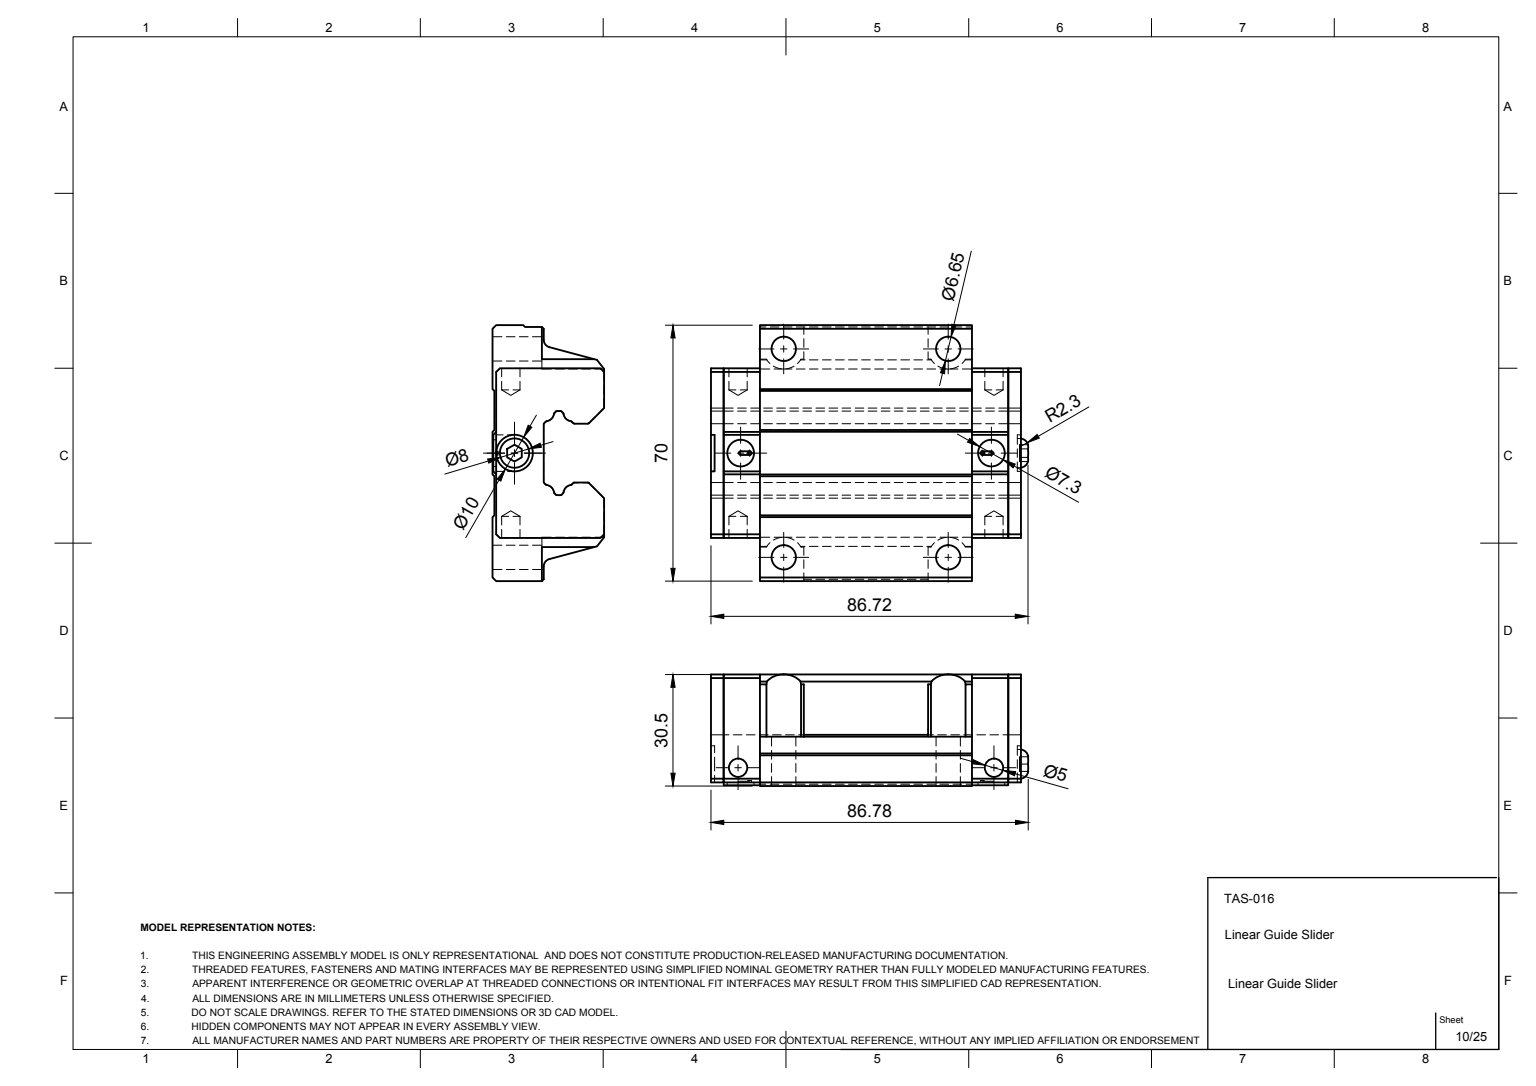
ISO-10303-21;
HEADER;
/* Generated by software containing ST-Developer
 * from STEP Tools, Inc. (www.steptools.com) 
 */

FILE_DESCRIPTION(
/* description */ ('STEP AP214'),
/* implementation_level */ '2;1');

FILE_NAME(
/* name */ 'Linear Guide Slider.step',
/* time_stamp */ '2026-11-15T14:55:55-08:00',
/* author */ (''),
/* organization */ (''),
/* preprocessor_version */ 'ST-DEVELOPER v20.2',
/* originating_system */ 'Autodesk Translation Framework v15.17.0.0',
/* authorisation */ '');

FILE_SCHEMA (('AUTOMOTIVE_DESIGN { 1 0 10303 214 3 1 1 }'));
ENDSEC;

DATA;
#10=MECHANICAL_DESIGN_GEOMETRIC_PRESENTATION_REPRESENTATION('',(#951),#57079);
#11=(
BOUNDED_CURVE()
B_SPLINE_CURVE(2,(#54195,#54196,#54197),.UNSPECIFIED.,.F.,.F.)
B_SPLINE_CURVE_WITH_KNOTS((3,3),(-1.29356557390797,0.),.UNSPECIFIED.)
CURVE()
GEOMETRIC_REPRESENTATION_ITEM()
RATIONAL_B_SPLINE_CURVE((0.954658532851732,0.77704632554749,1.))
REPRESENTATION_ITEM('')
);
#146=ELLIPSE('',#26558,6.97960018289555,5.49999999999817);
#147=ELLIPSE('',#26560,6.97960018289945,5.50000000000025);
#148=ELLIPSE('',#26561,6.97960018289465,5.49999999999756);
#149=ELLIPSE('',#26563,6.97960018289959,5.50000000000032);
#150=ELLIPSE('',#26564,6.97960018289765,5.49999999999922);
#151=ELLIPSE('',#26566,6.9796001828989,5.49999999999987);
#152=ELLIPSE('',#26887,21.2503681783598,5.50000000000001);
#153=ELLIPSE('',#26888,21.2503681783597,5.5);
#154=ELLIPSE('',#26893,21.2503681783597,5.5);
#155=ELLIPSE('',#26898,21.2503681783597,5.5);
#156=ELLIPSE('',#26900,21.2503681783597,5.49999999999999);
#157=ELLIPSE('',#26901,21.2503681783597,5.5);
#158=ELLIPSE('',#26994,21.2503681783598,5.50000000000001);
#159=ELLIPSE('',#26996,21.2503681783597,5.49999999999999);
#160=ELLIPSE('',#27001,6.97960018290351,5.50000000000224);
#161=ELLIPSE('',#27006,6.97960018290198,5.50000000000146);
#252=(
BOUNDED_SURFACE()
B_SPLINE_SURFACE(2,2,((#54133,#54134,#54135,#54136,#54137,#54138,#54139,
#54140,#54141),(#54142,#54143,#54144,#54145,#54146,#54147,#54148,#54149,
#54150),(#54151,#54152,#54153,#54154,#54155,#54156,#54157,#54158,#54159)),
 .UNSPECIFIED.,.F.,.T.,.F.)
B_SPLINE_SURFACE_WITH_KNOTS((3,3),(3,2,2,2,3),(0.,1.43998883071719),(-3.14159265358979,
-1.5707963267949,0.,1.5707963267949,3.14159265358979),.UNSPECIFIED.)
GEOMETRIC_REPRESENTATION_ITEM()
RATIONAL_B_SPLINE_SURFACE(((1.,0.707106781186548,1.,0.707106781186548,1.,
0.707106781186548,1.,0.707106781186548,1.),(0.751809411556116,0.531609533071198,
0.751809411556116,0.531609533071198,0.751809411556116,0.531609533071198,
0.751809411556116,0.531609533071198,0.751809411556116),(1.,0.707106781186548,
1.,0.707106781186548,1.,0.707106781186548,1.,0.707106781186548,1.)))
REPRESENTATION_ITEM('')
SURFACE()
);
#860=B_SPLINE_CURVE_WITH_KNOTS('',3,(#54162,#54163,#54164,#54165,#54166,
#54167,#54168,#54169,#54170,#54171),.UNSPECIFIED.,.F.,.F.,(4,2,2,2,4),(-0.991617660219933,
-0.988360888345703,-0.882558915285875,-0.776756942226048,-0.773500170351817),
 .UNSPECIFIED.);
#861=B_SPLINE_CURVE_WITH_KNOTS('',3,(#54173,#54174,#54175,#54176,#54177,
#54178,#54179,#54180,#54181,#54182),.UNSPECIFIED.,.F.,.F.,(4,2,2,2,4),(-0.991617660219933,
-0.988360888345703,-0.882558915285875,-0.776756942226048,-0.773500170351817),
 .UNSPECIFIED.);
#862=B_SPLINE_CURVE_WITH_KNOTS('',3,(#54184,#54185,#54186,#54187,#54188,
#54189,#54190,#54191,#54192,#54193),.UNSPECIFIED.,.F.,.F.,(4,2,2,2,4),(-0.991617660219934,
-0.988360888345704,-0.882558915285876,-0.776756942226048,-0.773500170351818),
 .UNSPECIFIED.);
#863=B_SPLINE_CURVE_WITH_KNOTS('',3,(#54202,#54203,#54204,#54205,#54206,
#54207,#54208,#54209,#54210,#54211),.UNSPECIFIED.,.F.,.F.,(4,2,2,2,4),(0.773500170351818,
0.776756942226048,0.882558915285876,0.988360888345703,0.991617660219934),
 .UNSPECIFIED.);
#864=B_SPLINE_CURVE_WITH_KNOTS('',3,(#54213,#54214,#54215,#54216,#54217,
#54218,#54219,#54220,#54221,#54222),.UNSPECIFIED.,.F.,.F.,(4,2,2,2,4),(0.773500170351817,
0.776756942226048,0.882558915285875,0.988360888345703,0.991617660219933),
 .UNSPECIFIED.);
#865=B_SPLINE_CURVE_WITH_KNOTS('',3,(#54223,#54224,#54225,#54226,#54227,
#54228,#54229,#54230,#54231,#54232),.UNSPECIFIED.,.F.,.F.,(4,2,2,2,4),(0.773500170351818,
0.776756942226048,0.882558915285876,0.988360888345704,0.991617660219934),
 .UNSPECIFIED.);
#889=SHAPE_REPRESENTATION_RELATIONSHIP('SRR','None',#57279,#918);
#918=ADVANCED_BREP_SHAPE_REPRESENTATION('',(#988),#57071);
#951=STYLED_ITEM('',(#57444),#988);
#988=MANIFOLD_SOLID_BREP('Body1',#24551);
#1293=FACE_BOUND('',#4751,.T.);
#1294=FACE_BOUND('',#4754,.T.);
#1295=FACE_BOUND('',#4769,.T.);
#1296=FACE_BOUND('',#4867,.T.);
#1297=FACE_BOUND('',#4880,.T.);
#1298=FACE_BOUND('',#4888,.T.);
#1299=FACE_BOUND('',#4891,.T.);
#1300=FACE_BOUND('',#4896,.T.);
#1301=FACE_BOUND('',#4944,.T.);
#1302=FACE_BOUND('',#4949,.T.);
#1303=FACE_BOUND('',#4951,.T.);
#1304=FACE_BOUND('',#4958,.T.);
#1305=FACE_BOUND('',#4959,.T.);
#1306=FACE_BOUND('',#4968,.T.);
#1307=FACE_BOUND('',#4969,.T.);
#1308=FACE_BOUND('',#4975,.T.);
#1309=FACE_BOUND('',#4981,.T.);
#1310=FACE_BOUND('',#4988,.T.);
#1311=FACE_BOUND('',#4993,.T.);
#1312=FACE_BOUND('',#5028,.T.);
#1313=FACE_BOUND('',#5040,.T.);
#1314=FACE_BOUND('',#5042,.T.);
#1788=PLANE('',#26557);
#1789=PLANE('',#26559);
#1790=PLANE('',#26562);
#1791=PLANE('',#26565);
#1792=PLANE('',#26567);
#1793=PLANE('',#26568);
#1794=PLANE('',#26569);
#1795=PLANE('',#26570);
#1796=PLANE('',#26571);
#1797=PLANE('',#26572);
#1798=PLANE('',#26573);
#1799=PLANE('',#26574);
#1800=PLANE('',#26575);
#1801=PLANE('',#26576);
#1802=PLANE('',#26577);
#1803=PLANE('',#26578);
#1804=PLANE('',#26579);
#1805=PLANE('',#26580);
#1806=PLANE('',#26581);
#1807=PLANE('',#26582);
#1808=PLANE('',#26583);
#1809=PLANE('',#26644);
#1810=PLANE('',#26645);
#1811=PLANE('',#26646);
#1812=PLANE('',#26647);
#1813=PLANE('',#26648);
#1814=PLANE('',#26649);
#1815=PLANE('',#26650);
#1816=PLANE('',#26651);
#1817=PLANE('',#26652);
#1818=PLANE('',#26653);
#1819=PLANE('',#26654);
#1820=PLANE('',#26655);
#1821=PLANE('',#26656);
#1822=PLANE('',#26657);
#1823=PLANE('',#26658);
#1824=PLANE('',#26659);
#1825=PLANE('',#26660);
#1826=PLANE('',#26681);
#1827=PLANE('',#26684);
#1828=PLANE('',#26687);
#1829=PLANE('',#26694);
#1830=PLANE('',#26697);
#1831=PLANE('',#26700);
#1832=PLANE('',#26707);
#1833=PLANE('',#26708);
#1834=PLANE('',#26709);
#1835=PLANE('',#26716);
#1836=PLANE('',#26719);
#1837=PLANE('',#26722);
#1838=PLANE('',#26729);
#1839=PLANE('',#26732);
#1840=PLANE('',#26735);
#1841=PLANE('',#26736);
#1842=PLANE('',#26737);
#1843=PLANE('',#26738);
#1844=PLANE('',#26739);
#1845=PLANE('',#26740);
#1846=PLANE('',#26741);
#1847=PLANE('',#26742);
#1848=PLANE('',#26743);
#1849=PLANE('',#26744);
#1850=PLANE('',#26745);
#1851=PLANE('',#26746);
#1852=PLANE('',#26748);
#1853=PLANE('',#26770);
#1854=PLANE('',#26771);
#1855=PLANE('',#26774);
#1856=PLANE('',#26775);
#1857=PLANE('',#26777);
#1858=PLANE('',#26778);
#1859=PLANE('',#26779);
#1860=PLANE('',#26780);
#1861=PLANE('',#26781);
#1862=PLANE('',#26782);
#1863=PLANE('',#26783);
#1864=PLANE('',#26784);
#1865=PLANE('',#26785);
#1866=PLANE('',#26786);
#1867=PLANE('',#26789);
#1868=PLANE('',#26792);
#1869=PLANE('',#26799);
#1870=PLANE('',#26802);
#1871=PLANE('',#26805);
#1872=PLANE('',#26812);
#1873=PLANE('',#26813);
#1874=PLANE('',#26814);
#1875=PLANE('',#26821);
#1876=PLANE('',#26824);
#1877=PLANE('',#26827);
#1878=PLANE('',#26834);
#1879=PLANE('',#26837);
#1880=PLANE('',#26840);
#1881=PLANE('',#26841);
#1882=PLANE('',#26842);
#1883=PLANE('',#26843);
#1884=PLANE('',#26844);
#1885=PLANE('',#26845);
#1886=PLANE('',#26851);
#1887=PLANE('',#26852);
#1888=PLANE('',#26853);
#1889=PLANE('',#26854);
#1890=PLANE('',#26858);
#1891=PLANE('',#26879);
#1892=PLANE('',#26880);
#1893=PLANE('',#26881);
#1894=PLANE('',#26882);
#1895=PLANE('',#26883);
#1896=PLANE('',#26884);
#1897=PLANE('',#26885);
#1898=PLANE('',#26886);
#1899=PLANE('',#26889);
#1900=PLANE('',#26891);
#1901=PLANE('',#26892);
#1902=PLANE('',#26894);
#1903=PLANE('',#26895);
#1904=PLANE('',#26897);
#1905=PLANE('',#26899);
#1906=PLANE('',#26902);
#1907=PLANE('',#26903);
#1908=PLANE('',#26904);
#1909=PLANE('',#26905);
#1910=PLANE('',#26906);
#1911=PLANE('',#26907);
#1912=PLANE('',#26908);
#1913=PLANE('',#26909);
#1914=PLANE('',#26910);
#1915=PLANE('',#26911);
#1916=PLANE('',#26914);
#1917=PLANE('',#26917);
#1918=PLANE('',#26924);
#1919=PLANE('',#26927);
#1920=PLANE('',#26930);
#1921=PLANE('',#26937);
#1922=PLANE('',#26938);
#1923=PLANE('',#26939);
#1924=PLANE('',#26946);
#1925=PLANE('',#26949);
#1926=PLANE('',#26952);
#1927=PLANE('',#26959);
#1928=PLANE('',#26962);
#1929=PLANE('',#26965);
#1930=PLANE('',#26966);
#1931=PLANE('',#26967);
#1932=PLANE('',#26968);
#1933=PLANE('',#26969);
#1934=PLANE('',#26970);
#1935=PLANE('',#26971);
#1936=PLANE('',#26972);
#1937=PLANE('',#26973);
#1938=PLANE('',#26974);
#1939=PLANE('',#26975);
#1940=PLANE('',#26976);
#1941=PLANE('',#26977);
#1942=PLANE('',#26978);
#1943=PLANE('',#26979);
#1944=PLANE('',#26980);
#1945=PLANE('',#26981);
#1946=PLANE('',#26982);
#1947=PLANE('',#26983);
#1948=PLANE('',#26984);
#1949=PLANE('',#26985);
#1950=PLANE('',#26986);
#1951=PLANE('',#26987);
#1952=PLANE('',#26988);
#1953=PLANE('',#26989);
#1954=PLANE('',#26990);
#1955=PLANE('',#26992);
#1956=PLANE('',#26993);
#1957=PLANE('',#26995);
#1958=PLANE('',#26997);
#1959=PLANE('',#26998);
#1960=PLANE('',#27000);
#1961=PLANE('',#27002);
#1962=PLANE('',#27003);
#1963=PLANE('',#27004);
#1964=PLANE('',#27005);
#1965=PLANE('',#27007);
#1966=PLANE('',#27028);
#1967=PLANE('',#27029);
#1968=PLANE('',#27030);
#1969=PLANE('',#27031);
#1970=PLANE('',#27032);
#1971=PLANE('',#27033);
#1972=PLANE('',#27038);
#1973=PLANE('',#27039);
#1974=PLANE('',#27040);
#1975=PLANE('',#27051);
#1976=PLANE('',#27052);
#1977=PLANE('',#27059);
#1978=PLANE('',#27060);
#1979=PLANE('',#27071);
#1980=PLANE('',#27072);
#1981=PLANE('',#27073);
#1982=PLANE('',#27084);
#1983=PLANE('',#27085);
#1984=PLANE('',#27086);
#1985=PLANE('',#27087);
#1986=PLANE('',#27088);
#1987=PLANE('',#27089);
#1988=PLANE('',#27090);
#1989=PLANE('',#27091);
#1990=PLANE('',#27092);
#1991=PLANE('',#27093);
#1992=PLANE('',#27094);
#1993=PLANE('',#27095);
#1994=PLANE('',#27096);
#1995=PLANE('',#27097);
#1996=PLANE('',#27098);
#1997=PLANE('',#27101);
#1998=PLANE('',#27102);
#2124=CONICAL_SURFACE('',#26517,2.5,1.02974425867665);
#2125=CONICAL_SURFACE('',#26518,2.5,1.02974425867665);
#2126=CONICAL_SURFACE('',#26544,2.5,1.02974425867665);
#2127=CONICAL_SURFACE('',#26545,2.5,1.02974425867665);
#3022=FACE_OUTER_BOUND('',#4690,.T.);
#3023=FACE_OUTER_BOUND('',#4691,.T.);
#3024=FACE_OUTER_BOUND('',#4692,.T.);
#3025=FACE_OUTER_BOUND('',#4693,.T.);
#3026=FACE_OUTER_BOUND('',#4694,.T.);
#3027=FACE_OUTER_BOUND('',#4695,.T.);
#3028=FACE_OUTER_BOUND('',#4696,.T.);
#3029=FACE_OUTER_BOUND('',#4697,.T.);
#3030=FACE_OUTER_BOUND('',#4698,.T.);
#3031=FACE_OUTER_BOUND('',#4699,.T.);
#3032=FACE_OUTER_BOUND('',#4700,.T.);
#3033=FACE_OUTER_BOUND('',#4701,.T.);
#3034=FACE_OUTER_BOUND('',#4702,.T.);
#3035=FACE_OUTER_BOUND('',#4703,.T.);
#3036=FACE_OUTER_BOUND('',#4704,.T.);
#3037=FACE_OUTER_BOUND('',#4705,.T.);
#3038=FACE_OUTER_BOUND('',#4706,.T.);
#3039=FACE_OUTER_BOUND('',#4707,.T.);
#3040=FACE_OUTER_BOUND('',#4708,.T.);
#3041=FACE_OUTER_BOUND('',#4709,.T.);
#3042=FACE_OUTER_BOUND('',#4710,.T.);
#3043=FACE_OUTER_BOUND('',#4711,.T.);
#3044=FACE_OUTER_BOUND('',#4712,.T.);
#3045=FACE_OUTER_BOUND('',#4713,.T.);
#3046=FACE_OUTER_BOUND('',#4714,.T.);
#3047=FACE_OUTER_BOUND('',#4715,.T.);
#3048=FACE_OUTER_BOUND('',#4716,.T.);
#3049=FACE_OUTER_BOUND('',#4717,.T.);
#3050=FACE_OUTER_BOUND('',#4718,.T.);
#3051=FACE_OUTER_BOUND('',#4719,.T.);
#3052=FACE_OUTER_BOUND('',#4720,.T.);
#3053=FACE_OUTER_BOUND('',#4721,.T.);
#3054=FACE_OUTER_BOUND('',#4722,.T.);
#3055=FACE_OUTER_BOUND('',#4723,.T.);
#3056=FACE_OUTER_BOUND('',#4724,.T.);
#3057=FACE_OUTER_BOUND('',#4725,.T.);
#3058=FACE_OUTER_BOUND('',#4726,.T.);
#3059=FACE_OUTER_BOUND('',#4727,.T.);
#3060=FACE_OUTER_BOUND('',#4728,.T.);
#3061=FACE_OUTER_BOUND('',#4729,.T.);
#3062=FACE_OUTER_BOUND('',#4730,.T.);
#3063=FACE_OUTER_BOUND('',#4731,.T.);
#3064=FACE_OUTER_BOUND('',#4732,.T.);
#3065=FACE_OUTER_BOUND('',#4733,.T.);
#3066=FACE_OUTER_BOUND('',#4734,.T.);
#3067=FACE_OUTER_BOUND('',#4735,.T.);
#3068=FACE_OUTER_BOUND('',#4736,.T.);
#3069=FACE_OUTER_BOUND('',#4737,.T.);
#3070=FACE_OUTER_BOUND('',#4738,.T.);
#3071=FACE_OUTER_BOUND('',#4739,.T.);
#3072=FACE_OUTER_BOUND('',#4740,.T.);
#3073=FACE_OUTER_BOUND('',#4741,.T.);
#3074=FACE_OUTER_BOUND('',#4742,.T.);
#3075=FACE_OUTER_BOUND('',#4743,.T.);
#3076=FACE_OUTER_BOUND('',#4744,.T.);
#3077=FACE_OUTER_BOUND('',#4745,.T.);
#3078=FACE_OUTER_BOUND('',#4746,.T.);
#3079=FACE_OUTER_BOUND('',#4747,.T.);
#3080=FACE_OUTER_BOUND('',#4748,.T.);
#3081=FACE_OUTER_BOUND('',#4749,.T.);
#3082=FACE_OUTER_BOUND('',#4750,.T.);
#3083=FACE_OUTER_BOUND('',#4752,.T.);
#3084=FACE_OUTER_BOUND('',#4753,.T.);
#3085=FACE_OUTER_BOUND('',#4755,.T.);
#3086=FACE_OUTER_BOUND('',#4756,.T.);
#3087=FACE_OUTER_BOUND('',#4757,.T.);
#3088=FACE_OUTER_BOUND('',#4758,.T.);
#3089=FACE_OUTER_BOUND('',#4759,.T.);
#3090=FACE_OUTER_BOUND('',#4760,.T.);
#3091=FACE_OUTER_BOUND('',#4761,.T.);
#3092=FACE_OUTER_BOUND('',#4762,.T.);
#3093=FACE_OUTER_BOUND('',#4763,.T.);
#3094=FACE_OUTER_BOUND('',#4764,.T.);
#3095=FACE_OUTER_BOUND('',#4765,.T.);
#3096=FACE_OUTER_BOUND('',#4766,.T.);
#3097=FACE_OUTER_BOUND('',#4767,.T.);
#3098=FACE_OUTER_BOUND('',#4768,.T.);
#3099=FACE_OUTER_BOUND('',#4770,.T.);
#3100=FACE_OUTER_BOUND('',#4771,.T.);
#3101=FACE_OUTER_BOUND('',#4772,.T.);
#3102=FACE_OUTER_BOUND('',#4773,.T.);
#3103=FACE_OUTER_BOUND('',#4774,.T.);
#3104=FACE_OUTER_BOUND('',#4775,.T.);
#3105=FACE_OUTER_BOUND('',#4776,.T.);
#3106=FACE_OUTER_BOUND('',#4777,.T.);
#3107=FACE_OUTER_BOUND('',#4778,.T.);
#3108=FACE_OUTER_BOUND('',#4779,.T.);
#3109=FACE_OUTER_BOUND('',#4780,.T.);
#3110=FACE_OUTER_BOUND('',#4781,.T.);
#3111=FACE_OUTER_BOUND('',#4782,.T.);
#3112=FACE_OUTER_BOUND('',#4783,.T.);
#3113=FACE_OUTER_BOUND('',#4784,.T.);
#3114=FACE_OUTER_BOUND('',#4785,.T.);
#3115=FACE_OUTER_BOUND('',#4786,.T.);
#3116=FACE_OUTER_BOUND('',#4787,.T.);
#3117=FACE_OUTER_BOUND('',#4788,.T.);
#3118=FACE_OUTER_BOUND('',#4789,.T.);
#3119=FACE_OUTER_BOUND('',#4790,.T.);
#3120=FACE_OUTER_BOUND('',#4791,.T.);
#3121=FACE_OUTER_BOUND('',#4792,.T.);
#3122=FACE_OUTER_BOUND('',#4793,.T.);
#3123=FACE_OUTER_BOUND('',#4794,.T.);
#3124=FACE_OUTER_BOUND('',#4795,.T.);
#3125=FACE_OUTER_BOUND('',#4796,.T.);
#3126=FACE_OUTER_BOUND('',#4797,.T.);
#3127=FACE_OUTER_BOUND('',#4798,.T.);
#3128=FACE_OUTER_BOUND('',#4799,.T.);
#3129=FACE_OUTER_BOUND('',#4800,.T.);
#3130=FACE_OUTER_BOUND('',#4801,.T.);
#3131=FACE_OUTER_BOUND('',#4802,.T.);
#3132=FACE_OUTER_BOUND('',#4803,.T.);
#3133=FACE_OUTER_BOUND('',#4804,.T.);
#3134=FACE_OUTER_BOUND('',#4805,.T.);
#3135=FACE_OUTER_BOUND('',#4806,.T.);
#3136=FACE_OUTER_BOUND('',#4807,.T.);
#3137=FACE_OUTER_BOUND('',#4808,.T.);
#3138=FACE_OUTER_BOUND('',#4809,.T.);
#3139=FACE_OUTER_BOUND('',#4810,.T.);
#3140=FACE_OUTER_BOUND('',#4811,.T.);
#3141=FACE_OUTER_BOUND('',#4812,.T.);
#3142=FACE_OUTER_BOUND('',#4813,.T.);
#3143=FACE_OUTER_BOUND('',#4814,.T.);
#3144=FACE_OUTER_BOUND('',#4815,.T.);
#3145=FACE_OUTER_BOUND('',#4816,.T.);
#3146=FACE_OUTER_BOUND('',#4817,.T.);
#3147=FACE_OUTER_BOUND('',#4818,.T.);
#3148=FACE_OUTER_BOUND('',#4819,.T.);
#3149=FACE_OUTER_BOUND('',#4820,.T.);
#3150=FACE_OUTER_BOUND('',#4821,.T.);
#3151=FACE_OUTER_BOUND('',#4822,.T.);
#3152=FACE_OUTER_BOUND('',#4823,.T.);
#3153=FACE_OUTER_BOUND('',#4824,.T.);
#3154=FACE_OUTER_BOUND('',#4825,.T.);
#3155=FACE_OUTER_BOUND('',#4826,.T.);
#3156=FACE_OUTER_BOUND('',#4827,.T.);
#3157=FACE_OUTER_BOUND('',#4828,.T.);
#3158=FACE_OUTER_BOUND('',#4829,.T.);
#3159=FACE_OUTER_BOUND('',#4830,.T.);
#3160=FACE_OUTER_BOUND('',#4831,.T.);
#3161=FACE_OUTER_BOUND('',#4832,.T.);
#3162=FACE_OUTER_BOUND('',#4833,.T.);
#3163=FACE_OUTER_BOUND('',#4834,.T.);
#3164=FACE_OUTER_BOUND('',#4835,.T.);
#3165=FACE_OUTER_BOUND('',#4836,.T.);
#3166=FACE_OUTER_BOUND('',#4837,.T.);
#3167=FACE_OUTER_BOUND('',#4838,.T.);
#3168=FACE_OUTER_BOUND('',#4839,.T.);
#3169=FACE_OUTER_BOUND('',#4840,.T.);
#3170=FACE_OUTER_BOUND('',#4841,.T.);
#3171=FACE_OUTER_BOUND('',#4842,.T.);
#3172=FACE_OUTER_BOUND('',#4843,.T.);
#3173=FACE_OUTER_BOUND('',#4844,.T.);
#3174=FACE_OUTER_BOUND('',#4845,.T.);
#3175=FACE_OUTER_BOUND('',#4846,.T.);
#3176=FACE_OUTER_BOUND('',#4847,.T.);
#3177=FACE_OUTER_BOUND('',#4848,.T.);
#3178=FACE_OUTER_BOUND('',#4849,.T.);
#3179=FACE_OUTER_BOUND('',#4850,.T.);
#3180=FACE_OUTER_BOUND('',#4851,.T.);
#3181=FACE_OUTER_BOUND('',#4852,.T.);
#3182=FACE_OUTER_BOUND('',#4853,.T.);
#3183=FACE_OUTER_BOUND('',#4854,.T.);
#3184=FACE_OUTER_BOUND('',#4855,.T.);
#3185=FACE_OUTER_BOUND('',#4856,.T.);
#3186=FACE_OUTER_BOUND('',#4857,.T.);
#3187=FACE_OUTER_BOUND('',#4858,.T.);
#3188=FACE_OUTER_BOUND('',#4859,.T.);
#3189=FACE_OUTER_BOUND('',#4860,.T.);
#3190=FACE_OUTER_BOUND('',#4861,.T.);
#3191=FACE_OUTER_BOUND('',#4862,.T.);
#3192=FACE_OUTER_BOUND('',#4863,.T.);
#3193=FACE_OUTER_BOUND('',#4864,.T.);
#3194=FACE_OUTER_BOUND('',#4865,.T.);
#3195=FACE_OUTER_BOUND('',#4866,.T.);
#3196=FACE_OUTER_BOUND('',#4868,.T.);
#3197=FACE_OUTER_BOUND('',#4869,.T.);
#3198=FACE_OUTER_BOUND('',#4870,.T.);
#3199=FACE_OUTER_BOUND('',#4871,.T.);
#3200=FACE_OUTER_BOUND('',#4872,.T.);
#3201=FACE_OUTER_BOUND('',#4873,.T.);
#3202=FACE_OUTER_BOUND('',#4874,.T.);
#3203=FACE_OUTER_BOUND('',#4875,.T.);
#3204=FACE_OUTER_BOUND('',#4876,.T.);
#3205=FACE_OUTER_BOUND('',#4877,.T.);
#3206=FACE_OUTER_BOUND('',#4878,.T.);
#3207=FACE_OUTER_BOUND('',#4879,.T.);
#3208=FACE_OUTER_BOUND('',#4881,.T.);
#3209=FACE_OUTER_BOUND('',#4882,.T.);
#3210=FACE_OUTER_BOUND('',#4883,.T.);
#3211=FACE_OUTER_BOUND('',#4884,.T.);
#3212=FACE_OUTER_BOUND('',#4885,.T.);
#3213=FACE_OUTER_BOUND('',#4886,.T.);
#3214=FACE_OUTER_BOUND('',#4887,.T.);
#3215=FACE_OUTER_BOUND('',#4889,.T.);
#3216=FACE_OUTER_BOUND('',#4890,.T.);
#3217=FACE_OUTER_BOUND('',#4892,.T.);
#3218=FACE_OUTER_BOUND('',#4893,.T.);
#3219=FACE_OUTER_BOUND('',#4894,.T.);
#3220=FACE_OUTER_BOUND('',#4895,.T.);
#3221=FACE_OUTER_BOUND('',#4897,.T.);
#3222=FACE_OUTER_BOUND('',#4898,.T.);
#3223=FACE_OUTER_BOUND('',#4899,.T.);
#3224=FACE_OUTER_BOUND('',#4900,.T.);
#3225=FACE_OUTER_BOUND('',#4901,.T.);
#3226=FACE_OUTER_BOUND('',#4902,.T.);
#3227=FACE_OUTER_BOUND('',#4903,.T.);
#3228=FACE_OUTER_BOUND('',#4904,.T.);
#3229=FACE_OUTER_BOUND('',#4905,.T.);
#3230=FACE_OUTER_BOUND('',#4906,.T.);
#3231=FACE_OUTER_BOUND('',#4907,.T.);
#3232=FACE_OUTER_BOUND('',#4908,.T.);
#3233=FACE_OUTER_BOUND('',#4909,.T.);
#3234=FACE_OUTER_BOUND('',#4910,.T.);
#3235=FACE_OUTER_BOUND('',#4911,.T.);
#3236=FACE_OUTER_BOUND('',#4912,.T.);
#3237=FACE_OUTER_BOUND('',#4913,.T.);
#3238=FACE_OUTER_BOUND('',#4914,.T.);
#3239=FACE_OUTER_BOUND('',#4915,.T.);
#3240=FACE_OUTER_BOUND('',#4916,.T.);
#3241=FACE_OUTER_BOUND('',#4917,.T.);
#3242=FACE_OUTER_BOUND('',#4918,.T.);
#3243=FACE_OUTER_BOUND('',#4919,.T.);
#3244=FACE_OUTER_BOUND('',#4920,.T.);
#3245=FACE_OUTER_BOUND('',#4921,.T.);
#3246=FACE_OUTER_BOUND('',#4922,.T.);
#3247=FACE_OUTER_BOUND('',#4923,.T.);
#3248=FACE_OUTER_BOUND('',#4924,.T.);
#3249=FACE_OUTER_BOUND('',#4925,.T.);
#3250=FACE_OUTER_BOUND('',#4926,.T.);
#3251=FACE_OUTER_BOUND('',#4927,.T.);
#3252=FACE_OUTER_BOUND('',#4928,.T.);
#3253=FACE_OUTER_BOUND('',#4929,.T.);
#3254=FACE_OUTER_BOUND('',#4930,.T.);
#3255=FACE_OUTER_BOUND('',#4931,.T.);
#3256=FACE_OUTER_BOUND('',#4932,.T.);
#3257=FACE_OUTER_BOUND('',#4933,.T.);
#3258=FACE_OUTER_BOUND('',#4934,.T.);
#3259=FACE_OUTER_BOUND('',#4935,.T.);
#3260=FACE_OUTER_BOUND('',#4936,.T.);
#3261=FACE_OUTER_BOUND('',#4937,.T.);
#3262=FACE_OUTER_BOUND('',#4938,.T.);
#3263=FACE_OUTER_BOUND('',#4939,.T.);
#3264=FACE_OUTER_BOUND('',#4940,.T.);
#3265=FACE_OUTER_BOUND('',#4941,.T.);
#3266=FACE_OUTER_BOUND('',#4942,.T.);
#3267=FACE_OUTER_BOUND('',#4943,.T.);
#3268=FACE_OUTER_BOUND('',#4945,.T.);
#3269=FACE_OUTER_BOUND('',#4946,.T.);
#3270=FACE_OUTER_BOUND('',#4947,.T.);
#3271=FACE_OUTER_BOUND('',#4948,.T.);
#3272=FACE_OUTER_BOUND('',#4950,.T.);
#3273=FACE_OUTER_BOUND('',#4952,.T.);
#3274=FACE_OUTER_BOUND('',#4953,.T.);
#3275=FACE_OUTER_BOUND('',#4954,.T.);
#3276=FACE_OUTER_BOUND('',#4955,.T.);
#3277=FACE_OUTER_BOUND('',#4956,.T.);
#3278=FACE_OUTER_BOUND('',#4957,.T.);
#3279=FACE_OUTER_BOUND('',#4960,.T.);
#3280=FACE_OUTER_BOUND('',#4961,.T.);
#3281=FACE_OUTER_BOUND('',#4962,.T.);
#3282=FACE_OUTER_BOUND('',#4963,.T.);
#3283=FACE_OUTER_BOUND('',#4964,.T.);
#3284=FACE_OUTER_BOUND('',#4965,.T.);
#3285=FACE_OUTER_BOUND('',#4966,.T.);
#3286=FACE_OUTER_BOUND('',#4967,.T.);
#3287=FACE_OUTER_BOUND('',#4970,.T.);
#3288=FACE_OUTER_BOUND('',#4971,.T.);
#3289=FACE_OUTER_BOUND('',#4972,.T.);
#3290=FACE_OUTER_BOUND('',#4973,.T.);
#3291=FACE_OUTER_BOUND('',#4974,.T.);
#3292=FACE_OUTER_BOUND('',#4976,.T.);
#3293=FACE_OUTER_BOUND('',#4977,.T.);
#3294=FACE_OUTER_BOUND('',#4978,.T.);
#3295=FACE_OUTER_BOUND('',#4979,.T.);
#3296=FACE_OUTER_BOUND('',#4980,.T.);
#3297=FACE_OUTER_BOUND('',#4982,.T.);
#3298=FACE_OUTER_BOUND('',#4983,.T.);
#3299=FACE_OUTER_BOUND('',#4984,.T.);
#3300=FACE_OUTER_BOUND('',#4985,.T.);
#3301=FACE_OUTER_BOUND('',#4986,.T.);
#3302=FACE_OUTER_BOUND('',#4987,.T.);
#3303=FACE_OUTER_BOUND('',#4989,.T.);
#3304=FACE_OUTER_BOUND('',#4990,.T.);
#3305=FACE_OUTER_BOUND('',#4991,.T.);
#3306=FACE_OUTER_BOUND('',#4992,.T.);
#3307=FACE_OUTER_BOUND('',#4994,.T.);
#3308=FACE_OUTER_BOUND('',#4995,.T.);
#3309=FACE_OUTER_BOUND('',#4996,.T.);
#3310=FACE_OUTER_BOUND('',#4997,.T.);
#3311=FACE_OUTER_BOUND('',#4998,.T.);
#3312=FACE_OUTER_BOUND('',#4999,.T.);
#3313=FACE_OUTER_BOUND('',#5000,.T.);
#3314=FACE_OUTER_BOUND('',#5001,.T.);
#3315=FACE_OUTER_BOUND('',#5002,.T.);
#3316=FACE_OUTER_BOUND('',#5003,.T.);
#3317=FACE_OUTER_BOUND('',#5004,.T.);
#3318=FACE_OUTER_BOUND('',#5005,.T.);
#3319=FACE_OUTER_BOUND('',#5006,.T.);
#3320=FACE_OUTER_BOUND('',#5007,.T.);
#3321=FACE_OUTER_BOUND('',#5008,.T.);
#3322=FACE_OUTER_BOUND('',#5009,.T.);
#3323=FACE_OUTER_BOUND('',#5010,.T.);
#3324=FACE_OUTER_BOUND('',#5011,.T.);
#3325=FACE_OUTER_BOUND('',#5012,.T.);
#3326=FACE_OUTER_BOUND('',#5013,.T.);
#3327=FACE_OUTER_BOUND('',#5014,.T.);
#3328=FACE_OUTER_BOUND('',#5015,.T.);
#3329=FACE_OUTER_BOUND('',#5016,.T.);
#3330=FACE_OUTER_BOUND('',#5017,.T.);
#3331=FACE_OUTER_BOUND('',#5018,.T.);
#3332=FACE_OUTER_BOUND('',#5019,.T.);
#3333=FACE_OUTER_BOUND('',#5020,.T.);
#3334=FACE_OUTER_BOUND('',#5021,.T.);
#3335=FACE_OUTER_BOUND('',#5022,.T.);
#3336=FACE_OUTER_BOUND('',#5023,.T.);
#3337=FACE_OUTER_BOUND('',#5024,.T.);
#3338=FACE_OUTER_BOUND('',#5025,.T.);
#3339=FACE_OUTER_BOUND('',#5026,.T.);
#3340=FACE_OUTER_BOUND('',#5027,.T.);
#3341=FACE_OUTER_BOUND('',#5029,.T.);
#3342=FACE_OUTER_BOUND('',#5030,.T.);
#3343=FACE_OUTER_BOUND('',#5031,.T.);
#3344=FACE_OUTER_BOUND('',#5032,.T.);
#3345=FACE_OUTER_BOUND('',#5033,.T.);
#3346=FACE_OUTER_BOUND('',#5034,.T.);
#3347=FACE_OUTER_BOUND('',#5035,.T.);
#3348=FACE_OUTER_BOUND('',#5036,.T.);
#3349=FACE_OUTER_BOUND('',#5037,.T.);
#3350=FACE_OUTER_BOUND('',#5038,.T.);
#3351=FACE_OUTER_BOUND('',#5039,.T.);
#3352=FACE_OUTER_BOUND('',#5041,.T.);
#3353=FACE_OUTER_BOUND('',#5043,.T.);
#3354=FACE_OUTER_BOUND('',#5044,.T.);
#3355=FACE_OUTER_BOUND('',#5045,.T.);
#3356=FACE_OUTER_BOUND('',#5046,.T.);
#3357=FACE_OUTER_BOUND('',#5047,.T.);
#3358=FACE_OUTER_BOUND('',#5048,.T.);
#3359=FACE_OUTER_BOUND('',#5049,.T.);
#3360=FACE_OUTER_BOUND('',#5050,.T.);
#4690=EDGE_LOOP('',(#20092,#20093,#20094,#20095));
#4691=EDGE_LOOP('',(#20096,#20097,#20098,#20099));
#4692=EDGE_LOOP('',(#20100,#20101,#20102,#20103));
#4693=EDGE_LOOP('',(#20104,#20105,#20106));
#4694=EDGE_LOOP('',(#20107,#20108,#20109));
#4695=EDGE_LOOP('',(#20110,#20111,#20112,#20113));
#4696=EDGE_LOOP('',(#20114,#20115,#20116,#20117));
#4697=EDGE_LOOP('',(#20118,#20119,#20120,#20121));
#4698=EDGE_LOOP('',(#20122,#20123,#20124,#20125));
#4699=EDGE_LOOP('',(#20126,#20127,#20128,#20129));
#4700=EDGE_LOOP('',(#20130,#20131,#20132,#20133));
#4701=EDGE_LOOP('',(#20134,#20135,#20136,#20137));
#4702=EDGE_LOOP('',(#20138,#20139,#20140,#20141,#20142,#20143,#20144));
#4703=EDGE_LOOP('',(#20145,#20146,#20147));
#4704=EDGE_LOOP('',(#20148,#20149,#20150));
#4705=EDGE_LOOP('',(#20151,#20152,#20153,#20154,#20155,#20156,#20157));
#4706=EDGE_LOOP('',(#20158,#20159,#20160,#20161,#20162,#20163,#20164,#20165,
#20166,#20167));
#4707=EDGE_LOOP('',(#20168,#20169,#20170,#20171,#20172));
#4708=EDGE_LOOP('',(#20173,#20174,#20175,#20176));
#4709=EDGE_LOOP('',(#20177,#20178,#20179,#20180));
#4710=EDGE_LOOP('',(#20181,#20182,#20183,#20184));
#4711=EDGE_LOOP('',(#20185,#20186,#20187,#20188));
#4712=EDGE_LOOP('',(#20189,#20190,#20191,#20192));
#4713=EDGE_LOOP('',(#20193,#20194,#20195,#20196));
#4714=EDGE_LOOP('',(#20197,#20198,#20199,#20200));
#4715=EDGE_LOOP('',(#20201,#20202,#20203,#20204));
#4716=EDGE_LOOP('',(#20205,#20206,#20207,#20208));
#4717=EDGE_LOOP('',(#20209,#20210,#20211,#20212));
#4718=EDGE_LOOP('',(#20213,#20214,#20215,#20216));
#4719=EDGE_LOOP('',(#20217,#20218,#20219,#20220));
#4720=EDGE_LOOP('',(#20221,#20222,#20223,#20224));
#4721=EDGE_LOOP('',(#20225,#20226,#20227,#20228));
#4722=EDGE_LOOP('',(#20229,#20230,#20231,#20232));
#4723=EDGE_LOOP('',(#20233,#20234,#20235,#20236));
#4724=EDGE_LOOP('',(#20237,#20238,#20239,#20240));
#4725=EDGE_LOOP('',(#20241,#20242,#20243,#20244));
#4726=EDGE_LOOP('',(#20245,#20246,#20247,#20248));
#4727=EDGE_LOOP('',(#20249,#20250,#20251,#20252));
#4728=EDGE_LOOP('',(#20253,#20254,#20255,#20256));
#4729=EDGE_LOOP('',(#20257,#20258,#20259,#20260));
#4730=EDGE_LOOP('',(#20261,#20262,#20263,#20264));
#4731=EDGE_LOOP('',(#20265,#20266,#20267,#20268));
#4732=EDGE_LOOP('',(#20269,#20270,#20271,#20272));
#4733=EDGE_LOOP('',(#20273,#20274,#20275,#20276));
#4734=EDGE_LOOP('',(#20277,#20278,#20279,#20280));
#4735=EDGE_LOOP('',(#20281,#20282,#20283,#20284));
#4736=EDGE_LOOP('',(#20285,#20286,#20287,#20288));
#4737=EDGE_LOOP('',(#20289,#20290,#20291,#20292));
#4738=EDGE_LOOP('',(#20293,#20294,#20295,#20296));
#4739=EDGE_LOOP('',(#20297,#20298,#20299,#20300));
#4740=EDGE_LOOP('',(#20301,#20302,#20303,#20304));
#4741=EDGE_LOOP('',(#20305,#20306,#20307,#20308));
#4742=EDGE_LOOP('',(#20309,#20310,#20311,#20312));
#4743=EDGE_LOOP('',(#20313,#20314,#20315,#20316));
#4744=EDGE_LOOP('',(#20317,#20318,#20319,#20320));
#4745=EDGE_LOOP('',(#20321,#20322,#20323,#20324));
#4746=EDGE_LOOP('',(#20325,#20326,#20327,#20328));
#4747=EDGE_LOOP('',(#20329,#20330,#20331,#20332));
#4748=EDGE_LOOP('',(#20333,#20334,#20335,#20336));
#4749=EDGE_LOOP('',(#20337,#20338,#20339,#20340));
#4750=EDGE_LOOP('',(#20341));
#4751=EDGE_LOOP('',(#20342));
#4752=EDGE_LOOP('',(#20343,#20344,#20345,#20346));
#4753=EDGE_LOOP('',(#20347,#20348,#20349,#20350,#20351,#20352,#20353,#20354,
#20355,#20356,#20357,#20358,#20359,#20360,#20361,#20362,#20363,#20364,#20365,
#20366,#20367,#20368,#20369,#20370,#20371,#20372,#20373,#20374,#20375,#20376,
#20377,#20378,#20379,#20380,#20381,#20382,#20383,#20384,#20385,#20386,#20387,
#20388,#20389,#20390));
#4754=EDGE_LOOP('',(#20391));
#4755=EDGE_LOOP('',(#20392,#20393,#20394,#20395));
#4756=EDGE_LOOP('',(#20396,#20397,#20398,#20399));
#4757=EDGE_LOOP('',(#20400,#20401,#20402,#20403));
#4758=EDGE_LOOP('',(#20404,#20405,#20406,#20407));
#4759=EDGE_LOOP('',(#20408,#20409,#20410,#20411));
#4760=EDGE_LOOP('',(#20412,#20413,#20414,#20415));
#4761=EDGE_LOOP('',(#20416,#20417,#20418,#20419));
#4762=EDGE_LOOP('',(#20420,#20421,#20422,#20423));
#4763=EDGE_LOOP('',(#20424,#20425,#20426,#20427));
#4764=EDGE_LOOP('',(#20428,#20429,#20430,#20431));
#4765=EDGE_LOOP('',(#20432,#20433,#20434,#20435));
#4766=EDGE_LOOP('',(#20436,#20437,#20438,#20439));
#4767=EDGE_LOOP('',(#20440,#20441,#20442,#20443,#20444,#20445));
#4768=EDGE_LOOP('',(#20446,#20447,#20448,#20449,#20450,#20451,#20452,#20453,
#20454,#20455,#20456,#20457,#20458,#20459,#20460,#20461,#20462,#20463,#20464,
#20465,#20466,#20467,#20468,#20469,#20470,#20471,#20472,#20473,#20474,#20475,
#20476,#20477,#20478,#20479,#20480,#20481,#20482,#20483,#20484,#20485,#20486,
#20487,#20488,#20489));
#4769=EDGE_LOOP('',(#20490,#20491,#20492,#20493,#20494,#20495,#20496,#20497,
#20498,#20499,#20500,#20501,#20502,#20503,#20504,#20505,#20506,#20507,#20508,
#20509,#20510,#20511,#20512,#20513,#20514,#20515,#20516,#20517,#20518,#20519,
#20520,#20521,#20522,#20523,#20524,#20525,#20526,#20527,#20528,#20529,#20530,
#20531,#20532,#20533));
#4770=EDGE_LOOP('',(#20534,#20535,#20536,#20537));
#4771=EDGE_LOOP('',(#20538,#20539,#20540,#20541));
#4772=EDGE_LOOP('',(#20542,#20543,#20544,#20545));
#4773=EDGE_LOOP('',(#20546,#20547,#20548,#20549));
#4774=EDGE_LOOP('',(#20550,#20551,#20552,#20553));
#4775=EDGE_LOOP('',(#20554,#20555,#20556,#20557));
#4776=EDGE_LOOP('',(#20558,#20559,#20560,#20561));
#4777=EDGE_LOOP('',(#20562,#20563,#20564,#20565));
#4778=EDGE_LOOP('',(#20566,#20567,#20568,#20569));
#4779=EDGE_LOOP('',(#20570,#20571,#20572,#20573));
#4780=EDGE_LOOP('',(#20574,#20575,#20576,#20577));
#4781=EDGE_LOOP('',(#20578,#20579,#20580,#20581));
#4782=EDGE_LOOP('',(#20582,#20583,#20584,#20585));
#4783=EDGE_LOOP('',(#20586,#20587,#20588,#20589));
#4784=EDGE_LOOP('',(#20590,#20591,#20592,#20593));
#4785=EDGE_LOOP('',(#20594,#20595,#20596,#20597));
#4786=EDGE_LOOP('',(#20598,#20599,#20600,#20601));
#4787=EDGE_LOOP('',(#20602,#20603,#20604,#20605));
#4788=EDGE_LOOP('',(#20606,#20607,#20608,#20609));
#4789=EDGE_LOOP('',(#20610,#20611,#20612,#20613));
#4790=EDGE_LOOP('',(#20614,#20615,#20616,#20617));
#4791=EDGE_LOOP('',(#20618,#20619,#20620,#20621));
#4792=EDGE_LOOP('',(#20622,#20623,#20624,#20625));
#4793=EDGE_LOOP('',(#20626,#20627,#20628,#20629));
#4794=EDGE_LOOP('',(#20630,#20631,#20632,#20633));
#4795=EDGE_LOOP('',(#20634,#20635,#20636,#20637));
#4796=EDGE_LOOP('',(#20638,#20639,#20640,#20641));
#4797=EDGE_LOOP('',(#20642,#20643,#20644,#20645));
#4798=EDGE_LOOP('',(#20646,#20647,#20648,#20649));
#4799=EDGE_LOOP('',(#20650,#20651,#20652,#20653));
#4800=EDGE_LOOP('',(#20654,#20655,#20656,#20657));
#4801=EDGE_LOOP('',(#20658,#20659,#20660,#20661));
#4802=EDGE_LOOP('',(#20662,#20663,#20664,#20665));
#4803=EDGE_LOOP('',(#20666,#20667,#20668,#20669));
#4804=EDGE_LOOP('',(#20670,#20671,#20672,#20673));
#4805=EDGE_LOOP('',(#20674,#20675,#20676,#20677));
#4806=EDGE_LOOP('',(#20678,#20679,#20680,#20681));
#4807=EDGE_LOOP('',(#20682,#20683,#20684,#20685));
#4808=EDGE_LOOP('',(#20686,#20687,#20688,#20689));
#4809=EDGE_LOOP('',(#20690,#20691,#20692,#20693));
#4810=EDGE_LOOP('',(#20694,#20695,#20696,#20697));
#4811=EDGE_LOOP('',(#20698,#20699,#20700,#20701));
#4812=EDGE_LOOP('',(#20702,#20703,#20704,#20705));
#4813=EDGE_LOOP('',(#20706,#20707,#20708,#20709));
#4814=EDGE_LOOP('',(#20710));
#4815=EDGE_LOOP('',(#20711,#20712,#20713,#20714));
#4816=EDGE_LOOP('',(#20715,#20716,#20717,#20718,#20719,#20720,#20721,#20722,
#20723,#20724,#20725,#20726,#20727,#20728,#20729,#20730,#20731,#20732,#20733,
#20734,#20735,#20736,#20737,#20738,#20739,#20740,#20741,#20742,#20743,#20744,
#20745,#20746,#20747,#20748,#20749,#20750,#20751,#20752,#20753,#20754,#20755,
#20756,#20757,#20758,#20759,#20760,#20761,#20762));
#4817=EDGE_LOOP('',(#20763,#20764,#20765,#20766));
#4818=EDGE_LOOP('',(#20767,#20768,#20769,#20770));
#4819=EDGE_LOOP('',(#20771,#20772,#20773,#20774));
#4820=EDGE_LOOP('',(#20775));
#4821=EDGE_LOOP('',(#20776,#20777,#20778,#20779));
#4822=EDGE_LOOP('',(#20780,#20781,#20782,#20783));
#4823=EDGE_LOOP('',(#20784,#20785,#20786,#20787));
#4824=EDGE_LOOP('',(#20788,#20789,#20790,#20791));
#4825=EDGE_LOOP('',(#20792,#20793,#20794,#20795));
#4826=EDGE_LOOP('',(#20796,#20797,#20798,#20799,#20800,#20801,#20802,#20803));
#4827=EDGE_LOOP('',(#20804,#20805,#20806,#20807));
#4828=EDGE_LOOP('',(#20808,#20809,#20810,#20811));
#4829=EDGE_LOOP('',(#20812,#20813,#20814,#20815));
#4830=EDGE_LOOP('',(#20816,#20817,#20818,#20819));
#4831=EDGE_LOOP('',(#20820,#20821,#20822,#20823));
#4832=EDGE_LOOP('',(#20824,#20825,#20826,#20827));
#4833=EDGE_LOOP('',(#20828,#20829,#20830,#20831));
#4834=EDGE_LOOP('',(#20832,#20833,#20834,#20835));
#4835=EDGE_LOOP('',(#20836,#20837,#20838,#20839));
#4836=EDGE_LOOP('',(#20840,#20841,#20842,#20843));
#4837=EDGE_LOOP('',(#20844,#20845,#20846,#20847));
#4838=EDGE_LOOP('',(#20848,#20849,#20850,#20851));
#4839=EDGE_LOOP('',(#20852,#20853,#20854,#20855));
#4840=EDGE_LOOP('',(#20856,#20857,#20858,#20859));
#4841=EDGE_LOOP('',(#20860,#20861,#20862,#20863));
#4842=EDGE_LOOP('',(#20864,#20865,#20866,#20867));
#4843=EDGE_LOOP('',(#20868,#20869,#20870,#20871));
#4844=EDGE_LOOP('',(#20872,#20873,#20874,#20875));
#4845=EDGE_LOOP('',(#20876,#20877,#20878,#20879));
#4846=EDGE_LOOP('',(#20880,#20881,#20882,#20883));
#4847=EDGE_LOOP('',(#20884,#20885,#20886,#20887));
#4848=EDGE_LOOP('',(#20888,#20889,#20890,#20891));
#4849=EDGE_LOOP('',(#20892,#20893,#20894,#20895));
#4850=EDGE_LOOP('',(#20896,#20897,#20898,#20899));
#4851=EDGE_LOOP('',(#20900,#20901,#20902,#20903));
#4852=EDGE_LOOP('',(#20904,#20905,#20906,#20907));
#4853=EDGE_LOOP('',(#20908,#20909,#20910,#20911));
#4854=EDGE_LOOP('',(#20912,#20913,#20914,#20915));
#4855=EDGE_LOOP('',(#20916,#20917,#20918,#20919));
#4856=EDGE_LOOP('',(#20920,#20921,#20922,#20923));
#4857=EDGE_LOOP('',(#20924,#20925,#20926,#20927));
#4858=EDGE_LOOP('',(#20928,#20929,#20930,#20931));
#4859=EDGE_LOOP('',(#20932,#20933,#20934,#20935));
#4860=EDGE_LOOP('',(#20936,#20937,#20938,#20939));
#4861=EDGE_LOOP('',(#20940,#20941,#20942,#20943));
#4862=EDGE_LOOP('',(#20944,#20945,#20946,#20947));
#4863=EDGE_LOOP('',(#20948,#20949,#20950,#20951));
#4864=EDGE_LOOP('',(#20952,#20953,#20954,#20955));
#4865=EDGE_LOOP('',(#20956,#20957,#20958,#20959));
#4866=EDGE_LOOP('',(#20960));
#4867=EDGE_LOOP('',(#20961,#20962,#20963,#20964));
#4868=EDGE_LOOP('',(#20965,#20966,#20967,#20968));
#4869=EDGE_LOOP('',(#20969,#20970,#20971,#20972));
#4870=EDGE_LOOP('',(#20973,#20974,#20975,#20976));
#4871=EDGE_LOOP('',(#20977,#20978,#20979,#20980));
#4872=EDGE_LOOP('',(#20981,#20982,#20983,#20984));
#4873=EDGE_LOOP('',(#20985,#20986,#20987,#20988));
#4874=EDGE_LOOP('',(#20989,#20990,#20991,#20992,#20993,#20994));
#4875=EDGE_LOOP('',(#20995,#20996,#20997,#20998));
#4876=EDGE_LOOP('',(#20999,#21000,#21001,#21002));
#4877=EDGE_LOOP('',(#21003,#21004,#21005,#21006,#21007,#21008));
#4878=EDGE_LOOP('',(#21009,#21010,#21011,#21012));
#4879=EDGE_LOOP('',(#21013,#21014,#21015,#21016,#21017,#21018,#21019,#21020,
#21021,#21022,#21023,#21024,#21025,#21026,#21027,#21028,#21029,#21030,#21031,
#21032,#21033,#21034,#21035,#21036,#21037,#21038,#21039,#21040,#21041,#21042,
#21043,#21044,#21045,#21046,#21047,#21048,#21049,#21050,#21051,#21052,#21053,
#21054,#21055,#21056));
#4880=EDGE_LOOP('',(#21057,#21058,#21059,#21060,#21061,#21062,#21063,#21064,
#21065,#21066,#21067,#21068,#21069,#21070,#21071,#21072,#21073,#21074,#21075,
#21076,#21077,#21078,#21079,#21080,#21081,#21082,#21083,#21084,#21085,#21086,
#21087,#21088,#21089,#21090,#21091,#21092,#21093,#21094,#21095,#21096,#21097,
#21098,#21099,#21100));
#4881=EDGE_LOOP('',(#21101,#21102,#21103,#21104));
#4882=EDGE_LOOP('',(#21105,#21106,#21107,#21108));
#4883=EDGE_LOOP('',(#21109,#21110,#21111,#21112,#21113,#21114));
#4884=EDGE_LOOP('',(#21115,#21116,#21117,#21118));
#4885=EDGE_LOOP('',(#21119,#21120,#21121,#21122,#21123,#21124));
#4886=EDGE_LOOP('',(#21125,#21126,#21127,#21128));
#4887=EDGE_LOOP('',(#21129));
#4888=EDGE_LOOP('',(#21130,#21131,#21132,#21133));
#4889=EDGE_LOOP('',(#21134,#21135,#21136,#21137,#21138,#21139,#21140,#21141));
#4890=EDGE_LOOP('',(#21142,#21143,#21144,#21145,#21146,#21147));
#4891=EDGE_LOOP('',(#21148));
#4892=EDGE_LOOP('',(#21149,#21150,#21151,#21152));
#4893=EDGE_LOOP('',(#21153,#21154,#21155,#21156));
#4894=EDGE_LOOP('',(#21157,#21158,#21159,#21160));
#4895=EDGE_LOOP('',(#21161,#21162,#21163,#21164,#21165,#21166));
#4896=EDGE_LOOP('',(#21167));
#4897=EDGE_LOOP('',(#21168,#21169,#21170,#21171));
#4898=EDGE_LOOP('',(#21172,#21173,#21174,#21175,#21176,#21177,#21178,#21179));
#4899=EDGE_LOOP('',(#21180,#21181,#21182,#21183));
#4900=EDGE_LOOP('',(#21184,#21185,#21186,#21187));
#4901=EDGE_LOOP('',(#21188,#21189,#21190,#21191));
#4902=EDGE_LOOP('',(#21192,#21193,#21194,#21195));
#4903=EDGE_LOOP('',(#21196,#21197,#21198,#21199));
#4904=EDGE_LOOP('',(#21200,#21201,#21202,#21203));
#4905=EDGE_LOOP('',(#21204,#21205,#21206,#21207));
#4906=EDGE_LOOP('',(#21208,#21209,#21210,#21211));
#4907=EDGE_LOOP('',(#21212,#21213,#21214,#21215));
#4908=EDGE_LOOP('',(#21216,#21217,#21218,#21219));
#4909=EDGE_LOOP('',(#21220,#21221,#21222,#21223));
#4910=EDGE_LOOP('',(#21224,#21225,#21226,#21227));
#4911=EDGE_LOOP('',(#21228,#21229,#21230,#21231));
#4912=EDGE_LOOP('',(#21232,#21233,#21234,#21235));
#4913=EDGE_LOOP('',(#21236,#21237,#21238,#21239));
#4914=EDGE_LOOP('',(#21240,#21241,#21242,#21243));
#4915=EDGE_LOOP('',(#21244,#21245,#21246,#21247));
#4916=EDGE_LOOP('',(#21248,#21249,#21250,#21251));
#4917=EDGE_LOOP('',(#21252,#21253,#21254,#21255));
#4918=EDGE_LOOP('',(#21256,#21257,#21258,#21259));
#4919=EDGE_LOOP('',(#21260,#21261,#21262,#21263));
#4920=EDGE_LOOP('',(#21264,#21265,#21266,#21267));
#4921=EDGE_LOOP('',(#21268,#21269,#21270,#21271));
#4922=EDGE_LOOP('',(#21272,#21273,#21274,#21275));
#4923=EDGE_LOOP('',(#21276,#21277,#21278,#21279));
#4924=EDGE_LOOP('',(#21280,#21281,#21282,#21283));
#4925=EDGE_LOOP('',(#21284,#21285,#21286,#21287));
#4926=EDGE_LOOP('',(#21288,#21289,#21290,#21291));
#4927=EDGE_LOOP('',(#21292,#21293,#21294,#21295));
#4928=EDGE_LOOP('',(#21296,#21297,#21298,#21299));
#4929=EDGE_LOOP('',(#21300,#21301,#21302,#21303));
#4930=EDGE_LOOP('',(#21304,#21305,#21306,#21307));
#4931=EDGE_LOOP('',(#21308,#21309,#21310,#21311));
#4932=EDGE_LOOP('',(#21312,#21313,#21314,#21315));
#4933=EDGE_LOOP('',(#21316,#21317,#21318,#21319));
#4934=EDGE_LOOP('',(#21320,#21321,#21322,#21323));
#4935=EDGE_LOOP('',(#21324,#21325,#21326,#21327));
#4936=EDGE_LOOP('',(#21328,#21329,#21330,#21331));
#4937=EDGE_LOOP('',(#21332,#21333,#21334,#21335));
#4938=EDGE_LOOP('',(#21336,#21337,#21338,#21339));
#4939=EDGE_LOOP('',(#21340,#21341,#21342,#21343));
#4940=EDGE_LOOP('',(#21344,#21345,#21346,#21347));
#4941=EDGE_LOOP('',(#21348,#21349,#21350,#21351));
#4942=EDGE_LOOP('',(#21352,#21353,#21354,#21355));
#4943=EDGE_LOOP('',(#21356,#21357,#21358,#21359));
#4944=EDGE_LOOP('',(#21360));
#4945=EDGE_LOOP('',(#21361,#21362,#21363,#21364));
#4946=EDGE_LOOP('',(#21365,#21366,#21367,#21368));
#4947=EDGE_LOOP('',(#21369,#21370,#21371,#21372));
#4948=EDGE_LOOP('',(#21373,#21374,#21375,#21376));
#4949=EDGE_LOOP('',(#21377));
#4950=EDGE_LOOP('',(#21378,#21379,#21380,#21381));
#4951=EDGE_LOOP('',(#21382));
#4952=EDGE_LOOP('',(#21383,#21384,#21385,#21386));
#4953=EDGE_LOOP('',(#21387,#21388,#21389,#21390));
#4954=EDGE_LOOP('',(#21391,#21392,#21393,#21394));
#4955=EDGE_LOOP('',(#21395,#21396,#21397,#21398,#21399,#21400));
#4956=EDGE_LOOP('',(#21401,#21402,#21403,#21404));
#4957=EDGE_LOOP('',(#21405,#21406,#21407,#21408));
#4958=EDGE_LOOP('',(#21409));
#4959=EDGE_LOOP('',(#21410));
#4960=EDGE_LOOP('',(#21411,#21412,#21413,#21414));
#4961=EDGE_LOOP('',(#21415,#21416,#21417,#21418));
#4962=EDGE_LOOP('',(#21419,#21420,#21421,#21422));
#4963=EDGE_LOOP('',(#21423,#21424,#21425,#21426));
#4964=EDGE_LOOP('',(#21427,#21428,#21429,#21430));
#4965=EDGE_LOOP('',(#21431,#21432,#21433,#21434));
#4966=EDGE_LOOP('',(#21435,#21436,#21437,#21438));
#4967=EDGE_LOOP('',(#21439,#21440,#21441,#21442));
#4968=EDGE_LOOP('',(#21443));
#4969=EDGE_LOOP('',(#21444));
#4970=EDGE_LOOP('',(#21445,#21446,#21447,#21448));
#4971=EDGE_LOOP('',(#21449,#21450,#21451,#21452));
#4972=EDGE_LOOP('',(#21453,#21454,#21455,#21456));
#4973=EDGE_LOOP('',(#21457,#21458,#21459,#21460,#21461,#21462));
#4974=EDGE_LOOP('',(#21463,#21464,#21465,#21466,#21467,#21468));
#4975=EDGE_LOOP('',(#21469));
#4976=EDGE_LOOP('',(#21470,#21471,#21472,#21473));
#4977=EDGE_LOOP('',(#21474,#21475,#21476,#21477));
#4978=EDGE_LOOP('',(#21478,#21479,#21480,#21481));
#4979=EDGE_LOOP('',(#21482,#21483,#21484,#21485));
#4980=EDGE_LOOP('',(#21486,#21487,#21488,#21489,#21490,#21491));
#4981=EDGE_LOOP('',(#21492));
#4982=EDGE_LOOP('',(#21493,#21494,#21495,#21496));
#4983=EDGE_LOOP('',(#21497,#21498,#21499,#21500));
#4984=EDGE_LOOP('',(#21501,#21502,#21503,#21504));
#4985=EDGE_LOOP('',(#21505,#21506,#21507,#21508,#21509,#21510,#21511,#21512,
#21513,#21514,#21515,#21516,#21517,#21518,#21519,#21520,#21521,#21522,#21523,
#21524,#21525,#21526,#21527,#21528,#21529,#21530,#21531,#21532,#21533,#21534,
#21535,#21536,#21537,#21538,#21539,#21540));
#4986=EDGE_LOOP('',(#21541,#21542,#21543,#21544));
#4987=EDGE_LOOP('',(#21545,#21546,#21547,#21548,#21549,#21550,#21551,#21552,
#21553,#21554,#21555,#21556,#21557,#21558,#21559,#21560,#21561,#21562,#21563,
#21564,#21565,#21566,#21567,#21568,#21569,#21570,#21571,#21572,#21573,#21574,
#21575,#21576,#21577,#21578,#21579,#21580,#21581,#21582,#21583,#21584,#21585,
#21586,#21587,#21588,#21589,#21590,#21591,#21592));
#4988=EDGE_LOOP('',(#21593,#21594,#21595,#21596,#21597,#21598,#21599,#21600,
#21601,#21602,#21603,#21604,#21605,#21606,#21607,#21608,#21609,#21610,#21611,
#21612,#21613,#21614,#21615,#21616,#21617,#21618,#21619,#21620,#21621,#21622,
#21623,#21624,#21625,#21626,#21627,#21628,#21629,#21630,#21631,#21632,#21633,
#21634,#21635,#21636));
#4989=EDGE_LOOP('',(#21637,#21638,#21639,#21640,#21641,#21642,#21643,#21644,
#21645,#21646,#21647,#21648,#21649,#21650,#21651,#21652,#21653,#21654,#21655,
#21656,#21657,#21658,#21659,#21660,#21661,#21662,#21663,#21664,#21665,#21666,
#21667,#21668,#21669,#21670,#21671,#21672));
#4990=EDGE_LOOP('',(#21673,#21674,#21675,#21676));
#4991=EDGE_LOOP('',(#21677,#21678,#21679,#21680));
#4992=EDGE_LOOP('',(#21681,#21682,#21683,#21684));
#4993=EDGE_LOOP('',(#21685));
#4994=EDGE_LOOP('',(#21686,#21687,#21688,#21689));
#4995=EDGE_LOOP('',(#21690,#21691,#21692,#21693));
#4996=EDGE_LOOP('',(#21694,#21695,#21696,#21697));
#4997=EDGE_LOOP('',(#21698,#21699,#21700,#21701));
#4998=EDGE_LOOP('',(#21702,#21703,#21704,#21705));
#4999=EDGE_LOOP('',(#21706,#21707,#21708,#21709));
#5000=EDGE_LOOP('',(#21710,#21711,#21712,#21713,#21714,#21715,#21716,#21717,
#21718,#21719));
#5001=EDGE_LOOP('',(#21720,#21721,#21722,#21723));
#5002=EDGE_LOOP('',(#21724,#21725,#21726,#21727));
#5003=EDGE_LOOP('',(#21728,#21729,#21730,#21731));
#5004=EDGE_LOOP('',(#21732,#21733,#21734,#21735));
#5005=EDGE_LOOP('',(#21736,#21737,#21738,#21739));
#5006=EDGE_LOOP('',(#21740,#21741,#21742,#21743));
#5007=EDGE_LOOP('',(#21744,#21745,#21746,#21747));
#5008=EDGE_LOOP('',(#21748,#21749,#21750,#21751));
#5009=EDGE_LOOP('',(#21752,#21753,#21754,#21755));
#5010=EDGE_LOOP('',(#21756,#21757,#21758,#21759));
#5011=EDGE_LOOP('',(#21760,#21761,#21762,#21763));
#5012=EDGE_LOOP('',(#21764,#21765,#21766,#21767));
#5013=EDGE_LOOP('',(#21768,#21769,#21770,#21771));
#5014=EDGE_LOOP('',(#21772,#21773,#21774,#21775));
#5015=EDGE_LOOP('',(#21776,#21777,#21778,#21779));
#5016=EDGE_LOOP('',(#21780,#21781,#21782,#21783));
#5017=EDGE_LOOP('',(#21784,#21785,#21786,#21787));
#5018=EDGE_LOOP('',(#21788,#21789,#21790,#21791));
#5019=EDGE_LOOP('',(#21792,#21793,#21794,#21795));
#5020=EDGE_LOOP('',(#21796,#21797,#21798,#21799));
#5021=EDGE_LOOP('',(#21800,#21801,#21802,#21803));
#5022=EDGE_LOOP('',(#21804,#21805,#21806,#21807));
#5023=EDGE_LOOP('',(#21808,#21809,#21810,#21811));
#5024=EDGE_LOOP('',(#21812,#21813,#21814,#21815));
#5025=EDGE_LOOP('',(#21816,#21817,#21818,#21819));
#5026=EDGE_LOOP('',(#21820,#21821,#21822,#21823));
#5027=EDGE_LOOP('',(#21824,#21825,#21826,#21827));
#5028=EDGE_LOOP('',(#21828));
#5029=EDGE_LOOP('',(#21829,#21830,#21831,#21832));
#5030=EDGE_LOOP('',(#21833,#21834,#21835,#21836));
#5031=EDGE_LOOP('',(#21837,#21838,#21839,#21840,#21841,#21842,#21843,#21844,
#21845,#21846));
#5032=EDGE_LOOP('',(#21847,#21848,#21849,#21850));
#5033=EDGE_LOOP('',(#21851,#21852,#21853,#21854));
#5034=EDGE_LOOP('',(#21855,#21856,#21857,#21858));
#5035=EDGE_LOOP('',(#21859,#21860,#21861,#21862));
#5036=EDGE_LOOP('',(#21863,#21864,#21865,#21866));
#5037=EDGE_LOOP('',(#21867,#21868,#21869,#21870));
#5038=EDGE_LOOP('',(#21871,#21872,#21873,#21874));
#5039=EDGE_LOOP('',(#21875,#21876,#21877,#21878));
#5040=EDGE_LOOP('',(#21879));
#5041=EDGE_LOOP('',(#21880,#21881,#21882,#21883,#21884,#21885,#21886,#21887,
#21888,#21889,#21890,#21891,#21892,#21893,#21894,#21895,#21896,#21897,#21898,
#21899,#21900,#21901,#21902,#21903,#21904,#21905,#21906,#21907,#21908,#21909,
#21910,#21911,#21912,#21913,#21914,#21915,#21916,#21917,#21918,#21919,#21920,
#21921,#21922,#21923,#21924,#21925,#21926,#21927));
#5042=EDGE_LOOP('',(#21928,#21929,#21930,#21931,#21932,#21933,#21934,#21935,
#21936,#21937,#21938,#21939,#21940,#21941,#21942,#21943,#21944,#21945,#21946,
#21947,#21948,#21949,#21950,#21951,#21952,#21953,#21954,#21955,#21956,#21957,
#21958,#21959,#21960,#21961,#21962,#21963,#21964,#21965,#21966,#21967,#21968,
#21969,#21970,#21971));
#5043=EDGE_LOOP('',(#21972,#21973,#21974,#21975));
#5044=EDGE_LOOP('',(#21976,#21977,#21978,#21979));
#5045=EDGE_LOOP('',(#21980,#21981,#21982,#21983));
#5046=EDGE_LOOP('',(#21984,#21985,#21986,#21987));
#5047=EDGE_LOOP('',(#21988,#21989,#21990,#21991,#21992,#21993,#21994));
#5048=EDGE_LOOP('',(#21995,#21996,#21997,#21998,#21999,#22000,#22001));
#5049=EDGE_LOOP('',(#22002,#22003,#22004,#22005,#22006,#22007,#22008));
#5050=EDGE_LOOP('',(#22009,#22010,#22011,#22012,#22013,#22014,#22015));
#6305=LINE('',#54041,#8272);
#6306=LINE('',#54047,#8273);
#6307=LINE('',#54053,#8274);
#6308=LINE('',#54057,#8275);
#6309=LINE('',#54060,#8276);
#6310=LINE('',#54065,#8277);
#6311=LINE('',#54071,#8278);
#6312=LINE('',#54077,#8279);
#6313=LINE('',#54083,#8280);
#6314=LINE('',#54089,#8281);
#6315=LINE('',#54095,#8282);
#6316=LINE('',#54101,#8283);
#6317=LINE('',#54107,#8284);
#6318=LINE('',#54111,#8285);
#6319=LINE('',#54114,#8286);
#6320=LINE('',#54117,#8287);
#6321=LINE('',#54120,#8288);
#6322=LINE('',#54125,#8289);
#6323=LINE('',#54127,#8290);
#6324=LINE('',#54131,#8291);
#6325=LINE('',#54236,#8292);
#6326=LINE('',#54241,#8293);
#6327=LINE('',#54248,#8294);
#6328=LINE('',#54250,#8295);
#6329=LINE('',#54251,#8296);
#6330=LINE('',#54256,#8297);
#6331=LINE('',#54259,#8298);
#6332=LINE('',#54265,#8299);
#6333=LINE('',#54268,#8300);
#6334=LINE('',#54273,#8301);
#6335=LINE('',#54275,#8302);
#6336=LINE('',#54276,#8303);
#6337=LINE('',#54280,#8304);
#6338=LINE('',#54282,#8305);
#6339=LINE('',#54284,#8306);
#6340=LINE('',#54285,#8307);
#6341=LINE('',#54289,#8308);
#6342=LINE('',#54291,#8309);
#6343=LINE('',#54293,#8310);
#6344=LINE('',#54294,#8311);
#6345=LINE('',#54298,#8312);
#6346=LINE('',#54300,#8313);
#6347=LINE('',#54302,#8314);
#6348=LINE('',#54303,#8315);
#6349=LINE('',#54307,#8316);
#6350=LINE('',#54309,#8317);
#6351=LINE('',#54311,#8318);
#6352=LINE('',#54312,#8319);
#6353=LINE('',#54316,#8320);
#6354=LINE('',#54318,#8321);
#6355=LINE('',#54320,#8322);
#6356=LINE('',#54321,#8323);
#6357=LINE('',#54325,#8324);
#6358=LINE('',#54327,#8325);
#6359=LINE('',#54329,#8326);
#6360=LINE('',#54330,#8327);
#6361=LINE('',#54334,#8328);
#6362=LINE('',#54336,#8329);
#6363=LINE('',#54338,#8330);
#6364=LINE('',#54339,#8331);
#6365=LINE('',#54343,#8332);
#6366=LINE('',#54345,#8333);
#6367=LINE('',#54347,#8334);
#6368=LINE('',#54348,#8335);
#6369=LINE('',#54352,#8336);
#6370=LINE('',#54354,#8337);
#6371=LINE('',#54356,#8338);
#6372=LINE('',#54357,#8339);
#6373=LINE('',#54360,#8340);
#6374=LINE('',#54362,#8341);
#6375=LINE('',#54363,#8342);
#6376=LINE('',#54367,#8343);
#6377=LINE('',#54369,#8344);
#6378=LINE('',#54371,#8345);
#6379=LINE('',#54372,#8346);
#6380=LINE('',#54375,#8347);
#6381=LINE('',#54377,#8348);
#6382=LINE('',#54378,#8349);
#6383=LINE('',#54382,#8350);
#6384=LINE('',#54384,#8351);
#6385=LINE('',#54386,#8352);
#6386=LINE('',#54387,#8353);
#6387=LINE('',#54391,#8354);
#6388=LINE('',#54393,#8355);
#6389=LINE('',#54395,#8356);
#6390=LINE('',#54396,#8357);
#6391=LINE('',#54400,#8358);
#6392=LINE('',#54402,#8359);
#6393=LINE('',#54404,#8360);
#6394=LINE('',#54405,#8361);
#6395=LINE('',#54409,#8362);
#6396=LINE('',#54411,#8363);
#6397=LINE('',#54413,#8364);
#6398=LINE('',#54414,#8365);
#6399=LINE('',#54416,#8366);
#6400=LINE('',#54417,#8367);
#6401=LINE('',#54423,#8368);
#6402=LINE('',#54426,#8369);
#6403=LINE('',#54432,#8370);
#6404=LINE('',#54435,#8371);
#6405=LINE('',#54441,#8372);
#6406=LINE('',#54444,#8373);
#6407=LINE('',#54450,#8374);
#6408=LINE('',#54453,#8375);
#6409=LINE('',#54506,#8376);
#6410=LINE('',#54508,#8377);
#6411=LINE('',#54510,#8378);
#6412=LINE('',#54511,#8379);
#6413=LINE('',#54514,#8380);
#6414=LINE('',#54516,#8381);
#6415=LINE('',#54517,#8382);
#6416=LINE('',#54519,#8383);
#6417=LINE('',#54521,#8384);
#6418=LINE('',#54522,#8385);
#6419=LINE('',#54525,#8386);
#6420=LINE('',#54526,#8387);
#6421=LINE('',#54529,#8388);
#6422=LINE('',#54530,#8389);
#6423=LINE('',#54532,#8390);
#6424=LINE('',#54535,#8391);
#6425=LINE('',#54536,#8392);
#6426=LINE('',#54539,#8393);
#6427=LINE('',#54540,#8394);
#6428=LINE('',#54542,#8395);
#6429=LINE('',#54545,#8396);
#6430=LINE('',#54547,#8397);
#6431=LINE('',#54548,#8398);
#6432=LINE('',#54551,#8399);
#6433=LINE('',#54552,#8400);
#6434=LINE('',#54555,#8401);
#6435=LINE('',#54556,#8402);
#6436=LINE('',#54559,#8403);
#6437=LINE('',#54560,#8404);
#6438=LINE('',#54563,#8405);
#6439=LINE('',#54564,#8406);
#6440=LINE('',#54566,#8407);
#6441=LINE('',#54571,#8408);
#6442=LINE('',#54575,#8409);
#6443=LINE('',#54579,#8410);
#6444=LINE('',#54587,#8411);
#6445=LINE('',#54591,#8412);
#6446=LINE('',#54595,#8413);
#6447=LINE('',#54603,#8414);
#6448=LINE('',#54605,#8415);
#6449=LINE('',#54607,#8416);
#6450=LINE('',#54615,#8417);
#6451=LINE('',#54619,#8418);
#6452=LINE('',#54623,#8419);
#6453=LINE('',#54631,#8420);
#6454=LINE('',#54635,#8421);
#6455=LINE('',#54639,#8422);
#6456=LINE('',#54641,#8423);
#6457=LINE('',#54643,#8424);
#6458=LINE('',#54645,#8425);
#6459=LINE('',#54647,#8426);
#6460=LINE('',#54649,#8427);
#6461=LINE('',#54651,#8428);
#6462=LINE('',#54653,#8429);
#6463=LINE('',#54655,#8430);
#6464=LINE('',#54656,#8431);
#6465=LINE('',#54660,#8432);
#6466=LINE('',#54661,#8433);
#6467=LINE('',#54662,#8434);
#6468=LINE('',#54666,#8435);
#6469=LINE('',#54669,#8436);
#6470=LINE('',#54670,#8437);
#6471=LINE('',#54674,#8438);
#6472=LINE('',#54677,#8439);
#6473=LINE('',#54678,#8440);
#6474=LINE('',#54682,#8441);
#6475=LINE('',#54686,#8442);
#6476=LINE('',#54690,#8443);
#6477=LINE('',#54693,#8444);
#6478=LINE('',#54694,#8445);
#6479=LINE('',#54698,#8446);
#6480=LINE('',#54701,#8447);
#6481=LINE('',#54702,#8448);
#6482=LINE('',#54706,#8449);
#6483=LINE('',#54709,#8450);
#6484=LINE('',#54710,#8451);
#6485=LINE('',#54714,#8452);
#6486=LINE('',#54718,#8453);
#6487=LINE('',#54722,#8454);
#6488=LINE('',#54725,#8455);
#6489=LINE('',#54726,#8456);
#6490=LINE('',#54729,#8457);
#6491=LINE('',#54730,#8458);
#6492=LINE('',#54733,#8459);
#6493=LINE('',#54734,#8460);
#6494=LINE('',#54738,#8461);
#6495=LINE('',#54742,#8462);
#6496=LINE('',#54746,#8463);
#6497=LINE('',#54749,#8464);
#6498=LINE('',#54750,#8465);
#6499=LINE('',#54754,#8466);
#6500=LINE('',#54757,#8467);
#6501=LINE('',#54758,#8468);
#6502=LINE('',#54762,#8469);
#6503=LINE('',#54765,#8470);
#6504=LINE('',#54766,#8471);
#6505=LINE('',#54770,#8472);
#6506=LINE('',#54774,#8473);
#6507=LINE('',#54778,#8474);
#6508=LINE('',#54781,#8475);
#6509=LINE('',#54782,#8476);
#6510=LINE('',#54786,#8477);
#6511=LINE('',#54789,#8478);
#6512=LINE('',#54790,#8479);
#6513=LINE('',#54794,#8480);
#6514=LINE('',#54797,#8481);
#6515=LINE('',#54798,#8482);
#6516=LINE('',#54801,#8483);
#6517=LINE('',#54802,#8484);
#6518=LINE('',#54805,#8485);
#6519=LINE('',#54806,#8486);
#6520=LINE('',#54809,#8487);
#6521=LINE('',#54810,#8488);
#6522=LINE('',#54813,#8489);
#6523=LINE('',#54814,#8490);
#6524=LINE('',#54817,#8491);
#6525=LINE('',#54818,#8492);
#6526=LINE('',#54821,#8493);
#6527=LINE('',#54822,#8494);
#6528=LINE('',#54825,#8495);
#6529=LINE('',#54826,#8496);
#6530=LINE('',#54829,#8497);
#6531=LINE('',#54830,#8498);
#6532=LINE('',#54832,#8499);
#6533=LINE('',#54836,#8500);
#6534=LINE('',#54839,#8501);
#6535=LINE('',#54843,#8502);
#6536=LINE('',#54845,#8503);
#6537=LINE('',#54849,#8504);
#6538=LINE('',#54851,#8505);
#6539=LINE('',#54853,#8506);
#6540=LINE('',#54855,#8507);
#6541=LINE('',#54857,#8508);
#6542=LINE('',#54859,#8509);
#6543=LINE('',#54861,#8510);
#6544=LINE('',#54865,#8511);
#6545=LINE('',#54869,#8512);
#6546=LINE('',#54877,#8513);
#6547=LINE('',#54881,#8514);
#6548=LINE('',#54885,#8515);
#6549=LINE('',#54893,#8516);
#6550=LINE('',#54895,#8517);
#6551=LINE('',#54897,#8518);
#6552=LINE('',#54905,#8519);
#6553=LINE('',#54909,#8520);
#6554=LINE('',#54913,#8521);
#6555=LINE('',#54921,#8522);
#6556=LINE('',#54925,#8523);
#6557=LINE('',#54929,#8524);
#6558=LINE('',#54931,#8525);
#6559=LINE('',#54933,#8526);
#6560=LINE('',#54935,#8527);
#6561=LINE('',#54936,#8528);
#6562=LINE('',#54939,#8529);
#6563=LINE('',#54940,#8530);
#6564=LINE('',#54943,#8531);
#6565=LINE('',#54944,#8532);
#6566=LINE('',#54950,#8533);
#6567=LINE('',#54953,#8534);
#6568=LINE('',#54957,#8535);
#6569=LINE('',#54958,#8536);
#6570=LINE('',#54959,#8537);
#6571=LINE('',#54962,#8538);
#6572=LINE('',#54963,#8539);
#6573=LINE('',#54966,#8540);
#6574=LINE('',#54967,#8541);
#6575=LINE('',#54970,#8542);
#6576=LINE('',#54971,#8543);
#6577=LINE('',#54975,#8544);
#6578=LINE('',#54976,#8545);
#6579=LINE('',#54978,#8546);
#6580=LINE('',#54979,#8547);
#6581=LINE('',#54980,#8548);
#6582=LINE('',#54983,#8549);
#6583=LINE('',#54984,#8550);
#6584=LINE('',#54987,#8551);
#6585=LINE('',#54988,#8552);
#6586=LINE('',#54991,#8553);
#6587=LINE('',#54992,#8554);
#6588=LINE('',#54995,#8555);
#6589=LINE('',#54996,#8556);
#6590=LINE('',#54999,#8557);
#6591=LINE('',#55000,#8558);
#6592=LINE('',#55004,#8559);
#6593=LINE('',#55007,#8560);
#6594=LINE('',#55008,#8561);
#6595=LINE('',#55012,#8562);
#6596=LINE('',#55015,#8563);
#6597=LINE('',#55016,#8564);
#6598=LINE('',#55020,#8565);
#6599=LINE('',#55024,#8566);
#6600=LINE('',#55028,#8567);
#6601=LINE('',#55031,#8568);
#6602=LINE('',#55032,#8569);
#6603=LINE('',#55036,#8570);
#6604=LINE('',#55039,#8571);
#6605=LINE('',#55040,#8572);
#6606=LINE('',#55044,#8573);
#6607=LINE('',#55047,#8574);
#6608=LINE('',#55048,#8575);
#6609=LINE('',#55052,#8576);
#6610=LINE('',#55056,#8577);
#6611=LINE('',#55060,#8578);
#6612=LINE('',#55063,#8579);
#6613=LINE('',#55064,#8580);
#6614=LINE('',#55067,#8581);
#6615=LINE('',#55068,#8582);
#6616=LINE('',#55071,#8583);
#6617=LINE('',#55072,#8584);
#6618=LINE('',#55076,#8585);
#6619=LINE('',#55080,#8586);
#6620=LINE('',#55084,#8587);
#6621=LINE('',#55087,#8588);
#6622=LINE('',#55088,#8589);
#6623=LINE('',#55092,#8590);
#6624=LINE('',#55095,#8591);
#6625=LINE('',#55096,#8592);
#6626=LINE('',#55100,#8593);
#6627=LINE('',#55103,#8594);
#6628=LINE('',#55104,#8595);
#6629=LINE('',#55108,#8596);
#6630=LINE('',#55112,#8597);
#6631=LINE('',#55116,#8598);
#6632=LINE('',#55119,#8599);
#6633=LINE('',#55120,#8600);
#6634=LINE('',#55124,#8601);
#6635=LINE('',#55127,#8602);
#6636=LINE('',#55128,#8603);
#6637=LINE('',#55132,#8604);
#6638=LINE('',#55134,#8605);
#6639=LINE('',#55139,#8606);
#6640=LINE('',#55141,#8607);
#6641=LINE('',#55143,#8608);
#6642=LINE('',#55144,#8609);
#6643=LINE('',#55148,#8610);
#6644=LINE('',#55150,#8611);
#6645=LINE('',#55152,#8612);
#6646=LINE('',#55153,#8613);
#6647=LINE('',#55156,#8614);
#6648=LINE('',#55157,#8615);
#6649=LINE('',#55160,#8616);
#6650=LINE('',#55161,#8617);
#6651=LINE('',#55169,#8618);
#6652=LINE('',#55172,#8619);
#6653=LINE('',#55174,#8620);
#6654=LINE('',#55176,#8621);
#6655=LINE('',#55177,#8622);
#6656=LINE('',#55180,#8623);
#6657=LINE('',#55182,#8624);
#6658=LINE('',#55183,#8625);
#6659=LINE('',#55187,#8626);
#6660=LINE('',#55189,#8627);
#6661=LINE('',#55191,#8628);
#6662=LINE('',#55192,#8629);
#6663=LINE('',#55195,#8630);
#6664=LINE('',#55198,#8631);
#6665=LINE('',#55199,#8632);
#6666=LINE('',#55202,#8633);
#6667=LINE('',#55207,#8634);
#6668=LINE('',#55209,#8635);
#6669=LINE('',#55211,#8636);
#6670=LINE('',#55213,#8637);
#6671=LINE('',#55215,#8638);
#6672=LINE('',#55217,#8639);
#6673=LINE('',#55219,#8640);
#6674=LINE('',#55221,#8641);
#6675=LINE('',#55223,#8642);
#6676=LINE('',#55225,#8643);
#6677=LINE('',#55229,#8644);
#6678=LINE('',#55233,#8645);
#6679=LINE('',#55241,#8646);
#6680=LINE('',#55245,#8647);
#6681=LINE('',#55249,#8648);
#6682=LINE('',#55257,#8649);
#6683=LINE('',#55259,#8650);
#6684=LINE('',#55261,#8651);
#6685=LINE('',#55269,#8652);
#6686=LINE('',#55273,#8653);
#6687=LINE('',#55277,#8654);
#6688=LINE('',#55285,#8655);
#6689=LINE('',#55289,#8656);
#6690=LINE('',#55292,#8657);
#6691=LINE('',#55295,#8658);
#6692=LINE('',#55296,#8659);
#6693=LINE('',#55299,#8660);
#6694=LINE('',#55300,#8661);
#6695=LINE('',#55304,#8662);
#6696=LINE('',#55305,#8663);
#6697=LINE('',#55306,#8664);
#6698=LINE('',#55309,#8665);
#6699=LINE('',#55311,#8666);
#6700=LINE('',#55312,#8667);
#6701=LINE('',#55315,#8668);
#6702=LINE('',#55317,#8669);
#6703=LINE('',#55318,#8670);
#6704=LINE('',#55321,#8671);
#6705=LINE('',#55323,#8672);
#6706=LINE('',#55324,#8673);
#6707=LINE('',#55333,#8674);
#6708=LINE('',#55335,#8675);
#6709=LINE('',#55336,#8676);
#6710=LINE('',#55340,#8677);
#6711=LINE('',#55341,#8678);
#6712=LINE('',#55342,#8679);
#6713=LINE('',#55347,#8680);
#6714=LINE('',#55348,#8681);
#6715=LINE('',#55352,#8682);
#6716=LINE('',#55353,#8683);
#6717=LINE('',#55354,#8684);
#6718=LINE('',#55357,#8685);
#6719=LINE('',#55358,#8686);
#6720=LINE('',#55364,#8687);
#6721=LINE('',#55365,#8688);
#6722=LINE('',#55372,#8689);
#6723=LINE('',#55373,#8690);
#6724=LINE('',#55374,#8691);
#6725=LINE('',#55377,#8692);
#6726=LINE('',#55378,#8693);
#6727=LINE('',#55381,#8694);
#6728=LINE('',#55382,#8695);
#6729=LINE('',#55385,#8696);
#6730=LINE('',#55386,#8697);
#6731=LINE('',#55389,#8698);
#6732=LINE('',#55390,#8699);
#6733=LINE('',#55393,#8700);
#6734=LINE('',#55394,#8701);
#6735=LINE('',#55397,#8702);
#6736=LINE('',#55398,#8703);
#6737=LINE('',#55401,#8704);
#6738=LINE('',#55402,#8705);
#6739=LINE('',#55405,#8706);
#6740=LINE('',#55406,#8707);
#6741=LINE('',#55409,#8708);
#6742=LINE('',#55410,#8709);
#6743=LINE('',#55414,#8710);
#6744=LINE('',#55417,#8711);
#6745=LINE('',#55418,#8712);
#6746=LINE('',#55422,#8713);
#6747=LINE('',#55425,#8714);
#6748=LINE('',#55426,#8715);
#6749=LINE('',#55430,#8716);
#6750=LINE('',#55434,#8717);
#6751=LINE('',#55438,#8718);
#6752=LINE('',#55441,#8719);
#6753=LINE('',#55442,#8720);
#6754=LINE('',#55446,#8721);
#6755=LINE('',#55449,#8722);
#6756=LINE('',#55450,#8723);
#6757=LINE('',#55454,#8724);
#6758=LINE('',#55457,#8725);
#6759=LINE('',#55458,#8726);
#6760=LINE('',#55462,#8727);
#6761=LINE('',#55466,#8728);
#6762=LINE('',#55470,#8729);
#6763=LINE('',#55473,#8730);
#6764=LINE('',#55474,#8731);
#6765=LINE('',#55477,#8732);
#6766=LINE('',#55478,#8733);
#6767=LINE('',#55481,#8734);
#6768=LINE('',#55482,#8735);
#6769=LINE('',#55486,#8736);
#6770=LINE('',#55490,#8737);
#6771=LINE('',#55494,#8738);
#6772=LINE('',#55497,#8739);
#6773=LINE('',#55498,#8740);
#6774=LINE('',#55502,#8741);
#6775=LINE('',#55505,#8742);
#6776=LINE('',#55506,#8743);
#6777=LINE('',#55510,#8744);
#6778=LINE('',#55513,#8745);
#6779=LINE('',#55514,#8746);
#6780=LINE('',#55518,#8747);
#6781=LINE('',#55522,#8748);
#6782=LINE('',#55526,#8749);
#6783=LINE('',#55529,#8750);
#6784=LINE('',#55530,#8751);
#6785=LINE('',#55534,#8752);
#6786=LINE('',#55537,#8753);
#6787=LINE('',#55538,#8754);
#6788=LINE('',#55542,#8755);
#6789=LINE('',#55544,#8756);
#6790=LINE('',#55548,#8757);
#6791=LINE('',#55550,#8758);
#6792=LINE('',#55552,#8759);
#6793=LINE('',#55553,#8760);
#6794=LINE('',#55556,#8761);
#6795=LINE('',#55558,#8762);
#6796=LINE('',#55559,#8763);
#6797=LINE('',#55562,#8764);
#6798=LINE('',#55564,#8765);
#6799=LINE('',#55565,#8766);
#6800=LINE('',#55568,#8767);
#6801=LINE('',#55570,#8768);
#6802=LINE('',#55571,#8769);
#6803=LINE('',#55574,#8770);
#6804=LINE('',#55576,#8771);
#6805=LINE('',#55577,#8772);
#6806=LINE('',#55581,#8773);
#6807=LINE('',#55583,#8774);
#6808=LINE('',#55585,#8775);
#6809=LINE('',#55586,#8776);
#6810=LINE('',#55589,#8777);
#6811=LINE('',#55591,#8778);
#6812=LINE('',#55592,#8779);
#6813=LINE('',#55595,#8780);
#6814=LINE('',#55597,#8781);
#6815=LINE('',#55598,#8782);
#6816=LINE('',#55600,#8783);
#6817=LINE('',#55601,#8784);
#6818=LINE('',#55604,#8785);
#6819=LINE('',#55606,#8786);
#6820=LINE('',#55608,#8787);
#6821=LINE('',#55609,#8788);
#6822=LINE('',#55612,#8789);
#6823=LINE('',#55614,#8790);
#6824=LINE('',#55615,#8791);
#6825=LINE('',#55619,#8792);
#6826=LINE('',#55620,#8793);
#6827=LINE('',#55621,#8794);
#6828=LINE('',#55625,#8795);
#6829=LINE('',#55626,#8796);
#6830=LINE('',#55627,#8797);
#6831=LINE('',#55631,#8798);
#6832=LINE('',#55632,#8799);
#6833=LINE('',#55633,#8800);
#6834=LINE('',#55637,#8801);
#6835=LINE('',#55638,#8802);
#6836=LINE('',#55639,#8803);
#6837=LINE('',#55642,#8804);
#6838=LINE('',#55644,#8805);
#6839=LINE('',#55645,#8806);
#6840=LINE('',#55649,#8807);
#6841=LINE('',#55650,#8808);
#6842=LINE('',#55651,#8809);
#6843=LINE('',#55655,#8810);
#6844=LINE('',#55656,#8811);
#6845=LINE('',#55657,#8812);
#6846=LINE('',#55661,#8813);
#6847=LINE('',#55662,#8814);
#6848=LINE('',#55663,#8815);
#6849=LINE('',#55666,#8816);
#6850=LINE('',#55668,#8817);
#6851=LINE('',#55669,#8818);
#6852=LINE('',#55672,#8819);
#6853=LINE('',#55674,#8820);
#6854=LINE('',#55675,#8821);
#6855=LINE('',#55678,#8822);
#6856=LINE('',#55680,#8823);
#6857=LINE('',#55681,#8824);
#6858=LINE('',#55684,#8825);
#6859=LINE('',#55686,#8826);
#6860=LINE('',#55687,#8827);
#6861=LINE('',#55690,#8828);
#6862=LINE('',#55691,#8829);
#6863=LINE('',#55692,#8830);
#6864=LINE('',#55697,#8831);
#6865=LINE('',#55698,#8832);
#6866=LINE('',#55702,#8833);
#6867=LINE('',#55703,#8834);
#6868=LINE('',#55704,#8835);
#6869=LINE('',#55709,#8836);
#6870=LINE('',#55710,#8837);
#6871=LINE('',#55715,#8838);
#6872=LINE('',#55716,#8839);
#6873=LINE('',#55720,#8840);
#6874=LINE('',#55721,#8841);
#6875=LINE('',#55722,#8842);
#6876=LINE('',#55724,#8843);
#6877=LINE('',#55729,#8844);
#6878=LINE('',#55730,#8845);
#6879=LINE('',#55733,#8846);
#6880=LINE('',#55735,#8847);
#6881=LINE('',#55736,#8848);
#6882=LINE('',#55739,#8849);
#6883=LINE('',#55741,#8850);
#6884=LINE('',#55742,#8851);
#6885=LINE('',#55744,#8852);
#6886=LINE('',#55746,#8853);
#6887=LINE('',#55747,#8854);
#6888=LINE('',#55750,#8855);
#6889=LINE('',#55753,#8856);
#6890=LINE('',#55755,#8857);
#6891=LINE('',#55759,#8858);
#6892=LINE('',#55763,#8859);
#6893=LINE('',#55771,#8860);
#6894=LINE('',#55775,#8861);
#6895=LINE('',#55779,#8862);
#6896=LINE('',#55787,#8863);
#6897=LINE('',#55789,#8864);
#6898=LINE('',#55791,#8865);
#6899=LINE('',#55799,#8866);
#6900=LINE('',#55803,#8867);
#6901=LINE('',#55807,#8868);
#6902=LINE('',#55815,#8869);
#6903=LINE('',#55819,#8870);
#6904=LINE('',#55823,#8871);
#6905=LINE('',#55824,#8872);
#6906=LINE('',#55827,#8873);
#6907=LINE('',#55829,#8874);
#6908=LINE('',#55831,#8875);
#6909=LINE('',#55833,#8876);
#6910=LINE('',#55835,#8877);
#6911=LINE('',#55837,#8878);
#6912=LINE('',#55839,#8879);
#6913=LINE('',#55841,#8880);
#6914=LINE('',#55843,#8881);
#6915=LINE('',#55845,#8882);
#6916=LINE('',#55847,#8883);
#6917=LINE('',#55849,#8884);
#6918=LINE('',#55850,#8885);
#6919=LINE('',#55854,#8886);
#6920=LINE('',#55855,#8887);
#6921=LINE('',#55856,#8888);
#6922=LINE('',#55860,#8889);
#6923=LINE('',#55861,#8890);
#6924=LINE('',#55862,#8891);
#6925=LINE('',#55865,#8892);
#6926=LINE('',#55866,#8893);
#6927=LINE('',#55869,#8894);
#6928=LINE('',#55870,#8895);
#6929=LINE('',#55873,#8896);
#6930=LINE('',#55874,#8897);
#6931=LINE('',#55877,#8898);
#6932=LINE('',#55880,#8899);
#6933=LINE('',#55883,#8900);
#6934=LINE('',#55886,#8901);
#6935=LINE('',#55888,#8902);
#6936=LINE('',#55891,#8903);
#6937=LINE('',#55892,#8904);
#6938=LINE('',#55894,#8905);
#6939=LINE('',#55899,#8906);
#6940=LINE('',#55900,#8907);
#6941=LINE('',#55905,#8908);
#6942=LINE('',#55906,#8909);
#6943=LINE('',#55913,#8910);
#6944=LINE('',#55914,#8911);
#6945=LINE('',#55919,#8912);
#6946=LINE('',#55920,#8913);
#6947=LINE('',#55922,#8914);
#6948=LINE('',#55924,#8915);
#6949=LINE('',#55929,#8916);
#6950=LINE('',#55930,#8917);
#6951=LINE('',#55935,#8918);
#6952=LINE('',#55936,#8919);
#6953=LINE('',#55941,#8920);
#6954=LINE('',#55943,#8921);
#6955=LINE('',#55944,#8922);
#6956=LINE('',#55946,#8923);
#6957=LINE('',#55951,#8924);
#6958=LINE('',#55952,#8925);
#6959=LINE('',#55957,#8926);
#6960=LINE('',#55958,#8927);
#6961=LINE('',#55965,#8928);
#6962=LINE('',#55966,#8929);
#6963=LINE('',#55971,#8930);
#6964=LINE('',#55972,#8931);
#6965=LINE('',#55974,#8932);
#6966=LINE('',#55976,#8933);
#6967=LINE('',#55978,#8934);
#6968=LINE('',#55983,#8935);
#6969=LINE('',#55984,#8936);
#6970=LINE('',#55989,#8937);
#6971=LINE('',#55990,#8938);
#6972=LINE('',#55995,#8939);
#6973=LINE('',#55998,#8940);
#6974=LINE('',#56001,#8941);
#6975=LINE('',#56004,#8942);
#6976=LINE('',#56008,#8943);
#6977=LINE('',#56009,#8944);
#6978=LINE('',#56010,#8945);
#6979=LINE('',#56013,#8946);
#6980=LINE('',#56014,#8947);
#6981=LINE('',#56017,#8948);
#6982=LINE('',#56018,#8949);
#6983=LINE('',#56020,#8950);
#6984=LINE('',#56023,#8951);
#6985=LINE('',#56024,#8952);
#6986=LINE('',#56026,#8953);
#6987=LINE('',#56028,#8954);
#6988=LINE('',#56030,#8955);
#6989=LINE('',#56032,#8956);
#6990=LINE('',#56034,#8957);
#6991=LINE('',#56036,#8958);
#6992=LINE('',#56039,#8959);
#6993=LINE('',#56040,#8960);
#6994=LINE('',#56042,#8961);
#6995=LINE('',#56046,#8962);
#6996=LINE('',#56047,#8963);
#6997=LINE('',#56051,#8964);
#6998=LINE('',#56053,#8965);
#8272=VECTOR('',#31785,2.5);
#8273=VECTOR('',#31792,2.5);
#8274=VECTOR('',#31799,3.65);
#8275=VECTOR('',#31804,2.5);
#8276=VECTOR('',#31807,2.5);
#8277=VECTOR('',#31812,3.32349999999999);
#8278=VECTOR('',#31819,3.3235);
#8279=VECTOR('',#31826,3.32349999999999);
#8280=VECTOR('',#31833,3.3235);
#8281=VECTOR('',#31840,2.5);
#8282=VECTOR('',#31847,2.5);
#8283=VECTOR('',#31854,3.65);
#8284=VECTOR('',#31861,0.500000000000006);
#8285=VECTOR('',#31864,1000.);
#8286=VECTOR('',#31867,1000.);
#8287=VECTOR('',#31870,2.5);
#8288=VECTOR('',#31873,2.5);
#8289=VECTOR('',#31878,0.5);
#8290=VECTOR('',#31879,1000.);
#8291=VECTOR('',#31882,1000.);
#8292=VECTOR('',#31893,4.);
#8293=VECTOR('',#31898,4.99995);
#8294=VECTOR('',#31905,1000.);
#8295=VECTOR('',#31906,1000.);
#8296=VECTOR('',#31907,1000.);
#8297=VECTOR('',#31912,1000.);
#8298=VECTOR('',#31915,1000.);
#8299=VECTOR('',#31920,1000.);
#8300=VECTOR('',#31923,1000.);
#8301=VECTOR('',#31928,1000.);
#8302=VECTOR('',#31929,1000.);
#8303=VECTOR('',#31930,1000.);
#8304=VECTOR('',#31933,1000.);
#8305=VECTOR('',#31934,1000.);
#8306=VECTOR('',#31935,1000.);
#8307=VECTOR('',#31936,1000.);
#8308=VECTOR('',#31939,1000.);
#8309=VECTOR('',#31940,1000.);
#8310=VECTOR('',#31941,1000.);
#8311=VECTOR('',#31942,1000.);
#8312=VECTOR('',#31945,1000.);
#8313=VECTOR('',#31946,1000.);
#8314=VECTOR('',#31947,1000.);
#8315=VECTOR('',#31948,1000.);
#8316=VECTOR('',#31951,1000.);
#8317=VECTOR('',#31952,1000.);
#8318=VECTOR('',#31953,1000.);
#8319=VECTOR('',#31954,1000.);
#8320=VECTOR('',#31957,1000.);
#8321=VECTOR('',#31958,1000.);
#8322=VECTOR('',#31959,1000.);
#8323=VECTOR('',#31960,1000.);
#8324=VECTOR('',#31963,1000.);
#8325=VECTOR('',#31964,1000.);
#8326=VECTOR('',#31965,1000.);
#8327=VECTOR('',#31966,1000.);
#8328=VECTOR('',#31969,1000.);
#8329=VECTOR('',#31970,1000.);
#8330=VECTOR('',#31971,1000.);
#8331=VECTOR('',#31972,1000.);
#8332=VECTOR('',#31975,1000.);
#8333=VECTOR('',#31976,1000.);
#8334=VECTOR('',#31977,1000.);
#8335=VECTOR('',#31978,1000.);
#8336=VECTOR('',#31981,1000.);
#8337=VECTOR('',#31982,1000.);
#8338=VECTOR('',#31983,1000.);
#8339=VECTOR('',#31984,1000.);
#8340=VECTOR('',#31987,1000.);
#8341=VECTOR('',#31988,1000.);
#8342=VECTOR('',#31989,1000.);
#8343=VECTOR('',#31992,1000.);
#8344=VECTOR('',#31993,1000.);
#8345=VECTOR('',#31994,1000.);
#8346=VECTOR('',#31995,1000.);
#8347=VECTOR('',#31998,1000.);
#8348=VECTOR('',#31999,1000.);
#8349=VECTOR('',#32000,1000.);
#8350=VECTOR('',#32003,1000.);
#8351=VECTOR('',#32004,1000.);
#8352=VECTOR('',#32005,1000.);
#8353=VECTOR('',#32006,1000.);
#8354=VECTOR('',#32009,1000.);
#8355=VECTOR('',#32010,1000.);
#8356=VECTOR('',#32011,1000.);
#8357=VECTOR('',#32012,1000.);
#8358=VECTOR('',#32015,1000.);
#8359=VECTOR('',#32016,1000.);
#8360=VECTOR('',#32017,1000.);
#8361=VECTOR('',#32018,1000.);
#8362=VECTOR('',#32021,1000.);
#8363=VECTOR('',#32022,1000.);
#8364=VECTOR('',#32023,1000.);
#8365=VECTOR('',#32024,1000.);
#8366=VECTOR('',#32027,1000.);
#8367=VECTOR('',#32028,1000.);
#8368=VECTOR('',#32033,1000.);
#8369=VECTOR('',#32036,1000.);
#8370=VECTOR('',#32041,1000.);
#8371=VECTOR('',#32044,1000.);
#8372=VECTOR('',#32049,1000.);
#8373=VECTOR('',#32052,1000.);
#8374=VECTOR('',#32057,1000.);
#8375=VECTOR('',#32060,1000.);
#8376=VECTOR('',#32161,1000.);
#8377=VECTOR('',#32162,1000.);
#8378=VECTOR('',#32163,1000.);
#8379=VECTOR('',#32164,1000.);
#8380=VECTOR('',#32167,1000.);
#8381=VECTOR('',#32168,1000.);
#8382=VECTOR('',#32169,1000.);
#8383=VECTOR('',#32170,1000.);
#8384=VECTOR('',#32171,1000.);
#8385=VECTOR('',#32172,1000.);
#8386=VECTOR('',#32175,1000.);
#8387=VECTOR('',#32176,1000.);
#8388=VECTOR('',#32179,1000.);
#8389=VECTOR('',#32180,1000.);
#8390=VECTOR('',#32183,1000.);
#8391=VECTOR('',#32186,1000.);
#8392=VECTOR('',#32187,1000.);
#8393=VECTOR('',#32190,1000.);
#8394=VECTOR('',#32191,1000.);
#8395=VECTOR('',#32194,1000.);
#8396=VECTOR('',#32197,1000.);
#8397=VECTOR('',#32198,1000.);
#8398=VECTOR('',#32199,1000.);
#8399=VECTOR('',#32202,1000.);
#8400=VECTOR('',#32203,1000.);
#8401=VECTOR('',#32206,1000.);
#8402=VECTOR('',#32207,1000.);
#8403=VECTOR('',#32210,1000.);
#8404=VECTOR('',#32211,1000.);
#8405=VECTOR('',#32214,1000.);
#8406=VECTOR('',#32215,1000.);
#8407=VECTOR('',#32218,1000.);
#8408=VECTOR('',#32223,1000.);
#8409=VECTOR('',#32226,1000.);
#8410=VECTOR('',#32229,1000.);
#8411=VECTOR('',#32236,1000.);
#8412=VECTOR('',#32239,1000.);
#8413=VECTOR('',#32242,1000.);
#8414=VECTOR('',#32249,1000.);
#8415=VECTOR('',#32250,1000.);
#8416=VECTOR('',#32251,1000.);
#8417=VECTOR('',#32258,1000.);
#8418=VECTOR('',#32261,1000.);
#8419=VECTOR('',#32264,1000.);
#8420=VECTOR('',#32271,1000.);
#8421=VECTOR('',#32274,1000.);
#8422=VECTOR('',#32277,1000.);
#8423=VECTOR('',#32278,1000.);
#8424=VECTOR('',#32279,1000.);
#8425=VECTOR('',#32280,1000.);
#8426=VECTOR('',#32281,1000.);
#8427=VECTOR('',#32282,1000.);
#8428=VECTOR('',#32283,1000.);
#8429=VECTOR('',#32284,1000.);
#8430=VECTOR('',#32285,1000.);
#8431=VECTOR('',#32286,1000.);
#8432=VECTOR('',#32289,1000.);
#8433=VECTOR('',#32290,1000.);
#8434=VECTOR('',#32291,1000.);
#8435=VECTOR('',#32296,1000.);
#8436=VECTOR('',#32299,1000.);
#8437=VECTOR('',#32300,1000.);
#8438=VECTOR('',#32305,1000.);
#8439=VECTOR('',#32308,1000.);
#8440=VECTOR('',#32309,1000.);
#8441=VECTOR('',#32314,1000.);
#8442=VECTOR('',#32319,1000.);
#8443=VECTOR('',#32324,1000.);
#8444=VECTOR('',#32327,1000.);
#8445=VECTOR('',#32328,1000.);
#8446=VECTOR('',#32333,1000.);
#8447=VECTOR('',#32336,1000.);
#8448=VECTOR('',#32337,1000.);
#8449=VECTOR('',#32342,1000.);
#8450=VECTOR('',#32345,1000.);
#8451=VECTOR('',#32346,1000.);
#8452=VECTOR('',#32351,1000.);
#8453=VECTOR('',#32356,1000.);
#8454=VECTOR('',#32361,1000.);
#8455=VECTOR('',#32364,1000.);
#8456=VECTOR('',#32365,1000.);
#8457=VECTOR('',#32368,1000.);
#8458=VECTOR('',#32369,1000.);
#8459=VECTOR('',#32372,1000.);
#8460=VECTOR('',#32373,1000.);
#8461=VECTOR('',#32378,1000.);
#8462=VECTOR('',#32383,1000.);
#8463=VECTOR('',#32388,1000.);
#8464=VECTOR('',#32391,1000.);
#8465=VECTOR('',#32392,1000.);
#8466=VECTOR('',#32397,1000.);
#8467=VECTOR('',#32400,1000.);
#8468=VECTOR('',#32401,1000.);
#8469=VECTOR('',#32406,1000.);
#8470=VECTOR('',#32409,1000.);
#8471=VECTOR('',#32410,1000.);
#8472=VECTOR('',#32415,1000.);
#8473=VECTOR('',#32420,1000.);
#8474=VECTOR('',#32425,1000.);
#8475=VECTOR('',#32428,1000.);
#8476=VECTOR('',#32429,1000.);
#8477=VECTOR('',#32434,1000.);
#8478=VECTOR('',#32437,1000.);
#8479=VECTOR('',#32438,1000.);
#8480=VECTOR('',#32443,1000.);
#8481=VECTOR('',#32446,1000.);
#8482=VECTOR('',#32447,1000.);
#8483=VECTOR('',#32450,1000.);
#8484=VECTOR('',#32451,1000.);
#8485=VECTOR('',#32454,1000.);
#8486=VECTOR('',#32455,1000.);
#8487=VECTOR('',#32458,1000.);
#8488=VECTOR('',#32459,1000.);
#8489=VECTOR('',#32462,1000.);
#8490=VECTOR('',#32463,1000.);
#8491=VECTOR('',#32466,1000.);
#8492=VECTOR('',#32467,1000.);
#8493=VECTOR('',#32470,1000.);
#8494=VECTOR('',#32471,1000.);
#8495=VECTOR('',#32474,1000.);
#8496=VECTOR('',#32475,1000.);
#8497=VECTOR('',#32478,1000.);
#8498=VECTOR('',#32479,1000.);
#8499=VECTOR('',#32482,1000.);
#8500=VECTOR('',#32487,1000.);
#8501=VECTOR('',#32490,1000.);
#8502=VECTOR('',#32493,1000.);
#8503=VECTOR('',#32494,1000.);
#8504=VECTOR('',#32497,1000.);
#8505=VECTOR('',#32498,1000.);
#8506=VECTOR('',#32499,1000.);
#8507=VECTOR('',#32500,1000.);
#8508=VECTOR('',#32501,1000.);
#8509=VECTOR('',#32502,1000.);
#8510=VECTOR('',#32503,1000.);
#8511=VECTOR('',#32506,1000.);
#8512=VECTOR('',#32509,1000.);
#8513=VECTOR('',#32516,1000.);
#8514=VECTOR('',#32519,1000.);
#8515=VECTOR('',#32522,1000.);
#8516=VECTOR('',#32529,1000.);
#8517=VECTOR('',#32530,1000.);
#8518=VECTOR('',#32531,1000.);
#8519=VECTOR('',#32538,1000.);
#8520=VECTOR('',#32541,1000.);
#8521=VECTOR('',#32544,1000.);
#8522=VECTOR('',#32551,1000.);
#8523=VECTOR('',#32554,1000.);
#8524=VECTOR('',#32557,1000.);
#8525=VECTOR('',#32558,1000.);
#8526=VECTOR('',#32559,1000.);
#8527=VECTOR('',#32560,1000.);
#8528=VECTOR('',#32561,1000.);
#8529=VECTOR('',#32564,1000.);
#8530=VECTOR('',#32565,1000.);
#8531=VECTOR('',#32568,1000.);
#8532=VECTOR('',#32569,1000.);
#8533=VECTOR('',#32578,1000.);
#8534=VECTOR('',#32581,1000.);
#8535=VECTOR('',#32584,1000.);
#8536=VECTOR('',#32585,1000.);
#8537=VECTOR('',#32586,1000.);
#8538=VECTOR('',#32589,1000.);
#8539=VECTOR('',#32590,1000.);
#8540=VECTOR('',#32593,1000.);
#8541=VECTOR('',#32594,1000.);
#8542=VECTOR('',#32597,1000.);
#8543=VECTOR('',#32598,1000.);
#8544=VECTOR('',#32601,1000.);
#8545=VECTOR('',#32602,1000.);
#8546=VECTOR('',#32603,1000.);
#8547=VECTOR('',#32604,1000.);
#8548=VECTOR('',#32605,1000.);
#8549=VECTOR('',#32608,1000.);
#8550=VECTOR('',#32609,1000.);
#8551=VECTOR('',#32612,1000.);
#8552=VECTOR('',#32613,1000.);
#8553=VECTOR('',#32616,1000.);
#8554=VECTOR('',#32617,1000.);
#8555=VECTOR('',#32620,1000.);
#8556=VECTOR('',#32621,1000.);
#8557=VECTOR('',#32624,1000.);
#8558=VECTOR('',#32625,1000.);
#8559=VECTOR('',#32630,1000.);
#8560=VECTOR('',#32633,1000.);
#8561=VECTOR('',#32634,1000.);
#8562=VECTOR('',#32639,1000.);
#8563=VECTOR('',#32642,1000.);
#8564=VECTOR('',#32643,1000.);
#8565=VECTOR('',#32648,1000.);
#8566=VECTOR('',#32653,1000.);
#8567=VECTOR('',#32658,1000.);
#8568=VECTOR('',#32661,1000.);
#8569=VECTOR('',#32662,1000.);
#8570=VECTOR('',#32667,1000.);
#8571=VECTOR('',#32670,1000.);
#8572=VECTOR('',#32671,1000.);
#8573=VECTOR('',#32676,1000.);
#8574=VECTOR('',#32679,1000.);
#8575=VECTOR('',#32680,1000.);
#8576=VECTOR('',#32685,1000.);
#8577=VECTOR('',#32690,1000.);
#8578=VECTOR('',#32695,1000.);
#8579=VECTOR('',#32698,1000.);
#8580=VECTOR('',#32699,1000.);
#8581=VECTOR('',#32702,1000.);
#8582=VECTOR('',#32703,1000.);
#8583=VECTOR('',#32706,1000.);
#8584=VECTOR('',#32707,1000.);
#8585=VECTOR('',#32712,1000.);
#8586=VECTOR('',#32717,1000.);
#8587=VECTOR('',#32722,1000.);
#8588=VECTOR('',#32725,1000.);
#8589=VECTOR('',#32726,1000.);
#8590=VECTOR('',#32731,1000.);
#8591=VECTOR('',#32734,1000.);
#8592=VECTOR('',#32735,1000.);
#8593=VECTOR('',#32740,1000.);
#8594=VECTOR('',#32743,1000.);
#8595=VECTOR('',#32744,1000.);
#8596=VECTOR('',#32749,1000.);
#8597=VECTOR('',#32754,1000.);
#8598=VECTOR('',#32759,1000.);
#8599=VECTOR('',#32762,1000.);
#8600=VECTOR('',#32763,1000.);
#8601=VECTOR('',#32768,1000.);
#8602=VECTOR('',#32771,1000.);
#8603=VECTOR('',#32772,1000.);
#8604=VECTOR('',#32777,1000.);
#8605=VECTOR('',#32780,1000.);
#8606=VECTOR('',#32785,1000.);
#8607=VECTOR('',#32786,1000.);
#8608=VECTOR('',#32787,1000.);
#8609=VECTOR('',#32788,1000.);
#8610=VECTOR('',#32791,1000.);
#8611=VECTOR('',#32792,1000.);
#8612=VECTOR('',#32793,1000.);
#8613=VECTOR('',#32794,1000.);
#8614=VECTOR('',#32797,1000.);
#8615=VECTOR('',#32798,1000.);
#8616=VECTOR('',#32801,1000.);
#8617=VECTOR('',#32802,1000.);
#8618=VECTOR('',#32813,1000.);
#8619=VECTOR('',#32816,1000.);
#8620=VECTOR('',#32817,1000.);
#8621=VECTOR('',#32818,1000.);
#8622=VECTOR('',#32819,1000.);
#8623=VECTOR('',#32822,1000.);
#8624=VECTOR('',#32823,1000.);
#8625=VECTOR('',#32824,1000.);
#8626=VECTOR('',#32827,1000.);
#8627=VECTOR('',#32828,1000.);
#8628=VECTOR('',#32829,1000.);
#8629=VECTOR('',#32830,1000.);
#8630=VECTOR('',#32833,1000.);
#8631=VECTOR('',#32836,1000.);
#8632=VECTOR('',#32837,1000.);
#8633=VECTOR('',#32840,1000.);
#8634=VECTOR('',#32845,1000.);
#8635=VECTOR('',#32846,1000.);
#8636=VECTOR('',#32847,1000.);
#8637=VECTOR('',#32848,1000.);
#8638=VECTOR('',#32849,1000.);
#8639=VECTOR('',#32850,1000.);
#8640=VECTOR('',#32851,1000.);
#8641=VECTOR('',#32852,1000.);
#8642=VECTOR('',#32853,1000.);
#8643=VECTOR('',#32854,1000.);
#8644=VECTOR('',#32857,1000.);
#8645=VECTOR('',#32860,1000.);
#8646=VECTOR('',#32867,1000.);
#8647=VECTOR('',#32870,1000.);
#8648=VECTOR('',#32873,1000.);
#8649=VECTOR('',#32880,1000.);
#8650=VECTOR('',#32881,1000.);
#8651=VECTOR('',#32882,1000.);
#8652=VECTOR('',#32889,1000.);
#8653=VECTOR('',#32892,1000.);
#8654=VECTOR('',#32895,1000.);
#8655=VECTOR('',#32902,1000.);
#8656=VECTOR('',#32905,1000.);
#8657=VECTOR('',#32908,1000.);
#8658=VECTOR('',#32911,1000.);
#8659=VECTOR('',#32912,1000.);
#8660=VECTOR('',#32915,1000.);
#8661=VECTOR('',#32916,1000.);
#8662=VECTOR('',#32919,1000.);
#8663=VECTOR('',#32920,1000.);
#8664=VECTOR('',#32921,1000.);
#8665=VECTOR('',#32924,1000.);
#8666=VECTOR('',#32925,1000.);
#8667=VECTOR('',#32926,1000.);
#8668=VECTOR('',#32929,1000.);
#8669=VECTOR('',#32930,1000.);
#8670=VECTOR('',#32931,1000.);
#8671=VECTOR('',#32934,1000.);
#8672=VECTOR('',#32935,1000.);
#8673=VECTOR('',#32936,1000.);
#8674=VECTOR('',#32949,1000.);
#8675=VECTOR('',#32950,1000.);
#8676=VECTOR('',#32951,1000.);
#8677=VECTOR('',#32954,1000.);
#8678=VECTOR('',#32955,1000.);
#8679=VECTOR('',#32956,1000.);
#8680=VECTOR('',#32961,1000.);
#8681=VECTOR('',#32962,1000.);
#8682=VECTOR('',#32965,1000.);
#8683=VECTOR('',#32966,1000.);
#8684=VECTOR('',#32967,1000.);
#8685=VECTOR('',#32970,1000.);
#8686=VECTOR('',#32971,1000.);
#8687=VECTOR('',#32978,1000.);
#8688=VECTOR('',#32979,1000.);
#8689=VECTOR('',#32988,1000.);
#8690=VECTOR('',#32989,1000.);
#8691=VECTOR('',#32990,1000.);
#8692=VECTOR('',#32993,1000.);
#8693=VECTOR('',#32994,1000.);
#8694=VECTOR('',#32997,1000.);
#8695=VECTOR('',#32998,1000.);
#8696=VECTOR('',#33001,1000.);
#8697=VECTOR('',#33002,1000.);
#8698=VECTOR('',#33005,1000.);
#8699=VECTOR('',#33006,1000.);
#8700=VECTOR('',#33009,1000.);
#8701=VECTOR('',#33010,1000.);
#8702=VECTOR('',#33013,1000.);
#8703=VECTOR('',#33014,1000.);
#8704=VECTOR('',#33017,1000.);
#8705=VECTOR('',#33018,1000.);
#8706=VECTOR('',#33021,1000.);
#8707=VECTOR('',#33022,1000.);
#8708=VECTOR('',#33025,1000.);
#8709=VECTOR('',#33026,1000.);
#8710=VECTOR('',#33031,1000.);
#8711=VECTOR('',#33034,1000.);
#8712=VECTOR('',#33035,1000.);
#8713=VECTOR('',#33040,1000.);
#8714=VECTOR('',#33043,1000.);
#8715=VECTOR('',#33044,1000.);
#8716=VECTOR('',#33049,1000.);
#8717=VECTOR('',#33054,1000.);
#8718=VECTOR('',#33059,1000.);
#8719=VECTOR('',#33062,1000.);
#8720=VECTOR('',#33063,1000.);
#8721=VECTOR('',#33068,1000.);
#8722=VECTOR('',#33071,1000.);
#8723=VECTOR('',#33072,1000.);
#8724=VECTOR('',#33077,1000.);
#8725=VECTOR('',#33080,1000.);
#8726=VECTOR('',#33081,1000.);
#8727=VECTOR('',#33086,1000.);
#8728=VECTOR('',#33091,1000.);
#8729=VECTOR('',#33096,1000.);
#8730=VECTOR('',#33099,1000.);
#8731=VECTOR('',#33100,1000.);
#8732=VECTOR('',#33103,1000.);
#8733=VECTOR('',#33104,1000.);
#8734=VECTOR('',#33107,1000.);
#8735=VECTOR('',#33108,1000.);
#8736=VECTOR('',#33113,1000.);
#8737=VECTOR('',#33118,1000.);
#8738=VECTOR('',#33123,1000.);
#8739=VECTOR('',#33126,1000.);
#8740=VECTOR('',#33127,1000.);
#8741=VECTOR('',#33132,1000.);
#8742=VECTOR('',#33135,1000.);
#8743=VECTOR('',#33136,1000.);
#8744=VECTOR('',#33141,1000.);
#8745=VECTOR('',#33144,1000.);
#8746=VECTOR('',#33145,1000.);
#8747=VECTOR('',#33150,1000.);
#8748=VECTOR('',#33155,1000.);
#8749=VECTOR('',#33160,1000.);
#8750=VECTOR('',#33163,1000.);
#8751=VECTOR('',#33164,1000.);
#8752=VECTOR('',#33169,1000.);
#8753=VECTOR('',#33172,1000.);
#8754=VECTOR('',#33173,1000.);
#8755=VECTOR('',#33178,1000.);
#8756=VECTOR('',#33181,1000.);
#8757=VECTOR('',#33184,1000.);
#8758=VECTOR('',#33185,1000.);
#8759=VECTOR('',#33186,1000.);
#8760=VECTOR('',#33187,1000.);
#8761=VECTOR('',#33190,1000.);
#8762=VECTOR('',#33191,1000.);
#8763=VECTOR('',#33192,1000.);
#8764=VECTOR('',#33195,1000.);
#8765=VECTOR('',#33196,1000.);
#8766=VECTOR('',#33197,1000.);
#8767=VECTOR('',#33200,1000.);
#8768=VECTOR('',#33201,1000.);
#8769=VECTOR('',#33202,1000.);
#8770=VECTOR('',#33205,1000.);
#8771=VECTOR('',#33206,1000.);
#8772=VECTOR('',#33207,1000.);
#8773=VECTOR('',#33210,1000.);
#8774=VECTOR('',#33211,1000.);
#8775=VECTOR('',#33212,1000.);
#8776=VECTOR('',#33213,1000.);
#8777=VECTOR('',#33216,1000.);
#8778=VECTOR('',#33217,1000.);
#8779=VECTOR('',#33218,1000.);
#8780=VECTOR('',#33221,1000.);
#8781=VECTOR('',#33222,1000.);
#8782=VECTOR('',#33223,1000.);
#8783=VECTOR('',#33226,1000.);
#8784=VECTOR('',#33227,1000.);
#8785=VECTOR('',#33230,1000.);
#8786=VECTOR('',#33231,1000.);
#8787=VECTOR('',#33232,1000.);
#8788=VECTOR('',#33233,1000.);
#8789=VECTOR('',#33236,1000.);
#8790=VECTOR('',#33237,1000.);
#8791=VECTOR('',#33238,1000.);
#8792=VECTOR('',#33241,1000.);
#8793=VECTOR('',#33242,1000.);
#8794=VECTOR('',#33243,1000.);
#8795=VECTOR('',#33246,1000.);
#8796=VECTOR('',#33247,1000.);
#8797=VECTOR('',#33248,1000.);
#8798=VECTOR('',#33251,1000.);
#8799=VECTOR('',#33252,1000.);
#8800=VECTOR('',#33253,1000.);
#8801=VECTOR('',#33256,1000.);
#8802=VECTOR('',#33257,1000.);
#8803=VECTOR('',#33258,1000.);
#8804=VECTOR('',#33261,1000.);
#8805=VECTOR('',#33262,1000.);
#8806=VECTOR('',#33263,1000.);
#8807=VECTOR('',#33266,1000.);
#8808=VECTOR('',#33267,1000.);
#8809=VECTOR('',#33268,1000.);
#8810=VECTOR('',#33271,1000.);
#8811=VECTOR('',#33272,1000.);
#8812=VECTOR('',#33273,1000.);
#8813=VECTOR('',#33276,1000.);
#8814=VECTOR('',#33277,1000.);
#8815=VECTOR('',#33278,1000.);
#8816=VECTOR('',#33281,1000.);
#8817=VECTOR('',#33282,1000.);
#8818=VECTOR('',#33283,1000.);
#8819=VECTOR('',#33286,1000.);
#8820=VECTOR('',#33287,1000.);
#8821=VECTOR('',#33288,1000.);
#8822=VECTOR('',#33291,1000.);
#8823=VECTOR('',#33292,1000.);
#8824=VECTOR('',#33293,1000.);
#8825=VECTOR('',#33296,1000.);
#8826=VECTOR('',#33297,1000.);
#8827=VECTOR('',#33298,1000.);
#8828=VECTOR('',#33301,1000.);
#8829=VECTOR('',#33302,1000.);
#8830=VECTOR('',#33303,1000.);
#8831=VECTOR('',#33308,1000.);
#8832=VECTOR('',#33309,1000.);
#8833=VECTOR('',#33312,1000.);
#8834=VECTOR('',#33313,1000.);
#8835=VECTOR('',#33314,1000.);
#8836=VECTOR('',#33319,1000.);
#8837=VECTOR('',#33320,1000.);
#8838=VECTOR('',#33325,1000.);
#8839=VECTOR('',#33326,1000.);
#8840=VECTOR('',#33329,1000.);
#8841=VECTOR('',#33330,1000.);
#8842=VECTOR('',#33331,1000.);
#8843=VECTOR('',#33334,1000.);
#8844=VECTOR('',#33341,1000.);
#8845=VECTOR('',#33342,1000.);
#8846=VECTOR('',#33345,1000.);
#8847=VECTOR('',#33346,1000.);
#8848=VECTOR('',#33347,1000.);
#8849=VECTOR('',#33350,1000.);
#8850=VECTOR('',#33351,1000.);
#8851=VECTOR('',#33352,1000.);
#8852=VECTOR('',#33355,1000.);
#8853=VECTOR('',#33356,1000.);
#8854=VECTOR('',#33357,1000.);
#8855=VECTOR('',#33362,1000.);
#8856=VECTOR('',#33365,1000.);
#8857=VECTOR('',#33366,1000.);
#8858=VECTOR('',#33369,1000.);
#8859=VECTOR('',#33372,1000.);
#8860=VECTOR('',#33379,1000.);
#8861=VECTOR('',#33382,1000.);
#8862=VECTOR('',#33385,1000.);
#8863=VECTOR('',#33392,1000.);
#8864=VECTOR('',#33393,1000.);
#8865=VECTOR('',#33394,1000.);
#8866=VECTOR('',#33401,1000.);
#8867=VECTOR('',#33404,1000.);
#8868=VECTOR('',#33407,1000.);
#8869=VECTOR('',#33414,1000.);
#8870=VECTOR('',#33417,1000.);
#8871=VECTOR('',#33420,1000.);
#8872=VECTOR('',#33421,1000.);
#8873=VECTOR('',#33424,1000.);
#8874=VECTOR('',#33425,1000.);
#8875=VECTOR('',#33426,1000.);
#8876=VECTOR('',#33427,1000.);
#8877=VECTOR('',#33428,1000.);
#8878=VECTOR('',#33429,1000.);
#8879=VECTOR('',#33430,1000.);
#8880=VECTOR('',#33431,1000.);
#8881=VECTOR('',#33432,1000.);
#8882=VECTOR('',#33433,1000.);
#8883=VECTOR('',#33434,1000.);
#8884=VECTOR('',#33435,1000.);
#8885=VECTOR('',#33436,1000.);
#8886=VECTOR('',#33439,1000.);
#8887=VECTOR('',#33440,1000.);
#8888=VECTOR('',#33441,1000.);
#8889=VECTOR('',#33444,1000.);
#8890=VECTOR('',#33445,1000.);
#8891=VECTOR('',#33446,1000.);
#8892=VECTOR('',#33449,1000.);
#8893=VECTOR('',#33450,1000.);
#8894=VECTOR('',#33453,1000.);
#8895=VECTOR('',#33454,1000.);
#8896=VECTOR('',#33457,1000.);
#8897=VECTOR('',#33458,1000.);
#8898=VECTOR('',#33461,1000.);
#8899=VECTOR('',#33464,1000.);
#8900=VECTOR('',#33467,1000.);
#8901=VECTOR('',#33470,1000.);
#8902=VECTOR('',#33473,1000.);
#8903=VECTOR('',#33476,1000.);
#8904=VECTOR('',#33477,1000.);
#8905=VECTOR('',#33480,1000.);
#8906=VECTOR('',#33485,1000.);
#8907=VECTOR('',#33486,1000.);
#8908=VECTOR('',#33491,1000.);
#8909=VECTOR('',#33492,1000.);
#8910=VECTOR('',#33501,1000.);
#8911=VECTOR('',#33502,1000.);
#8912=VECTOR('',#33507,1000.);
#8913=VECTOR('',#33508,1000.);
#8914=VECTOR('',#33511,1000.);
#8915=VECTOR('',#33514,1000.);
#8916=VECTOR('',#33519,1000.);
#8917=VECTOR('',#33520,1000.);
#8918=VECTOR('',#33525,1000.);
#8919=VECTOR('',#33526,1000.);
#8920=VECTOR('',#33533,1000.);
#8921=VECTOR('',#33534,1000.);
#8922=VECTOR('',#33535,1000.);
#8923=VECTOR('',#33538,1000.);
#8924=VECTOR('',#33543,1000.);
#8925=VECTOR('',#33544,1000.);
#8926=VECTOR('',#33549,1000.);
#8927=VECTOR('',#33550,1000.);
#8928=VECTOR('',#33559,1000.);
#8929=VECTOR('',#33560,1000.);
#8930=VECTOR('',#33565,1000.);
#8931=VECTOR('',#33566,1000.);
#8932=VECTOR('',#33569,1000.);
#8933=VECTOR('',#33572,1000.);
#8934=VECTOR('',#33575,1000.);
#8935=VECTOR('',#33580,1000.);
#8936=VECTOR('',#33581,1000.);
#8937=VECTOR('',#33586,1000.);
#8938=VECTOR('',#33587,1000.);
#8939=VECTOR('',#33594,1000.);
#8940=VECTOR('',#33597,1000.);
#8941=VECTOR('',#33600,1000.);
#8942=VECTOR('',#33603,1000.);
#8943=VECTOR('',#33606,1000.);
#8944=VECTOR('',#33607,1000.);
#8945=VECTOR('',#33608,1000.);
#8946=VECTOR('',#33611,1000.);
#8947=VECTOR('',#33612,1000.);
#8948=VECTOR('',#33615,1000.);
#8949=VECTOR('',#33616,1000.);
#8950=VECTOR('',#33619,1000.);
#8951=VECTOR('',#33622,1000.);
#8952=VECTOR('',#33623,1000.);
#8953=VECTOR('',#33626,1000.);
#8954=VECTOR('',#33629,1000.);
#8955=VECTOR('',#33632,1000.);
#8956=VECTOR('',#33635,1000.);
#8957=VECTOR('',#33638,1000.);
#8958=VECTOR('',#33641,1000.);
#8959=VECTOR('',#33644,1000.);
#8960=VECTOR('',#33645,1000.);
#8961=VECTOR('',#33648,1000.);
#8962=VECTOR('',#33653,1000.);
#8963=VECTOR('',#33654,1000.);
#8964=VECTOR('',#33659,1000.);
#8965=VECTOR('',#33662,1000.);
#9916=CIRCLE('',#26509,2.5);
#9917=CIRCLE('',#26510,2.5);
#9918=CIRCLE('',#26512,2.5);
#9919=CIRCLE('',#26513,2.5);
#9920=CIRCLE('',#26515,3.65);
#9921=CIRCLE('',#26516,3.65);
#9922=CIRCLE('',#26520,3.3235);
#9923=CIRCLE('',#26521,3.3235);
#9924=CIRCLE('',#26523,3.3235);
#9925=CIRCLE('',#26524,3.3235);
#9926=CIRCLE('',#26526,3.3235);
#9927=CIRCLE('',#26527,3.32349999999999);
#9928=CIRCLE('',#26529,3.32349999999999);
#9929=CIRCLE('',#26530,3.3235);
#9930=CIRCLE('',#26532,2.5);
#9931=CIRCLE('',#26533,2.5);
#9932=CIRCLE('',#26535,2.5);
#9933=CIRCLE('',#26536,2.5);
#9934=CIRCLE('',#26538,3.65);
#9935=CIRCLE('',#26539,3.65);
#9936=CIRCLE('',#26541,0.500000000000004);
#9937=CIRCLE('',#26542,0.500000000000004);
#9938=CIRCLE('',#26543,0.500000000000006);
#9939=CIRCLE('',#26547,0.5);
#9940=CIRCLE('',#26548,0.5);
#9941=CIRCLE('',#26549,0.5);
#9942=CIRCLE('',#26550,4.);
#9943=CIRCLE('',#26551,4.);
#9944=CIRCLE('',#26553,4.);
#9945=CIRCLE('',#26555,4.99995);
#9946=CIRCLE('',#26556,4.99995);
#9947=CIRCLE('',#26585,2.3);
#9948=CIRCLE('',#26586,2.3);
#9949=CIRCLE('',#26588,2.3);
#9950=CIRCLE('',#26589,2.3);
#9951=CIRCLE('',#26591,2.3);
#9952=CIRCLE('',#26592,2.3);
#9953=CIRCLE('',#26594,2.3);
#9954=CIRCLE('',#26595,2.3);
#9955=CIRCLE('',#26597,0.5);
#9956=CIRCLE('',#26598,0.5);
#9957=CIRCLE('',#26600,0.5);
#9958=CIRCLE('',#26601,0.5);
#9959=CIRCLE('',#26603,0.5);
#9960=CIRCLE('',#26604,0.5);
#9961=CIRCLE('',#26606,0.5);
#9962=CIRCLE('',#26607,0.5);
#9963=CIRCLE('',#26609,0.5);
#9964=CIRCLE('',#26610,0.5);
#9965=CIRCLE('',#26612,0.5);
#9966=CIRCLE('',#26613,0.5);
#9967=CIRCLE('',#26615,0.5);
#9968=CIRCLE('',#26616,0.5);
#9969=CIRCLE('',#26618,0.5);
#9970=CIRCLE('',#26619,0.5);
#9971=CIRCLE('',#26621,0.5);
#9972=CIRCLE('',#26622,0.5);
#9973=CIRCLE('',#26624,0.5);
#9974=CIRCLE('',#26625,0.5);
#9975=CIRCLE('',#26627,0.5);
#9976=CIRCLE('',#26628,0.5);
#9977=CIRCLE('',#26630,0.499999999999999);
#9978=CIRCLE('',#26631,0.5);
#9979=CIRCLE('',#26633,0.5);
#9980=CIRCLE('',#26634,0.5);
#9981=CIRCLE('',#26636,0.5);
#9982=CIRCLE('',#26637,0.5);
#9983=CIRCLE('',#26639,0.5);
#9984=CIRCLE('',#26640,0.5);
#9985=CIRCLE('',#26642,0.500000000000001);
#9986=CIRCLE('',#26643,0.5);
#9987=CIRCLE('',#26661,0.450000000000001);
#9988=CIRCLE('',#26662,0.450000000000001);
#9989=CIRCLE('',#26663,0.55);
#9990=CIRCLE('',#26664,2.25);
#9991=CIRCLE('',#26665,0.549999999999998);
#9992=CIRCLE('',#26666,0.55);
#9993=CIRCLE('',#26667,0.55);
#9994=CIRCLE('',#26668,0.55);
#9995=CIRCLE('',#26669,2.25);
#9996=CIRCLE('',#26670,0.55);
#9997=CIRCLE('',#26671,0.550000000000001);
#9998=CIRCLE('',#26672,2.25);
#9999=CIRCLE('',#26673,0.550000000000002);
#10000=CIRCLE('',#26674,0.55);
#10001=CIRCLE('',#26675,0.55);
#10002=CIRCLE('',#26676,0.55);
#10003=CIRCLE('',#26677,2.25);
#10004=CIRCLE('',#26678,0.55);
#10005=CIRCLE('',#26679,0.450000000000001);
#10006=CIRCLE('',#26680,0.450000000000001);
#10007=CIRCLE('',#26683,0.450000000000001);
#10008=CIRCLE('',#26686,0.450000000000001);
#10009=CIRCLE('',#26689,0.55);
#10010=CIRCLE('',#26691,2.25);
#10011=CIRCLE('',#26693,0.549999999999998);
#10012=CIRCLE('',#26696,0.55);
#10013=CIRCLE('',#26699,0.55);
#10014=CIRCLE('',#26702,0.55);
#10015=CIRCLE('',#26704,2.25);
#10016=CIRCLE('',#26706,0.55);
#10017=CIRCLE('',#26711,0.550000000000001);
#10018=CIRCLE('',#26713,2.25);
#10019=CIRCLE('',#26715,0.550000000000002);
#10020=CIRCLE('',#26718,0.55);
#10021=CIRCLE('',#26721,0.55);
#10022=CIRCLE('',#26724,0.55);
#10023=CIRCLE('',#26726,2.25);
#10024=CIRCLE('',#26728,0.55);
#10025=CIRCLE('',#26731,0.450000000000001);
#10026=CIRCLE('',#26734,0.450000000000001);
#10027=CIRCLE('',#26747,0.5);
#10028=CIRCLE('',#26749,4.99995);
#10029=CIRCLE('',#26750,0.5);
#10030=CIRCLE('',#26751,0.5);
#10031=CIRCLE('',#26752,0.5);
#10032=CIRCLE('',#26753,2.3);
#10033=CIRCLE('',#26754,0.5);
#10034=CIRCLE('',#26755,0.5);
#10035=CIRCLE('',#26756,0.5);
#10036=CIRCLE('',#26757,0.5);
#10037=CIRCLE('',#26758,2.3);
#10038=CIRCLE('',#26759,0.5);
#10039=CIRCLE('',#26760,0.5);
#10040=CIRCLE('',#26761,2.3);
#10041=CIRCLE('',#26762,0.5);
#10042=CIRCLE('',#26763,0.5);
#10043=CIRCLE('',#26764,0.5);
#10044=CIRCLE('',#26765,0.5);
#10045=CIRCLE('',#26766,2.3);
#10046=CIRCLE('',#26767,0.5);
#10047=CIRCLE('',#26768,0.5);
#10048=CIRCLE('',#26769,0.5);
#10049=CIRCLE('',#26773,0.5);
#10050=CIRCLE('',#26776,0.500000000000006);
#10051=CIRCLE('',#26788,0.5);
#10052=CIRCLE('',#26791,0.5);
#10053=CIRCLE('',#26794,0.5);
#10054=CIRCLE('',#26796,2.3);
#10055=CIRCLE('',#26798,0.499999999999999);
#10056=CIRCLE('',#26801,0.5);
#10057=CIRCLE('',#26804,0.5);
#10058=CIRCLE('',#26807,0.5);
#10059=CIRCLE('',#26809,2.3);
#10060=CIRCLE('',#26811,0.500000000000001);
#10061=CIRCLE('',#26816,0.5);
#10062=CIRCLE('',#26818,2.3);
#10063=CIRCLE('',#26820,0.5);
#10064=CIRCLE('',#26823,0.5);
#10065=CIRCLE('',#26826,0.5);
#10066=CIRCLE('',#26829,0.5);
#10067=CIRCLE('',#26831,2.3);
#10068=CIRCLE('',#26833,0.5);
#10069=CIRCLE('',#26836,0.5);
#10070=CIRCLE('',#26839,0.5);
#10071=CIRCLE('',#26847,0.500000000000006);
#10072=CIRCLE('',#26849,2.);
#10073=CIRCLE('',#26850,2.);
#10074=CIRCLE('',#26855,2.);
#10075=CIRCLE('',#26857,2.);
#10076=CIRCLE('',#26859,0.450000000000001);
#10077=CIRCLE('',#26860,0.450000000000001);
#10078=CIRCLE('',#26861,0.55);
#10079=CIRCLE('',#26862,2.25);
#10080=CIRCLE('',#26863,0.55);
#10081=CIRCLE('',#26864,0.55);
#10082=CIRCLE('',#26865,0.55);
#10083=CIRCLE('',#26866,0.550000000000002);
#10084=CIRCLE('',#26867,2.25);
#10085=CIRCLE('',#26868,0.550000000000001);
#10086=CIRCLE('',#26869,0.55);
#10087=CIRCLE('',#26870,2.25);
#10088=CIRCLE('',#26871,0.55);
#10089=CIRCLE('',#26872,0.55);
#10090=CIRCLE('',#26873,0.55);
#10091=CIRCLE('',#26874,0.549999999999998);
#10092=CIRCLE('',#26875,2.25);
#10093=CIRCLE('',#26876,0.55);
#10094=CIRCLE('',#26877,0.450000000000001);
#10095=CIRCLE('',#26878,0.450000000000001);
#10096=CIRCLE('',#26890,5.5);
#10097=CIRCLE('',#26896,5.5);
#10098=CIRCLE('',#26913,0.450000000000001);
#10099=CIRCLE('',#26916,0.450000000000001);
#10100=CIRCLE('',#26919,0.55);
#10101=CIRCLE('',#26921,2.25);
#10102=CIRCLE('',#26923,0.55);
#10103=CIRCLE('',#26926,0.55);
#10104=CIRCLE('',#26929,0.55);
#10105=CIRCLE('',#26932,0.550000000000002);
#10106=CIRCLE('',#26934,2.25);
#10107=CIRCLE('',#26936,0.550000000000001);
#10108=CIRCLE('',#26941,0.55);
#10109=CIRCLE('',#26943,2.25);
#10110=CIRCLE('',#26945,0.55);
#10111=CIRCLE('',#26948,0.55);
#10112=CIRCLE('',#26951,0.55);
#10113=CIRCLE('',#26954,0.549999999999998);
#10114=CIRCLE('',#26956,2.25);
#10115=CIRCLE('',#26958,0.55);
#10116=CIRCLE('',#26961,0.450000000000001);
#10117=CIRCLE('',#26964,0.450000000000001);
#10118=CIRCLE('',#26991,5.50000000000001);
#10119=CIRCLE('',#26999,5.49999999999999);
#10120=CIRCLE('',#27008,0.5);
#10121=CIRCLE('',#27009,0.5);
#10122=CIRCLE('',#27010,0.5);
#10123=CIRCLE('',#27011,2.3);
#10124=CIRCLE('',#27012,0.499999999999999);
#10125=CIRCLE('',#27013,0.5);
#10126=CIRCLE('',#27014,0.5);
#10127=CIRCLE('',#27015,0.5);
#10128=CIRCLE('',#27016,2.3);
#10129=CIRCLE('',#27017,0.500000000000001);
#10130=CIRCLE('',#27018,0.5);
#10131=CIRCLE('',#27019,2.3);
#10132=CIRCLE('',#27020,0.5);
#10133=CIRCLE('',#27021,0.5);
#10134=CIRCLE('',#27022,0.5);
#10135=CIRCLE('',#27023,0.5);
#10136=CIRCLE('',#27024,2.3);
#10137=CIRCLE('',#27025,0.5);
#10138=CIRCLE('',#27026,0.5);
#10139=CIRCLE('',#27027,0.5);
#10140=CIRCLE('',#27035,0.5);
#10141=CIRCLE('',#27037,0.5);
#10142=CIRCLE('',#27042,0.5);
#10143=CIRCLE('',#27044,0.5);
#10144=CIRCLE('',#27046,2.3);
#10145=CIRCLE('',#27048,0.5);
#10146=CIRCLE('',#27050,0.5);
#10147=CIRCLE('',#27054,0.5);
#10148=CIRCLE('',#27056,0.5);
#10149=CIRCLE('',#27058,2.3);
#10150=CIRCLE('',#27062,0.500000000000001);
#10151=CIRCLE('',#27064,0.5);
#10152=CIRCLE('',#27066,2.3);
#10153=CIRCLE('',#27068,0.5);
#10154=CIRCLE('',#27070,0.5);
#10155=CIRCLE('',#27075,0.499999999999999);
#10156=CIRCLE('',#27077,0.5);
#10157=CIRCLE('',#27079,2.3);
#10158=CIRCLE('',#27081,0.5);
#10159=CIRCLE('',#27083,0.5);
#10160=CIRCLE('',#27100,4.99995);
#11629=VERTEX_POINT('',#54038);
#11630=VERTEX_POINT('',#54040);
#11631=VERTEX_POINT('',#54044);
#11632=VERTEX_POINT('',#54046);
#11633=VERTEX_POINT('',#54050);
#11634=VERTEX_POINT('',#54052);
#11635=VERTEX_POINT('',#54056);
#11636=VERTEX_POINT('',#54059);
#11637=VERTEX_POINT('',#54062);
#11638=VERTEX_POINT('',#54064);
#11639=VERTEX_POINT('',#54068);
#11640=VERTEX_POINT('',#54070);
#11641=VERTEX_POINT('',#54074);
#11642=VERTEX_POINT('',#54076);
#11643=VERTEX_POINT('',#54080);
#11644=VERTEX_POINT('',#54082);
#11645=VERTEX_POINT('',#54086);
#11646=VERTEX_POINT('',#54088);
#11647=VERTEX_POINT('',#54092);
#11648=VERTEX_POINT('',#54094);
#11649=VERTEX_POINT('',#54098);
#11650=VERTEX_POINT('',#54100);
#11651=VERTEX_POINT('',#54104);
#11652=VERTEX_POINT('',#54106);
#11653=VERTEX_POINT('',#54108);
#11654=VERTEX_POINT('',#54110);
#11655=VERTEX_POINT('',#54112);
#11656=VERTEX_POINT('',#54116);
#11657=VERTEX_POINT('',#54119);
#11658=VERTEX_POINT('',#54122);
#11659=VERTEX_POINT('',#54124);
#11660=VERTEX_POINT('',#54126);
#11661=VERTEX_POINT('',#54128);
#11662=VERTEX_POINT('',#54130);
#11663=VERTEX_POINT('',#54160);
#11664=VERTEX_POINT('',#54161);
#11665=VERTEX_POINT('',#54172);
#11666=VERTEX_POINT('',#54183);
#11667=VERTEX_POINT('',#54194);
#11668=VERTEX_POINT('',#54198);
#11669=VERTEX_POINT('',#54201);
#11670=VERTEX_POINT('',#54212);
#11671=VERTEX_POINT('',#54234);
#11672=VERTEX_POINT('',#54238);
#11673=VERTEX_POINT('',#54240);
#11674=VERTEX_POINT('',#54244);
#11675=VERTEX_POINT('',#54245);
#11676=VERTEX_POINT('',#54247);
#11677=VERTEX_POINT('',#54249);
#11678=VERTEX_POINT('',#54253);
#11679=VERTEX_POINT('',#54255);
#11680=VERTEX_POINT('',#54257);
#11681=VERTEX_POINT('',#54261);
#11682=VERTEX_POINT('',#54262);
#11683=VERTEX_POINT('',#54264);
#11684=VERTEX_POINT('',#54266);
#11685=VERTEX_POINT('',#54270);
#11686=VERTEX_POINT('',#54272);
#11687=VERTEX_POINT('',#54274);
#11688=VERTEX_POINT('',#54278);
#11689=VERTEX_POINT('',#54279);
#11690=VERTEX_POINT('',#54281);
#11691=VERTEX_POINT('',#54283);
#11692=VERTEX_POINT('',#54287);
#11693=VERTEX_POINT('',#54288);
#11694=VERTEX_POINT('',#54290);
#11695=VERTEX_POINT('',#54292);
#11696=VERTEX_POINT('',#54296);
#11697=VERTEX_POINT('',#54297);
#11698=VERTEX_POINT('',#54299);
#11699=VERTEX_POINT('',#54301);
#11700=VERTEX_POINT('',#54305);
#11701=VERTEX_POINT('',#54306);
#11702=VERTEX_POINT('',#54308);
#11703=VERTEX_POINT('',#54310);
#11704=VERTEX_POINT('',#54314);
#11705=VERTEX_POINT('',#54315);
#11706=VERTEX_POINT('',#54317);
#11707=VERTEX_POINT('',#54319);
#11708=VERTEX_POINT('',#54323);
#11709=VERTEX_POINT('',#54324);
#11710=VERTEX_POINT('',#54326);
#11711=VERTEX_POINT('',#54328);
#11712=VERTEX_POINT('',#54332);
#11713=VERTEX_POINT('',#54333);
#11714=VERTEX_POINT('',#54335);
#11715=VERTEX_POINT('',#54337);
#11716=VERTEX_POINT('',#54341);
#11717=VERTEX_POINT('',#54342);
#11718=VERTEX_POINT('',#54344);
#11719=VERTEX_POINT('',#54346);
#11720=VERTEX_POINT('',#54350);
#11721=VERTEX_POINT('',#54351);
#11722=VERTEX_POINT('',#54353);
#11723=VERTEX_POINT('',#54355);
#11724=VERTEX_POINT('',#54359);
#11725=VERTEX_POINT('',#54361);
#11726=VERTEX_POINT('',#54365);
#11727=VERTEX_POINT('',#54366);
#11728=VERTEX_POINT('',#54368);
#11729=VERTEX_POINT('',#54370);
#11730=VERTEX_POINT('',#54374);
#11731=VERTEX_POINT('',#54376);
#11732=VERTEX_POINT('',#54380);
#11733=VERTEX_POINT('',#54381);
#11734=VERTEX_POINT('',#54383);
#11735=VERTEX_POINT('',#54385);
#11736=VERTEX_POINT('',#54389);
#11737=VERTEX_POINT('',#54390);
#11738=VERTEX_POINT('',#54392);
#11739=VERTEX_POINT('',#54394);
#11740=VERTEX_POINT('',#54398);
#11741=VERTEX_POINT('',#54399);
#11742=VERTEX_POINT('',#54401);
#11743=VERTEX_POINT('',#54403);
#11744=VERTEX_POINT('',#54407);
#11745=VERTEX_POINT('',#54408);
#11746=VERTEX_POINT('',#54410);
#11747=VERTEX_POINT('',#54412);
#11748=VERTEX_POINT('',#54419);
#11749=VERTEX_POINT('',#54420);
#11750=VERTEX_POINT('',#54422);
#11751=VERTEX_POINT('',#54424);
#11752=VERTEX_POINT('',#54428);
#11753=VERTEX_POINT('',#54429);
#11754=VERTEX_POINT('',#54431);
#11755=VERTEX_POINT('',#54433);
#11756=VERTEX_POINT('',#54437);
#11757=VERTEX_POINT('',#54438);
#11758=VERTEX_POINT('',#54440);
#11759=VERTEX_POINT('',#54442);
#11760=VERTEX_POINT('',#54446);
#11761=VERTEX_POINT('',#54447);
#11762=VERTEX_POINT('',#54449);
#11763=VERTEX_POINT('',#54451);
#11764=VERTEX_POINT('',#54504);
#11765=VERTEX_POINT('',#54505);
#11766=VERTEX_POINT('',#54507);
#11767=VERTEX_POINT('',#54509);
#11768=VERTEX_POINT('',#54513);
#11769=VERTEX_POINT('',#54515);
#11770=VERTEX_POINT('',#54518);
#11771=VERTEX_POINT('',#54520);
#11772=VERTEX_POINT('',#54524);
#11773=VERTEX_POINT('',#54528);
#11774=VERTEX_POINT('',#54534);
#11775=VERTEX_POINT('',#54538);
#11776=VERTEX_POINT('',#54544);
#11777=VERTEX_POINT('',#54546);
#11778=VERTEX_POINT('',#54550);
#11779=VERTEX_POINT('',#54554);
#11780=VERTEX_POINT('',#54558);
#11781=VERTEX_POINT('',#54562);
#11782=VERTEX_POINT('',#54569);
#11783=VERTEX_POINT('',#54570);
#11784=VERTEX_POINT('',#54572);
#11785=VERTEX_POINT('',#54574);
#11786=VERTEX_POINT('',#54576);
#11787=VERTEX_POINT('',#54578);
#11788=VERTEX_POINT('',#54580);
#11789=VERTEX_POINT('',#54582);
#11790=VERTEX_POINT('',#54584);
#11791=VERTEX_POINT('',#54586);
#11792=VERTEX_POINT('',#54588);
#11793=VERTEX_POINT('',#54590);
#11794=VERTEX_POINT('',#54592);
#11795=VERTEX_POINT('',#54594);
#11796=VERTEX_POINT('',#54596);
#11797=VERTEX_POINT('',#54598);
#11798=VERTEX_POINT('',#54600);
#11799=VERTEX_POINT('',#54602);
#11800=VERTEX_POINT('',#54604);
#11801=VERTEX_POINT('',#54606);
#11802=VERTEX_POINT('',#54608);
#11803=VERTEX_POINT('',#54610);
#11804=VERTEX_POINT('',#54612);
#11805=VERTEX_POINT('',#54614);
#11806=VERTEX_POINT('',#54616);
#11807=VERTEX_POINT('',#54618);
#11808=VERTEX_POINT('',#54620);
#11809=VERTEX_POINT('',#54622);
#11810=VERTEX_POINT('',#54624);
#11811=VERTEX_POINT('',#54626);
#11812=VERTEX_POINT('',#54628);
#11813=VERTEX_POINT('',#54630);
#11814=VERTEX_POINT('',#54632);
#11815=VERTEX_POINT('',#54634);
#11816=VERTEX_POINT('',#54636);
#11817=VERTEX_POINT('',#54638);
#11818=VERTEX_POINT('',#54640);
#11819=VERTEX_POINT('',#54642);
#11820=VERTEX_POINT('',#54644);
#11821=VERTEX_POINT('',#54646);
#11822=VERTEX_POINT('',#54648);
#11823=VERTEX_POINT('',#54650);
#11824=VERTEX_POINT('',#54652);
#11825=VERTEX_POINT('',#54654);
#11826=VERTEX_POINT('',#54658);
#11827=VERTEX_POINT('',#54659);
#11828=VERTEX_POINT('',#54664);
#11829=VERTEX_POINT('',#54668);
#11830=VERTEX_POINT('',#54672);
#11831=VERTEX_POINT('',#54676);
#11832=VERTEX_POINT('',#54680);
#11833=VERTEX_POINT('',#54684);
#11834=VERTEX_POINT('',#54688);
#11835=VERTEX_POINT('',#54692);
#11836=VERTEX_POINT('',#54696);
#11837=VERTEX_POINT('',#54700);
#11838=VERTEX_POINT('',#54704);
#11839=VERTEX_POINT('',#54708);
#11840=VERTEX_POINT('',#54712);
#11841=VERTEX_POINT('',#54716);
#11842=VERTEX_POINT('',#54720);
#11843=VERTEX_POINT('',#54724);
#11844=VERTEX_POINT('',#54728);
#11845=VERTEX_POINT('',#54732);
#11846=VERTEX_POINT('',#54736);
#11847=VERTEX_POINT('',#54740);
#11848=VERTEX_POINT('',#54744);
#11849=VERTEX_POINT('',#54748);
#11850=VERTEX_POINT('',#54752);
#11851=VERTEX_POINT('',#54756);
#11852=VERTEX_POINT('',#54760);
#11853=VERTEX_POINT('',#54764);
#11854=VERTEX_POINT('',#54768);
#11855=VERTEX_POINT('',#54772);
#11856=VERTEX_POINT('',#54776);
#11857=VERTEX_POINT('',#54780);
#11858=VERTEX_POINT('',#54784);
#11859=VERTEX_POINT('',#54788);
#11860=VERTEX_POINT('',#54792);
#11861=VERTEX_POINT('',#54796);
#11862=VERTEX_POINT('',#54800);
#11863=VERTEX_POINT('',#54804);
#11864=VERTEX_POINT('',#54808);
#11865=VERTEX_POINT('',#54812);
#11866=VERTEX_POINT('',#54816);
#11867=VERTEX_POINT('',#54820);
#11868=VERTEX_POINT('',#54824);
#11869=VERTEX_POINT('',#54828);
#11870=VERTEX_POINT('',#54835);
#11871=VERTEX_POINT('',#54837);
#11872=VERTEX_POINT('',#54841);
#11873=VERTEX_POINT('',#54842);
#11874=VERTEX_POINT('',#54844);
#11875=VERTEX_POINT('',#54846);
#11876=VERTEX_POINT('',#54848);
#11877=VERTEX_POINT('',#54850);
#11878=VERTEX_POINT('',#54852);
#11879=VERTEX_POINT('',#54854);
#11880=VERTEX_POINT('',#54856);
#11881=VERTEX_POINT('',#54858);
#11882=VERTEX_POINT('',#54860);
#11883=VERTEX_POINT('',#54862);
#11884=VERTEX_POINT('',#54864);
#11885=VERTEX_POINT('',#54866);
#11886=VERTEX_POINT('',#54868);
#11887=VERTEX_POINT('',#54870);
#11888=VERTEX_POINT('',#54872);
#11889=VERTEX_POINT('',#54874);
#11890=VERTEX_POINT('',#54876);
#11891=VERTEX_POINT('',#54878);
#11892=VERTEX_POINT('',#54880);
#11893=VERTEX_POINT('',#54882);
#11894=VERTEX_POINT('',#54884);
#11895=VERTEX_POINT('',#54886);
#11896=VERTEX_POINT('',#54888);
#11897=VERTEX_POINT('',#54890);
#11898=VERTEX_POINT('',#54892);
#11899=VERTEX_POINT('',#54894);
#11900=VERTEX_POINT('',#54896);
#11901=VERTEX_POINT('',#54898);
#11902=VERTEX_POINT('',#54900);
#11903=VERTEX_POINT('',#54902);
#11904=VERTEX_POINT('',#54904);
#11905=VERTEX_POINT('',#54906);
#11906=VERTEX_POINT('',#54908);
#11907=VERTEX_POINT('',#54910);
#11908=VERTEX_POINT('',#54912);
#11909=VERTEX_POINT('',#54914);
#11910=VERTEX_POINT('',#54916);
#11911=VERTEX_POINT('',#54918);
#11912=VERTEX_POINT('',#54920);
#11913=VERTEX_POINT('',#54922);
#11914=VERTEX_POINT('',#54924);
#11915=VERTEX_POINT('',#54926);
#11916=VERTEX_POINT('',#54928);
#11917=VERTEX_POINT('',#54930);
#11918=VERTEX_POINT('',#54932);
#11919=VERTEX_POINT('',#54934);
#11920=VERTEX_POINT('',#54938);
#11921=VERTEX_POINT('',#54942);
#11922=VERTEX_POINT('',#54949);
#11923=VERTEX_POINT('',#54951);
#11924=VERTEX_POINT('',#54955);
#11925=VERTEX_POINT('',#54956);
#11926=VERTEX_POINT('',#54961);
#11927=VERTEX_POINT('',#54965);
#11928=VERTEX_POINT('',#54969);
#11929=VERTEX_POINT('',#54973);
#11930=VERTEX_POINT('',#54974);
#11931=VERTEX_POINT('',#54977);
#11932=VERTEX_POINT('',#54982);
#11933=VERTEX_POINT('',#54986);
#11934=VERTEX_POINT('',#54990);
#11935=VERTEX_POINT('',#54994);
#11936=VERTEX_POINT('',#54998);
#11937=VERTEX_POINT('',#55002);
#11938=VERTEX_POINT('',#55006);
#11939=VERTEX_POINT('',#55010);
#11940=VERTEX_POINT('',#55014);
#11941=VERTEX_POINT('',#55018);
#11942=VERTEX_POINT('',#55022);
#11943=VERTEX_POINT('',#55026);
#11944=VERTEX_POINT('',#55030);
#11945=VERTEX_POINT('',#55034);
#11946=VERTEX_POINT('',#55038);
#11947=VERTEX_POINT('',#55042);
#11948=VERTEX_POINT('',#55046);
#11949=VERTEX_POINT('',#55050);
#11950=VERTEX_POINT('',#55054);
#11951=VERTEX_POINT('',#55058);
#11952=VERTEX_POINT('',#55062);
#11953=VERTEX_POINT('',#55066);
#11954=VERTEX_POINT('',#55070);
#11955=VERTEX_POINT('',#55074);
#11956=VERTEX_POINT('',#55078);
#11957=VERTEX_POINT('',#55082);
#11958=VERTEX_POINT('',#55086);
#11959=VERTEX_POINT('',#55090);
#11960=VERTEX_POINT('',#55094);
#11961=VERTEX_POINT('',#55098);
#11962=VERTEX_POINT('',#55102);
#11963=VERTEX_POINT('',#55106);
#11964=VERTEX_POINT('',#55110);
#11965=VERTEX_POINT('',#55114);
#11966=VERTEX_POINT('',#55118);
#11967=VERTEX_POINT('',#55122);
#11968=VERTEX_POINT('',#55126);
#11969=VERTEX_POINT('',#55130);
#11970=VERTEX_POINT('',#55137);
#11971=VERTEX_POINT('',#55138);
#11972=VERTEX_POINT('',#55140);
#11973=VERTEX_POINT('',#55142);
#11974=VERTEX_POINT('',#55146);
#11975=VERTEX_POINT('',#55147);
#11976=VERTEX_POINT('',#55149);
#11977=VERTEX_POINT('',#55151);
#11978=VERTEX_POINT('',#55155);
#11979=VERTEX_POINT('',#55159);
#11980=VERTEX_POINT('',#55165);
#11981=VERTEX_POINT('',#55167);
#11982=VERTEX_POINT('',#55171);
#11983=VERTEX_POINT('',#55173);
#11984=VERTEX_POINT('',#55175);
#11985=VERTEX_POINT('',#55179);
#11986=VERTEX_POINT('',#55181);
#11987=VERTEX_POINT('',#55185);
#11988=VERTEX_POINT('',#55186);
#11989=VERTEX_POINT('',#55188);
#11990=VERTEX_POINT('',#55190);
#11991=VERTEX_POINT('',#55194);
#11992=VERTEX_POINT('',#55197);
#11993=VERTEX_POINT('',#55201);
#11994=VERTEX_POINT('',#55205);
#11995=VERTEX_POINT('',#55206);
#11996=VERTEX_POINT('',#55208);
#11997=VERTEX_POINT('',#55210);
#11998=VERTEX_POINT('',#55212);
#11999=VERTEX_POINT('',#55214);
#12000=VERTEX_POINT('',#55216);
#12001=VERTEX_POINT('',#55218);
#12002=VERTEX_POINT('',#55220);
#12003=VERTEX_POINT('',#55222);
#12004=VERTEX_POINT('',#55224);
#12005=VERTEX_POINT('',#55226);
#12006=VERTEX_POINT('',#55228);
#12007=VERTEX_POINT('',#55230);
#12008=VERTEX_POINT('',#55232);
#12009=VERTEX_POINT('',#55234);
#12010=VERTEX_POINT('',#55236);
#12011=VERTEX_POINT('',#55238);
#12012=VERTEX_POINT('',#55240);
#12013=VERTEX_POINT('',#55242);
#12014=VERTEX_POINT('',#55244);
#12015=VERTEX_POINT('',#55246);
#12016=VERTEX_POINT('',#55248);
#12017=VERTEX_POINT('',#55250);
#12018=VERTEX_POINT('',#55252);
#12019=VERTEX_POINT('',#55254);
#12020=VERTEX_POINT('',#55256);
#12021=VERTEX_POINT('',#55258);
#12022=VERTEX_POINT('',#55260);
#12023=VERTEX_POINT('',#55262);
#12024=VERTEX_POINT('',#55264);
#12025=VERTEX_POINT('',#55266);
#12026=VERTEX_POINT('',#55268);
#12027=VERTEX_POINT('',#55270);
#12028=VERTEX_POINT('',#55272);
#12029=VERTEX_POINT('',#55274);
#12030=VERTEX_POINT('',#55276);
#12031=VERTEX_POINT('',#55278);
#12032=VERTEX_POINT('',#55280);
#12033=VERTEX_POINT('',#55282);
#12034=VERTEX_POINT('',#55284);
#12035=VERTEX_POINT('',#55286);
#12036=VERTEX_POINT('',#55288);
#12037=VERTEX_POINT('',#55290);
#12038=VERTEX_POINT('',#55294);
#12039=VERTEX_POINT('',#55298);
#12040=VERTEX_POINT('',#55302);
#12041=VERTEX_POINT('',#55303);
#12042=VERTEX_POINT('',#55308);
#12043=VERTEX_POINT('',#55310);
#12044=VERTEX_POINT('',#55314);
#12045=VERTEX_POINT('',#55316);
#12046=VERTEX_POINT('',#55320);
#12047=VERTEX_POINT('',#55322);
#12048=VERTEX_POINT('',#55330);
#12049=VERTEX_POINT('',#55332);
#12050=VERTEX_POINT('',#55334);
#12051=VERTEX_POINT('',#55338);
#12052=VERTEX_POINT('',#55339);
#12053=VERTEX_POINT('',#55344);
#12054=VERTEX_POINT('',#55346);
#12055=VERTEX_POINT('',#55350);
#12056=VERTEX_POINT('',#55351);
#12057=VERTEX_POINT('',#55356);
#12058=VERTEX_POINT('',#55361);
#12059=VERTEX_POINT('',#55363);
#12060=VERTEX_POINT('',#55370);
#12061=VERTEX_POINT('',#55371);
#12062=VERTEX_POINT('',#55376);
#12063=VERTEX_POINT('',#55380);
#12064=VERTEX_POINT('',#55384);
#12065=VERTEX_POINT('',#55388);
#12066=VERTEX_POINT('',#55392);
#12067=VERTEX_POINT('',#55396);
#12068=VERTEX_POINT('',#55400);
#12069=VERTEX_POINT('',#55404);
#12070=VERTEX_POINT('',#55408);
#12071=VERTEX_POINT('',#55412);
#12072=VERTEX_POINT('',#55416);
#12073=VERTEX_POINT('',#55420);
#12074=VERTEX_POINT('',#55424);
#12075=VERTEX_POINT('',#55428);
#12076=VERTEX_POINT('',#55432);
#12077=VERTEX_POINT('',#55436);
#12078=VERTEX_POINT('',#55440);
#12079=VERTEX_POINT('',#55444);
#12080=VERTEX_POINT('',#55448);
#12081=VERTEX_POINT('',#55452);
#12082=VERTEX_POINT('',#55456);
#12083=VERTEX_POINT('',#55460);
#12084=VERTEX_POINT('',#55464);
#12085=VERTEX_POINT('',#55468);
#12086=VERTEX_POINT('',#55472);
#12087=VERTEX_POINT('',#55476);
#12088=VERTEX_POINT('',#55480);
#12089=VERTEX_POINT('',#55484);
#12090=VERTEX_POINT('',#55488);
#12091=VERTEX_POINT('',#55492);
#12092=VERTEX_POINT('',#55496);
#12093=VERTEX_POINT('',#55500);
#12094=VERTEX_POINT('',#55504);
#12095=VERTEX_POINT('',#55508);
#12096=VERTEX_POINT('',#55512);
#12097=VERTEX_POINT('',#55516);
#12098=VERTEX_POINT('',#55520);
#12099=VERTEX_POINT('',#55524);
#12100=VERTEX_POINT('',#55528);
#12101=VERTEX_POINT('',#55532);
#12102=VERTEX_POINT('',#55536);
#12103=VERTEX_POINT('',#55540);
#12104=VERTEX_POINT('',#55546);
#12105=VERTEX_POINT('',#55547);
#12106=VERTEX_POINT('',#55549);
#12107=VERTEX_POINT('',#55551);
#12108=VERTEX_POINT('',#55555);
#12109=VERTEX_POINT('',#55557);
#12110=VERTEX_POINT('',#55561);
#12111=VERTEX_POINT('',#55563);
#12112=VERTEX_POINT('',#55567);
#12113=VERTEX_POINT('',#55569);
#12114=VERTEX_POINT('',#55573);
#12115=VERTEX_POINT('',#55575);
#12116=VERTEX_POINT('',#55579);
#12117=VERTEX_POINT('',#55580);
#12118=VERTEX_POINT('',#55582);
#12119=VERTEX_POINT('',#55584);
#12120=VERTEX_POINT('',#55588);
#12121=VERTEX_POINT('',#55590);
#12122=VERTEX_POINT('',#55594);
#12123=VERTEX_POINT('',#55596);
#12124=VERTEX_POINT('',#55603);
#12125=VERTEX_POINT('',#55605);
#12126=VERTEX_POINT('',#55607);
#12127=VERTEX_POINT('',#55611);
#12128=VERTEX_POINT('',#55613);
#12129=VERTEX_POINT('',#55617);
#12130=VERTEX_POINT('',#55618);
#12131=VERTEX_POINT('',#55623);
#12132=VERTEX_POINT('',#55624);
#12133=VERTEX_POINT('',#55629);
#12134=VERTEX_POINT('',#55630);
#12135=VERTEX_POINT('',#55635);
#12136=VERTEX_POINT('',#55636);
#12137=VERTEX_POINT('',#55641);
#12138=VERTEX_POINT('',#55643);
#12139=VERTEX_POINT('',#55647);
#12140=VERTEX_POINT('',#55648);
#12141=VERTEX_POINT('',#55653);
#12142=VERTEX_POINT('',#55654);
#12143=VERTEX_POINT('',#55659);
#12144=VERTEX_POINT('',#55660);
#12145=VERTEX_POINT('',#55665);
#12146=VERTEX_POINT('',#55667);
#12147=VERTEX_POINT('',#55671);
#12148=VERTEX_POINT('',#55673);
#12149=VERTEX_POINT('',#55677);
#12150=VERTEX_POINT('',#55679);
#12151=VERTEX_POINT('',#55683);
#12152=VERTEX_POINT('',#55685);
#12153=VERTEX_POINT('',#55689);
#12154=VERTEX_POINT('',#55694);
#12155=VERTEX_POINT('',#55696);
#12156=VERTEX_POINT('',#55700);
#12157=VERTEX_POINT('',#55701);
#12158=VERTEX_POINT('',#55706);
#12159=VERTEX_POINT('',#55708);
#12160=VERTEX_POINT('',#55712);
#12161=VERTEX_POINT('',#55714);
#12162=VERTEX_POINT('',#55718);
#12163=VERTEX_POINT('',#55719);
#12164=VERTEX_POINT('',#55728);
#12165=VERTEX_POINT('',#55732);
#12166=VERTEX_POINT('',#55734);
#12167=VERTEX_POINT('',#55738);
#12168=VERTEX_POINT('',#55740);
#12169=VERTEX_POINT('',#55745);
#12170=VERTEX_POINT('',#55752);
#12171=VERTEX_POINT('',#55754);
#12172=VERTEX_POINT('',#55756);
#12173=VERTEX_POINT('',#55758);
#12174=VERTEX_POINT('',#55760);
#12175=VERTEX_POINT('',#55762);
#12176=VERTEX_POINT('',#55764);
#12177=VERTEX_POINT('',#55766);
#12178=VERTEX_POINT('',#55768);
#12179=VERTEX_POINT('',#55770);
#12180=VERTEX_POINT('',#55772);
#12181=VERTEX_POINT('',#55774);
#12182=VERTEX_POINT('',#55776);
#12183=VERTEX_POINT('',#55778);
#12184=VERTEX_POINT('',#55780);
#12185=VERTEX_POINT('',#55782);
#12186=VERTEX_POINT('',#55784);
#12187=VERTEX_POINT('',#55786);
#12188=VERTEX_POINT('',#55788);
#12189=VERTEX_POINT('',#55790);
#12190=VERTEX_POINT('',#55792);
#12191=VERTEX_POINT('',#55794);
#12192=VERTEX_POINT('',#55796);
#12193=VERTEX_POINT('',#55798);
#12194=VERTEX_POINT('',#55800);
#12195=VERTEX_POINT('',#55802);
#12196=VERTEX_POINT('',#55804);
#12197=VERTEX_POINT('',#55806);
#12198=VERTEX_POINT('',#55808);
#12199=VERTEX_POINT('',#55810);
#12200=VERTEX_POINT('',#55812);
#12201=VERTEX_POINT('',#55814);
#12202=VERTEX_POINT('',#55816);
#12203=VERTEX_POINT('',#55818);
#12204=VERTEX_POINT('',#55820);
#12205=VERTEX_POINT('',#55822);
#12206=VERTEX_POINT('',#55826);
#12207=VERTEX_POINT('',#55828);
#12208=VERTEX_POINT('',#55830);
#12209=VERTEX_POINT('',#55832);
#12210=VERTEX_POINT('',#55834);
#12211=VERTEX_POINT('',#55836);
#12212=VERTEX_POINT('',#55838);
#12213=VERTEX_POINT('',#55840);
#12214=VERTEX_POINT('',#55842);
#12215=VERTEX_POINT('',#55844);
#12216=VERTEX_POINT('',#55846);
#12217=VERTEX_POINT('',#55848);
#12218=VERTEX_POINT('',#55852);
#12219=VERTEX_POINT('',#55853);
#12220=VERTEX_POINT('',#55858);
#12221=VERTEX_POINT('',#55859);
#12222=VERTEX_POINT('',#55864);
#12223=VERTEX_POINT('',#55868);
#12224=VERTEX_POINT('',#55872);
#12225=VERTEX_POINT('',#55876);
#12226=VERTEX_POINT('',#55878);
#12227=VERTEX_POINT('',#55882);
#12228=VERTEX_POINT('',#55884);
#12229=VERTEX_POINT('',#55890);
#12230=VERTEX_POINT('',#55896);
#12231=VERTEX_POINT('',#55897);
#12232=VERTEX_POINT('',#55902);
#12233=VERTEX_POINT('',#55903);
#12234=VERTEX_POINT('',#55910);
#12235=VERTEX_POINT('',#55911);
#12236=VERTEX_POINT('',#55916);
#12237=VERTEX_POINT('',#55917);
#12238=VERTEX_POINT('',#55926);
#12239=VERTEX_POINT('',#55927);
#12240=VERTEX_POINT('',#55932);
#12241=VERTEX_POINT('',#55933);
#12242=VERTEX_POINT('',#55940);
#12243=VERTEX_POINT('',#55942);
#12244=VERTEX_POINT('',#55948);
#12245=VERTEX_POINT('',#55949);
#12246=VERTEX_POINT('',#55954);
#12247=VERTEX_POINT('',#55955);
#12248=VERTEX_POINT('',#55962);
#12249=VERTEX_POINT('',#55963);
#12250=VERTEX_POINT('',#55968);
#12251=VERTEX_POINT('',#55969);
#12252=VERTEX_POINT('',#55980);
#12253=VERTEX_POINT('',#55981);
#12254=VERTEX_POINT('',#55986);
#12255=VERTEX_POINT('',#55987);
#12256=VERTEX_POINT('',#55994);
#12257=VERTEX_POINT('',#55996);
#12258=VERTEX_POINT('',#56000);
#12259=VERTEX_POINT('',#56002);
#12260=VERTEX_POINT('',#56006);
#12261=VERTEX_POINT('',#56007);
#12262=VERTEX_POINT('',#56012);
#12263=VERTEX_POINT('',#56016);
#12264=VERTEX_POINT('',#56022);
#12265=VERTEX_POINT('',#56038);
#12266=VERTEX_POINT('',#56045);
#12267=VERTEX_POINT('',#56049);
#14591=EDGE_CURVE('',#11629,#11629,#9916,.T.);
#14592=EDGE_CURVE('',#11629,#11630,#6305,.T.);
#14593=EDGE_CURVE('',#11630,#11630,#9917,.T.);
#14594=EDGE_CURVE('',#11631,#11631,#9918,.T.);
#14595=EDGE_CURVE('',#11631,#11632,#6306,.T.);
#14596=EDGE_CURVE('',#11632,#11632,#9919,.T.);
#14597=EDGE_CURVE('',#11633,#11633,#9920,.T.);
#14598=EDGE_CURVE('',#11633,#11634,#6307,.T.);
#14599=EDGE_CURVE('',#11634,#11634,#9921,.T.);
#14600=EDGE_CURVE('',#11635,#11629,#6308,.T.);
#14601=EDGE_CURVE('',#11636,#11631,#6309,.T.);
#14602=EDGE_CURVE('',#11637,#11637,#9922,.T.);
#14603=EDGE_CURVE('',#11637,#11638,#6310,.T.);
#14604=EDGE_CURVE('',#11638,#11638,#9923,.T.);
#14605=EDGE_CURVE('',#11639,#11639,#9924,.T.);
#14606=EDGE_CURVE('',#11639,#11640,#6311,.T.);
#14607=EDGE_CURVE('',#11640,#11640,#9925,.T.);
#14608=EDGE_CURVE('',#11641,#11641,#9926,.T.);
#14609=EDGE_CURVE('',#11641,#11642,#6312,.T.);
#14610=EDGE_CURVE('',#11642,#11642,#9927,.T.);
#14611=EDGE_CURVE('',#11643,#11643,#9928,.T.);
#14612=EDGE_CURVE('',#11643,#11644,#6313,.T.);
#14613=EDGE_CURVE('',#11644,#11644,#9929,.T.);
#14614=EDGE_CURVE('',#11645,#11645,#9930,.T.);
#14615=EDGE_CURVE('',#11645,#11646,#6314,.T.);
#14616=EDGE_CURVE('',#11646,#11646,#9931,.T.);
#14617=EDGE_CURVE('',#11647,#11647,#9932,.T.);
#14618=EDGE_CURVE('',#11647,#11648,#6315,.T.);
#14619=EDGE_CURVE('',#11648,#11648,#9933,.T.);
#14620=EDGE_CURVE('',#11649,#11649,#9934,.T.);
#14621=EDGE_CURVE('',#11649,#11650,#6316,.T.);
#14622=EDGE_CURVE('',#11650,#11650,#9935,.T.);
#14623=EDGE_CURVE('',#11651,#11651,#9936,.T.);
#14624=EDGE_CURVE('',#11651,#11652,#6317,.T.);
#14625=EDGE_CURVE('',#11652,#11653,#9937,.T.);
#14626=EDGE_CURVE('',#11653,#11654,#6318,.T.);
#14627=EDGE_CURVE('',#11654,#11655,#9938,.T.);
#14628=EDGE_CURVE('',#11652,#11655,#6319,.T.);
#14629=EDGE_CURVE('',#11656,#11645,#6320,.T.);
#14630=EDGE_CURVE('',#11657,#11647,#6321,.T.);
#14631=EDGE_CURVE('',#11658,#11658,#9939,.T.);
#14632=EDGE_CURVE('',#11658,#11659,#6322,.T.);
#14633=EDGE_CURVE('',#11659,#11660,#6323,.T.);
#14634=EDGE_CURVE('',#11660,#11661,#9940,.T.);
#14635=EDGE_CURVE('',#11662,#11661,#6324,.T.);
#14636=EDGE_CURVE('',#11662,#11659,#9941,.T.);
#14637=EDGE_CURVE('',#11663,#11664,#860,.T.);
#14638=EDGE_CURVE('',#11665,#11663,#861,.T.);
#14639=EDGE_CURVE('',#11666,#11665,#862,.T.);
#14640=EDGE_CURVE('',#11666,#11667,#11,.T.);
#14641=EDGE_CURVE('',#11668,#11667,#9942,.T.);
#14642=EDGE_CURVE('',#11667,#11668,#9943,.T.);
#14643=EDGE_CURVE('',#11669,#11666,#863,.T.);
#14644=EDGE_CURVE('',#11670,#11669,#864,.T.);
#14645=EDGE_CURVE('',#11664,#11670,#865,.T.);
#14646=EDGE_CURVE('',#11671,#11671,#9944,.T.);
#14647=EDGE_CURVE('',#11671,#11668,#6325,.T.);
#14648=EDGE_CURVE('',#11672,#11672,#9945,.T.);
#14649=EDGE_CURVE('',#11672,#11673,#6326,.T.);
#14650=EDGE_CURVE('',#11673,#11673,#9946,.T.);
#14651=EDGE_CURVE('',#11674,#11675,#146,.T.);
#14652=EDGE_CURVE('',#11676,#11674,#6327,.T.);
#14653=EDGE_CURVE('',#11676,#11677,#6328,.T.);
#14654=EDGE_CURVE('',#11677,#11675,#6329,.T.);
#14655=EDGE_CURVE('',#11678,#11674,#147,.T.);
#14656=EDGE_CURVE('',#11678,#11679,#6330,.T.);
#14657=EDGE_CURVE('',#11680,#11679,#148,.T.);
#14658=EDGE_CURVE('',#11674,#11680,#6331,.T.);
#14659=EDGE_CURVE('',#11681,#11682,#149,.T.);
#14660=EDGE_CURVE('',#11681,#11683,#6332,.T.);
#14661=EDGE_CURVE('',#11684,#11683,#150,.T.);
#14662=EDGE_CURVE('',#11682,#11684,#6333,.T.);
#14663=EDGE_CURVE('',#11683,#11685,#151,.T.);
#14664=EDGE_CURVE('',#11683,#11686,#6334,.T.);
#14665=EDGE_CURVE('',#11687,#11686,#6335,.T.);
#14666=EDGE_CURVE('',#11685,#11687,#6336,.T.);
#14667=EDGE_CURVE('',#11688,#11689,#6337,.T.);
#14668=EDGE_CURVE('',#11688,#11690,#6338,.T.);
#14669=EDGE_CURVE('',#11690,#11691,#6339,.T.);
#14670=EDGE_CURVE('',#11691,#11689,#6340,.T.);
#14671=EDGE_CURVE('',#11692,#11693,#6341,.T.);
#14672=EDGE_CURVE('',#11692,#11694,#6342,.T.);
#14673=EDGE_CURVE('',#11694,#11695,#6343,.T.);
#14674=EDGE_CURVE('',#11695,#11693,#6344,.T.);
#14675=EDGE_CURVE('',#11696,#11697,#6345,.T.);
#14676=EDGE_CURVE('',#11696,#11698,#6346,.T.);
#14677=EDGE_CURVE('',#11698,#11699,#6347,.T.);
#14678=EDGE_CURVE('',#11699,#11697,#6348,.T.);
#14679=EDGE_CURVE('',#11700,#11701,#6349,.T.);
#14680=EDGE_CURVE('',#11700,#11702,#6350,.T.);
#14681=EDGE_CURVE('',#11702,#11703,#6351,.T.);
#14682=EDGE_CURVE('',#11703,#11701,#6352,.T.);
#14683=EDGE_CURVE('',#11704,#11705,#6353,.T.);
#14684=EDGE_CURVE('',#11704,#11706,#6354,.T.);
#14685=EDGE_CURVE('',#11706,#11707,#6355,.T.);
#14686=EDGE_CURVE('',#11707,#11705,#6356,.T.);
#14687=EDGE_CURVE('',#11708,#11709,#6357,.T.);
#14688=EDGE_CURVE('',#11708,#11710,#6358,.T.);
#14689=EDGE_CURVE('',#11710,#11711,#6359,.T.);
#14690=EDGE_CURVE('',#11711,#11709,#6360,.T.);
#14691=EDGE_CURVE('',#11712,#11713,#6361,.T.);
#14692=EDGE_CURVE('',#11712,#11714,#6362,.T.);
#14693=EDGE_CURVE('',#11714,#11715,#6363,.T.);
#14694=EDGE_CURVE('',#11715,#11713,#6364,.T.);
#14695=EDGE_CURVE('',#11716,#11717,#6365,.T.);
#14696=EDGE_CURVE('',#11716,#11718,#6366,.T.);
#14697=EDGE_CURVE('',#11718,#11719,#6367,.T.);
#14698=EDGE_CURVE('',#11719,#11717,#6368,.T.);
#14699=EDGE_CURVE('',#11720,#11721,#6369,.T.);
#14700=EDGE_CURVE('',#11722,#11720,#6370,.T.);
#14701=EDGE_CURVE('',#11722,#11723,#6371,.T.);
#14702=EDGE_CURVE('',#11723,#11721,#6372,.T.);
#14703=EDGE_CURVE('',#11724,#11720,#6373,.T.);
#14704=EDGE_CURVE('',#11725,#11724,#6374,.T.);
#14705=EDGE_CURVE('',#11725,#11722,#6375,.T.);
#14706=EDGE_CURVE('',#11726,#11727,#6376,.T.);
#14707=EDGE_CURVE('',#11728,#11726,#6377,.T.);
#14708=EDGE_CURVE('',#11728,#11729,#6378,.T.);
#14709=EDGE_CURVE('',#11729,#11727,#6379,.T.);
#14710=EDGE_CURVE('',#11730,#11726,#6380,.T.);
#14711=EDGE_CURVE('',#11730,#11731,#6381,.T.);
#14712=EDGE_CURVE('',#11731,#11728,#6382,.T.);
#14713=EDGE_CURVE('',#11732,#11733,#6383,.T.);
#14714=EDGE_CURVE('',#11732,#11734,#6384,.T.);
#14715=EDGE_CURVE('',#11734,#11735,#6385,.T.);
#14716=EDGE_CURVE('',#11735,#11733,#6386,.T.);
#14717=EDGE_CURVE('',#11736,#11737,#6387,.T.);
#14718=EDGE_CURVE('',#11736,#11738,#6388,.T.);
#14719=EDGE_CURVE('',#11738,#11739,#6389,.T.);
#14720=EDGE_CURVE('',#11739,#11737,#6390,.T.);
#14721=EDGE_CURVE('',#11740,#11741,#6391,.T.);
#14722=EDGE_CURVE('',#11740,#11742,#6392,.T.);
#14723=EDGE_CURVE('',#11742,#11743,#6393,.T.);
#14724=EDGE_CURVE('',#11743,#11741,#6394,.T.);
#14725=EDGE_CURVE('',#11744,#11745,#6395,.T.);
#14726=EDGE_CURVE('',#11746,#11744,#6396,.T.);
#14727=EDGE_CURVE('',#11746,#11747,#6397,.T.);
#14728=EDGE_CURVE('',#11747,#11745,#6398,.T.);
#14729=EDGE_CURVE('',#11701,#11744,#6399,.T.);
#14730=EDGE_CURVE('',#11703,#11746,#6400,.T.);
#14731=EDGE_CURVE('',#11748,#11749,#9947,.T.);
#14732=EDGE_CURVE('',#11748,#11750,#6401,.T.);
#14733=EDGE_CURVE('',#11750,#11751,#9948,.T.);
#14734=EDGE_CURVE('',#11751,#11749,#6402,.T.);
#14735=EDGE_CURVE('',#11752,#11753,#9949,.T.);
#14736=EDGE_CURVE('',#11752,#11754,#6403,.T.);
#14737=EDGE_CURVE('',#11754,#11755,#9950,.T.);
#14738=EDGE_CURVE('',#11755,#11753,#6404,.T.);
#14739=EDGE_CURVE('',#11756,#11757,#9951,.T.);
#14740=EDGE_CURVE('',#11756,#11758,#6405,.T.);
#14741=EDGE_CURVE('',#11758,#11759,#9952,.T.);
#14742=EDGE_CURVE('',#11759,#11757,#6406,.T.);
#14743=EDGE_CURVE('',#11760,#11761,#9953,.T.);
#14744=EDGE_CURVE('',#11760,#11762,#6407,.T.);
#14745=EDGE_CURVE('',#11762,#11763,#9954,.T.);
#14746=EDGE_CURVE('',#11763,#11761,#6408,.T.);
#14747=EDGE_CURVE('',#11733,#11730,#9955,.T.);
#14748=EDGE_CURVE('',#11731,#11735,#9956,.T.);
#14749=EDGE_CURVE('',#11721,#11716,#9957,.T.);
#14750=EDGE_CURVE('',#11718,#11723,#9958,.T.);
#14751=EDGE_CURVE('',#11741,#11736,#9959,.T.);
#14752=EDGE_CURVE('',#11738,#11743,#9960,.T.);
#14753=EDGE_CURVE('',#11693,#11740,#9961,.T.);
#14754=EDGE_CURVE('',#11742,#11695,#9962,.T.);
#14755=EDGE_CURVE('',#11757,#11692,#9963,.T.);
#14756=EDGE_CURVE('',#11694,#11759,#9964,.T.);
#14757=EDGE_CURVE('',#11745,#11756,#9965,.T.);
#14758=EDGE_CURVE('',#11758,#11747,#9966,.T.);
#14759=EDGE_CURVE('',#11737,#11760,#9967,.T.);
#14760=EDGE_CURVE('',#11762,#11739,#9968,.T.);
#14761=EDGE_CURVE('',#11761,#11688,#9969,.T.);
#14762=EDGE_CURVE('',#11690,#11763,#9970,.T.);
#14763=EDGE_CURVE('',#11689,#11732,#9971,.T.);
#14764=EDGE_CURVE('',#11734,#11691,#9972,.T.);
#14765=EDGE_CURVE('',#11717,#11712,#9973,.T.);
#14766=EDGE_CURVE('',#11714,#11719,#9974,.T.);
#14767=EDGE_CURVE('',#11713,#11752,#9975,.T.);
#14768=EDGE_CURVE('',#11754,#11715,#9976,.T.);
#14769=EDGE_CURVE('',#11753,#11696,#9977,.T.);
#14770=EDGE_CURVE('',#11698,#11755,#9978,.T.);
#14771=EDGE_CURVE('',#11697,#11708,#9979,.T.);
#14772=EDGE_CURVE('',#11710,#11699,#9980,.T.);
#14773=EDGE_CURVE('',#11709,#11704,#9981,.T.);
#14774=EDGE_CURVE('',#11706,#11711,#9982,.T.);
#14775=EDGE_CURVE('',#11705,#11748,#9983,.T.);
#14776=EDGE_CURVE('',#11750,#11707,#9984,.T.);
#14777=EDGE_CURVE('',#11749,#11700,#9985,.T.);
#14778=EDGE_CURVE('',#11702,#11751,#9986,.T.);
#14779=EDGE_CURVE('',#11764,#11765,#6409,.T.);
#14780=EDGE_CURVE('',#11766,#11765,#6410,.T.);
#14781=EDGE_CURVE('',#11767,#11766,#6411,.T.);
#14782=EDGE_CURVE('',#11764,#11767,#6412,.T.);
#14783=EDGE_CURVE('',#11725,#11768,#6413,.T.);
#14784=EDGE_CURVE('',#11768,#11769,#6414,.T.);
#14785=EDGE_CURVE('',#11769,#11764,#6415,.T.);
#14786=EDGE_CURVE('',#11767,#11770,#6416,.T.);
#14787=EDGE_CURVE('',#11770,#11771,#6417,.T.);
#14788=EDGE_CURVE('',#11771,#11729,#6418,.T.);
#14789=EDGE_CURVE('',#11769,#11772,#6419,.T.);
#14790=EDGE_CURVE('',#11765,#11772,#6420,.T.);
#14791=EDGE_CURVE('',#11768,#11773,#6421,.T.);
#14792=EDGE_CURVE('',#11772,#11773,#6422,.T.);
#14793=EDGE_CURVE('',#11773,#11724,#6423,.T.);
#14794=EDGE_CURVE('',#11771,#11774,#6424,.T.);
#14795=EDGE_CURVE('',#11727,#11774,#6425,.T.);
#14796=EDGE_CURVE('',#11770,#11775,#6426,.T.);
#14797=EDGE_CURVE('',#11774,#11775,#6427,.T.);
#14798=EDGE_CURVE('',#11775,#11766,#6428,.T.);
#14799=EDGE_CURVE('',#11776,#11664,#6429,.T.);
#14800=EDGE_CURVE('',#11777,#11670,#6430,.T.);
#14801=EDGE_CURVE('',#11776,#11777,#6431,.T.);
#14802=EDGE_CURVE('',#11778,#11776,#6432,.T.);
#14803=EDGE_CURVE('',#11778,#11663,#6433,.T.);
#14804=EDGE_CURVE('',#11779,#11665,#6434,.T.);
#14805=EDGE_CURVE('',#11779,#11778,#6435,.T.);
#14806=EDGE_CURVE('',#11780,#11666,#6436,.T.);
#14807=EDGE_CURVE('',#11780,#11779,#6437,.T.);
#14808=EDGE_CURVE('',#11781,#11669,#6438,.T.);
#14809=EDGE_CURVE('',#11781,#11780,#6439,.T.);
#14810=EDGE_CURVE('',#11777,#11781,#6440,.T.);
#14811=EDGE_CURVE('',#11782,#11783,#6441,.T.);
#14812=EDGE_CURVE('',#11784,#11782,#9987,.T.);
#14813=EDGE_CURVE('',#11785,#11784,#6442,.T.);
#14814=EDGE_CURVE('',#11786,#11785,#9988,.T.);
#14815=EDGE_CURVE('',#11787,#11786,#6443,.T.);
#14816=EDGE_CURVE('',#11788,#11787,#9989,.T.);
#14817=EDGE_CURVE('',#11789,#11788,#9990,.T.);
#14818=EDGE_CURVE('',#11790,#11789,#9991,.T.);
#14819=EDGE_CURVE('',#11791,#11790,#6444,.T.);
#14820=EDGE_CURVE('',#11792,#11791,#9992,.T.);
#14821=EDGE_CURVE('',#11793,#11792,#6445,.T.);
#14822=EDGE_CURVE('',#11794,#11793,#9993,.T.);
#14823=EDGE_CURVE('',#11795,#11794,#6446,.T.);
#14824=EDGE_CURVE('',#11796,#11795,#9994,.T.);
#14825=EDGE_CURVE('',#11797,#11796,#9995,.T.);
#14826=EDGE_CURVE('',#11798,#11797,#9996,.T.);
#14827=EDGE_CURVE('',#11799,#11798,#6447,.T.);
#14828=EDGE_CURVE('',#11800,#11799,#6448,.T.);
#14829=EDGE_CURVE('',#11801,#11800,#6449,.T.);
#14830=EDGE_CURVE('',#11802,#11801,#9997,.T.);
#14831=EDGE_CURVE('',#11803,#11802,#9998,.T.);
#14832=EDGE_CURVE('',#11804,#11803,#9999,.T.);
#14833=EDGE_CURVE('',#11805,#11804,#6450,.T.);
#14834=EDGE_CURVE('',#11806,#11805,#10000,.T.);
#14835=EDGE_CURVE('',#11807,#11806,#6451,.T.);
#14836=EDGE_CURVE('',#11808,#11807,#10001,.T.);
#14837=EDGE_CURVE('',#11809,#11808,#6452,.T.);
#14838=EDGE_CURVE('',#11810,#11809,#10002,.T.);
#14839=EDGE_CURVE('',#11811,#11810,#10003,.T.);
#14840=EDGE_CURVE('',#11812,#11811,#10004,.T.);
#14841=EDGE_CURVE('',#11813,#11812,#6453,.T.);
#14842=EDGE_CURVE('',#11814,#11813,#10005,.T.);
#14843=EDGE_CURVE('',#11815,#11814,#6454,.T.);
#14844=EDGE_CURVE('',#11816,#11815,#10006,.T.);
#14845=EDGE_CURVE('',#11817,#11816,#6455,.T.);
#14846=EDGE_CURVE('',#11818,#11817,#6456,.T.);
#14847=EDGE_CURVE('',#11819,#11818,#6457,.T.);
#14848=EDGE_CURVE('',#11820,#11819,#6458,.T.);
#14849=EDGE_CURVE('',#11821,#11820,#6459,.T.);
#14850=EDGE_CURVE('',#11822,#11821,#6460,.T.);
#14851=EDGE_CURVE('',#11823,#11822,#6461,.T.);
#14852=EDGE_CURVE('',#11824,#11823,#6462,.T.);
#14853=EDGE_CURVE('',#11825,#11824,#6463,.T.);
#14854=EDGE_CURVE('',#11783,#11825,#6464,.T.);
#14855=EDGE_CURVE('',#11826,#11827,#6465,.T.);
#14856=EDGE_CURVE('',#11782,#11826,#6466,.T.);
#14857=EDGE_CURVE('',#11783,#11827,#6467,.T.);
#14858=EDGE_CURVE('',#11828,#11826,#10007,.T.);
#14859=EDGE_CURVE('',#11784,#11828,#6468,.T.);
#14860=EDGE_CURVE('',#11829,#11828,#6469,.T.);
#14861=EDGE_CURVE('',#11785,#11829,#6470,.T.);
#14862=EDGE_CURVE('',#11830,#11829,#10008,.T.);
#14863=EDGE_CURVE('',#11786,#11830,#6471,.T.);
#14864=EDGE_CURVE('',#11831,#11830,#6472,.T.);
#14865=EDGE_CURVE('',#11787,#11831,#6473,.T.);
#14866=EDGE_CURVE('',#11832,#11831,#10009,.T.);
#14867=EDGE_CURVE('',#11788,#11832,#6474,.T.);
#14868=EDGE_CURVE('',#11833,#11832,#10010,.T.);
#14869=EDGE_CURVE('',#11789,#11833,#6475,.T.);
#14870=EDGE_CURVE('',#11834,#11833,#10011,.T.);
#14871=EDGE_CURVE('',#11790,#11834,#6476,.T.);
#14872=EDGE_CURVE('',#11835,#11834,#6477,.T.);
#14873=EDGE_CURVE('',#11791,#11835,#6478,.T.);
#14874=EDGE_CURVE('',#11836,#11835,#10012,.T.);
#14875=EDGE_CURVE('',#11792,#11836,#6479,.T.);
#14876=EDGE_CURVE('',#11837,#11836,#6480,.T.);
#14877=EDGE_CURVE('',#11793,#11837,#6481,.T.);
#14878=EDGE_CURVE('',#11838,#11837,#10013,.T.);
#14879=EDGE_CURVE('',#11794,#11838,#6482,.T.);
#14880=EDGE_CURVE('',#11839,#11838,#6483,.T.);
#14881=EDGE_CURVE('',#11795,#11839,#6484,.T.);
#14882=EDGE_CURVE('',#11840,#11839,#10014,.T.);
#14883=EDGE_CURVE('',#11796,#11840,#6485,.T.);
#14884=EDGE_CURVE('',#11841,#11840,#10015,.T.);
#14885=EDGE_CURVE('',#11797,#11841,#6486,.T.);
#14886=EDGE_CURVE('',#11842,#11841,#10016,.T.);
#14887=EDGE_CURVE('',#11798,#11842,#6487,.T.);
#14888=EDGE_CURVE('',#11843,#11842,#6488,.T.);
#14889=EDGE_CURVE('',#11799,#11843,#6489,.T.);
#14890=EDGE_CURVE('',#11844,#11843,#6490,.T.);
#14891=EDGE_CURVE('',#11800,#11844,#6491,.T.);
#14892=EDGE_CURVE('',#11845,#11844,#6492,.T.);
#14893=EDGE_CURVE('',#11801,#11845,#6493,.T.);
#14894=EDGE_CURVE('',#11846,#11845,#10017,.T.);
#14895=EDGE_CURVE('',#11802,#11846,#6494,.T.);
#14896=EDGE_CURVE('',#11847,#11846,#10018,.T.);
#14897=EDGE_CURVE('',#11803,#11847,#6495,.T.);
#14898=EDGE_CURVE('',#11848,#11847,#10019,.T.);
#14899=EDGE_CURVE('',#11804,#11848,#6496,.T.);
#14900=EDGE_CURVE('',#11849,#11848,#6497,.T.);
#14901=EDGE_CURVE('',#11805,#11849,#6498,.T.);
#14902=EDGE_CURVE('',#11850,#11849,#10020,.T.);
#14903=EDGE_CURVE('',#11806,#11850,#6499,.T.);
#14904=EDGE_CURVE('',#11851,#11850,#6500,.T.);
#14905=EDGE_CURVE('',#11807,#11851,#6501,.T.);
#14906=EDGE_CURVE('',#11852,#11851,#10021,.T.);
#14907=EDGE_CURVE('',#11808,#11852,#6502,.T.);
#14908=EDGE_CURVE('',#11853,#11852,#6503,.T.);
#14909=EDGE_CURVE('',#11809,#11853,#6504,.T.);
#14910=EDGE_CURVE('',#11854,#11853,#10022,.T.);
#14911=EDGE_CURVE('',#11810,#11854,#6505,.T.);
#14912=EDGE_CURVE('',#11855,#11854,#10023,.T.);
#14913=EDGE_CURVE('',#11811,#11855,#6506,.T.);
#14914=EDGE_CURVE('',#11856,#11855,#10024,.T.);
#14915=EDGE_CURVE('',#11812,#11856,#6507,.T.);
#14916=EDGE_CURVE('',#11857,#11856,#6508,.T.);
#14917=EDGE_CURVE('',#11813,#11857,#6509,.T.);
#14918=EDGE_CURVE('',#11858,#11857,#10025,.T.);
#14919=EDGE_CURVE('',#11814,#11858,#6510,.T.);
#14920=EDGE_CURVE('',#11859,#11858,#6511,.T.);
#14921=EDGE_CURVE('',#11815,#11859,#6512,.T.);
#14922=EDGE_CURVE('',#11860,#11859,#10026,.T.);
#14923=EDGE_CURVE('',#11816,#11860,#6513,.T.);
#14924=EDGE_CURVE('',#11861,#11860,#6514,.T.);
#14925=EDGE_CURVE('',#11817,#11861,#6515,.T.);
#14926=EDGE_CURVE('',#11862,#11861,#6516,.T.);
#14927=EDGE_CURVE('',#11818,#11862,#6517,.T.);
#14928=EDGE_CURVE('',#11863,#11862,#6518,.T.);
#14929=EDGE_CURVE('',#11819,#11863,#6519,.T.);
#14930=EDGE_CURVE('',#11864,#11863,#6520,.T.);
#14931=EDGE_CURVE('',#11820,#11864,#6521,.T.);
#14932=EDGE_CURVE('',#11865,#11864,#6522,.T.);
#14933=EDGE_CURVE('',#11821,#11865,#6523,.T.);
#14934=EDGE_CURVE('',#11866,#11865,#6524,.T.);
#14935=EDGE_CURVE('',#11822,#11866,#6525,.T.);
#14936=EDGE_CURVE('',#11867,#11866,#6526,.T.);
#14937=EDGE_CURVE('',#11823,#11867,#6527,.T.);
#14938=EDGE_CURVE('',#11868,#11867,#6528,.T.);
#14939=EDGE_CURVE('',#11824,#11868,#6529,.T.);
#14940=EDGE_CURVE('',#11869,#11868,#6530,.T.);
#14941=EDGE_CURVE('',#11825,#11869,#6531,.T.);
#14942=EDGE_CURVE('',#11827,#11869,#6532,.T.);
#14943=EDGE_CURVE('',#11662,#11870,#6533,.T.);
#14944=EDGE_CURVE('',#11870,#11871,#10027,.T.);
#14945=EDGE_CURVE('',#11871,#11659,#6534,.T.);
#14946=EDGE_CURVE('',#11872,#11873,#6535,.T.);
#14947=EDGE_CURVE('',#11874,#11872,#6536,.T.);
#14948=EDGE_CURVE('',#11875,#11874,#10028,.T.);
#14949=EDGE_CURVE('',#11876,#11875,#6537,.T.);
#14950=EDGE_CURVE('',#11877,#11876,#6538,.T.);
#14951=EDGE_CURVE('',#11878,#11877,#6539,.T.);
#14952=EDGE_CURVE('',#11879,#11878,#6540,.T.);
#14953=EDGE_CURVE('',#11880,#11879,#6541,.T.);
#14954=EDGE_CURVE('',#11880,#11881,#6542,.T.);
#14955=EDGE_CURVE('',#11881,#11882,#6543,.T.);
#14956=EDGE_CURVE('',#11882,#11883,#10029,.T.);
#14957=EDGE_CURVE('',#11883,#11884,#6544,.T.);
#14958=EDGE_CURVE('',#11884,#11885,#10030,.T.);
#14959=EDGE_CURVE('',#11885,#11886,#6545,.T.);
#14960=EDGE_CURVE('',#11886,#11887,#10031,.T.);
#14961=EDGE_CURVE('',#11887,#11888,#10032,.T.);
#14962=EDGE_CURVE('',#11888,#11889,#10033,.T.);
#14963=EDGE_CURVE('',#11889,#11890,#6546,.T.);
#14964=EDGE_CURVE('',#11890,#11891,#10034,.T.);
#14965=EDGE_CURVE('',#11891,#11892,#6547,.T.);
#14966=EDGE_CURVE('',#11892,#11893,#10035,.T.);
#14967=EDGE_CURVE('',#11893,#11894,#6548,.T.);
#14968=EDGE_CURVE('',#11894,#11895,#10036,.T.);
#14969=EDGE_CURVE('',#11895,#11896,#10037,.T.);
#14970=EDGE_CURVE('',#11896,#11897,#10038,.T.);
#14971=EDGE_CURVE('',#11897,#11898,#6549,.T.);
#14972=EDGE_CURVE('',#11898,#11899,#6550,.T.);
#14973=EDGE_CURVE('',#11899,#11900,#6551,.T.);
#14974=EDGE_CURVE('',#11900,#11901,#10039,.T.);
#14975=EDGE_CURVE('',#11901,#11902,#10040,.T.);
#14976=EDGE_CURVE('',#11902,#11903,#10041,.T.);
#14977=EDGE_CURVE('',#11903,#11904,#6552,.T.);
#14978=EDGE_CURVE('',#11904,#11905,#10042,.T.);
#14979=EDGE_CURVE('',#11905,#11906,#6553,.T.);
#14980=EDGE_CURVE('',#11906,#11907,#10043,.T.);
#14981=EDGE_CURVE('',#11907,#11908,#6554,.T.);
#14982=EDGE_CURVE('',#11908,#11909,#10044,.T.);
#14983=EDGE_CURVE('',#11909,#11910,#10045,.T.);
#14984=EDGE_CURVE('',#11910,#11911,#10046,.T.);
#14985=EDGE_CURVE('',#11911,#11912,#6555,.T.);
#14986=EDGE_CURVE('',#11912,#11913,#10047,.T.);
#14987=EDGE_CURVE('',#11913,#11914,#6556,.T.);
#14988=EDGE_CURVE('',#11914,#11915,#10048,.T.);
#14989=EDGE_CURVE('',#11915,#11916,#6557,.T.);
#14990=EDGE_CURVE('',#11916,#11917,#6558,.T.);
#14991=EDGE_CURVE('',#11918,#11917,#6559,.T.);
#14992=EDGE_CURVE('',#11919,#11918,#6560,.T.);
#14993=EDGE_CURVE('',#11873,#11919,#6561,.T.);
#14994=EDGE_CURVE('',#11920,#11660,#6562,.T.);
#14995=EDGE_CURVE('',#11871,#11920,#6563,.T.);
#14996=EDGE_CURVE('',#11661,#11921,#6564,.T.);
#14997=EDGE_CURVE('',#11870,#11921,#6565,.T.);
#14998=EDGE_CURVE('',#11921,#11920,#10049,.T.);
#14999=EDGE_CURVE('',#11652,#11922,#6566,.T.);
#15000=EDGE_CURVE('',#11922,#11923,#10050,.T.);
#15001=EDGE_CURVE('',#11923,#11653,#6567,.T.);
#15002=EDGE_CURVE('',#11924,#11925,#6568,.T.);
#15003=EDGE_CURVE('',#11925,#11917,#6569,.T.);
#15004=EDGE_CURVE('',#11924,#11916,#6570,.T.);
#15005=EDGE_CURVE('',#11925,#11926,#6571,.T.);
#15006=EDGE_CURVE('',#11926,#11918,#6572,.T.);
#15007=EDGE_CURVE('',#11926,#11927,#6573,.T.);
#15008=EDGE_CURVE('',#11927,#11919,#6574,.T.);
#15009=EDGE_CURVE('',#11927,#11928,#6575,.T.);
#15010=EDGE_CURVE('',#11928,#11873,#6576,.T.);
#15011=EDGE_CURVE('',#11929,#11930,#6577,.T.);
#15012=EDGE_CURVE('',#11929,#11872,#6578,.T.);
#15013=EDGE_CURVE('',#11928,#11931,#6579,.T.);
#15014=EDGE_CURVE('',#11931,#11877,#6580,.T.);
#15015=EDGE_CURVE('',#11930,#11876,#6581,.T.);
#15016=EDGE_CURVE('',#11931,#11932,#6582,.T.);
#15017=EDGE_CURVE('',#11932,#11878,#6583,.T.);
#15018=EDGE_CURVE('',#11932,#11933,#6584,.T.);
#15019=EDGE_CURVE('',#11933,#11879,#6585,.T.);
#15020=EDGE_CURVE('',#11933,#11934,#6586,.T.);
#15021=EDGE_CURVE('',#11934,#11880,#6587,.T.);
#15022=EDGE_CURVE('',#11934,#11935,#6588,.T.);
#15023=EDGE_CURVE('',#11935,#11881,#6589,.T.);
#15024=EDGE_CURVE('',#11935,#11936,#6590,.T.);
#15025=EDGE_CURVE('',#11936,#11882,#6591,.T.);
#15026=EDGE_CURVE('',#11936,#11937,#10051,.T.);
#15027=EDGE_CURVE('',#11883,#11937,#6592,.T.);
#15028=EDGE_CURVE('',#11937,#11938,#6593,.T.);
#15029=EDGE_CURVE('',#11938,#11884,#6594,.T.);
#15030=EDGE_CURVE('',#11938,#11939,#10052,.T.);
#15031=EDGE_CURVE('',#11885,#11939,#6595,.T.);
#15032=EDGE_CURVE('',#11939,#11940,#6596,.T.);
#15033=EDGE_CURVE('',#11940,#11886,#6597,.T.);
#15034=EDGE_CURVE('',#11940,#11941,#10053,.T.);
#15035=EDGE_CURVE('',#11887,#11941,#6598,.T.);
#15036=EDGE_CURVE('',#11941,#11942,#10054,.T.);
#15037=EDGE_CURVE('',#11942,#11888,#6599,.T.);
#15038=EDGE_CURVE('',#11942,#11943,#10055,.T.);
#15039=EDGE_CURVE('',#11889,#11943,#6600,.T.);
#15040=EDGE_CURVE('',#11943,#11944,#6601,.T.);
#15041=EDGE_CURVE('',#11944,#11890,#6602,.T.);
#15042=EDGE_CURVE('',#11944,#11945,#10056,.T.);
#15043=EDGE_CURVE('',#11891,#11945,#6603,.T.);
#15044=EDGE_CURVE('',#11945,#11946,#6604,.T.);
#15045=EDGE_CURVE('',#11946,#11892,#6605,.T.);
#15046=EDGE_CURVE('',#11946,#11947,#10057,.T.);
#15047=EDGE_CURVE('',#11893,#11947,#6606,.T.);
#15048=EDGE_CURVE('',#11947,#11948,#6607,.T.);
#15049=EDGE_CURVE('',#11948,#11894,#6608,.T.);
#15050=EDGE_CURVE('',#11948,#11949,#10058,.T.);
#15051=EDGE_CURVE('',#11895,#11949,#6609,.T.);
#15052=EDGE_CURVE('',#11949,#11950,#10059,.T.);
#15053=EDGE_CURVE('',#11950,#11896,#6610,.T.);
#15054=EDGE_CURVE('',#11950,#11951,#10060,.T.);
#15055=EDGE_CURVE('',#11897,#11951,#6611,.T.);
#15056=EDGE_CURVE('',#11951,#11952,#6612,.T.);
#15057=EDGE_CURVE('',#11952,#11898,#6613,.T.);
#15058=EDGE_CURVE('',#11952,#11953,#6614,.T.);
#15059=EDGE_CURVE('',#11953,#11899,#6615,.T.);
#15060=EDGE_CURVE('',#11953,#11954,#6616,.T.);
#15061=EDGE_CURVE('',#11954,#11900,#6617,.T.);
#15062=EDGE_CURVE('',#11954,#11955,#10061,.T.);
#15063=EDGE_CURVE('',#11901,#11955,#6618,.T.);
#15064=EDGE_CURVE('',#11955,#11956,#10062,.T.);
#15065=EDGE_CURVE('',#11956,#11902,#6619,.T.);
#15066=EDGE_CURVE('',#11956,#11957,#10063,.T.);
#15067=EDGE_CURVE('',#11903,#11957,#6620,.T.);
#15068=EDGE_CURVE('',#11957,#11958,#6621,.T.);
#15069=EDGE_CURVE('',#11958,#11904,#6622,.T.);
#15070=EDGE_CURVE('',#11958,#11959,#10064,.T.);
#15071=EDGE_CURVE('',#11905,#11959,#6623,.T.);
#15072=EDGE_CURVE('',#11959,#11960,#6624,.T.);
#15073=EDGE_CURVE('',#11960,#11906,#6625,.T.);
#15074=EDGE_CURVE('',#11960,#11961,#10065,.T.);
#15075=EDGE_CURVE('',#11907,#11961,#6626,.T.);
#15076=EDGE_CURVE('',#11961,#11962,#6627,.T.);
#15077=EDGE_CURVE('',#11962,#11908,#6628,.T.);
#15078=EDGE_CURVE('',#11962,#11963,#10066,.T.);
#15079=EDGE_CURVE('',#11909,#11963,#6629,.T.);
#15080=EDGE_CURVE('',#11963,#11964,#10067,.T.);
#15081=EDGE_CURVE('',#11964,#11910,#6630,.T.);
#15082=EDGE_CURVE('',#11964,#11965,#10068,.T.);
#15083=EDGE_CURVE('',#11911,#11965,#6631,.T.);
#15084=EDGE_CURVE('',#11965,#11966,#6632,.T.);
#15085=EDGE_CURVE('',#11966,#11912,#6633,.T.);
#15086=EDGE_CURVE('',#11966,#11967,#10069,.T.);
#15087=EDGE_CURVE('',#11913,#11967,#6634,.T.);
#15088=EDGE_CURVE('',#11967,#11968,#6635,.T.);
#15089=EDGE_CURVE('',#11968,#11914,#6636,.T.);
#15090=EDGE_CURVE('',#11968,#11969,#10070,.T.);
#15091=EDGE_CURVE('',#11915,#11969,#6637,.T.);
#15092=EDGE_CURVE('',#11969,#11924,#6638,.T.);
#15093=EDGE_CURVE('',#11970,#11971,#6639,.T.);
#15094=EDGE_CURVE('',#11971,#11972,#6640,.T.);
#15095=EDGE_CURVE('',#11972,#11973,#6641,.T.);
#15096=EDGE_CURVE('',#11973,#11970,#6642,.T.);
#15097=EDGE_CURVE('',#11974,#11975,#6643,.T.);
#15098=EDGE_CURVE('',#11975,#11976,#6644,.T.);
#15099=EDGE_CURVE('',#11976,#11977,#6645,.T.);
#15100=EDGE_CURVE('',#11974,#11977,#6646,.T.);
#15101=EDGE_CURVE('',#11978,#11654,#6647,.T.);
#15102=EDGE_CURVE('',#11923,#11978,#6648,.T.);
#15103=EDGE_CURVE('',#11655,#11979,#6649,.T.);
#15104=EDGE_CURVE('',#11922,#11979,#6650,.T.);
#15105=EDGE_CURVE('',#11979,#11978,#10071,.T.);
#15106=EDGE_CURVE('',#11971,#11980,#10072,.T.);
#15107=EDGE_CURVE('',#11981,#11970,#10073,.T.);
#15108=EDGE_CURVE('',#11980,#11981,#6651,.T.);
#15109=EDGE_CURVE('',#11982,#11980,#6652,.T.);
#15110=EDGE_CURVE('',#11982,#11983,#6653,.T.);
#15111=EDGE_CURVE('',#11983,#11984,#6654,.T.);
#15112=EDGE_CURVE('',#11972,#11984,#6655,.T.);
#15113=EDGE_CURVE('',#11982,#11985,#6656,.T.);
#15114=EDGE_CURVE('',#11985,#11986,#6657,.T.);
#15115=EDGE_CURVE('',#11983,#11986,#6658,.T.);
#15116=EDGE_CURVE('',#11987,#11988,#6659,.T.);
#15117=EDGE_CURVE('',#11988,#11989,#6660,.T.);
#15118=EDGE_CURVE('',#11989,#11990,#6661,.T.);
#15119=EDGE_CURVE('',#11987,#11990,#6662,.T.);
#15120=EDGE_CURVE('',#11991,#11990,#6663,.T.);
#15121=EDGE_CURVE('',#11991,#11976,#10074,.T.);
#15122=EDGE_CURVE('',#11992,#11975,#6664,.T.);
#15123=EDGE_CURVE('',#11992,#11987,#6665,.T.);
#15124=EDGE_CURVE('',#11993,#11991,#6666,.T.);
#15125=EDGE_CURVE('',#11993,#11977,#10075,.T.);
#15126=EDGE_CURVE('',#11994,#11995,#6667,.T.);
#15127=EDGE_CURVE('',#11995,#11996,#6668,.T.);
#15128=EDGE_CURVE('',#11996,#11997,#6669,.T.);
#15129=EDGE_CURVE('',#11997,#11998,#6670,.T.);
#15130=EDGE_CURVE('',#11998,#11999,#6671,.T.);
#15131=EDGE_CURVE('',#11999,#12000,#6672,.T.);
#15132=EDGE_CURVE('',#12000,#12001,#6673,.T.);
#15133=EDGE_CURVE('',#12001,#12002,#6674,.T.);
#15134=EDGE_CURVE('',#12002,#12003,#6675,.T.);
#15135=EDGE_CURVE('',#12003,#12004,#6676,.T.);
#15136=EDGE_CURVE('',#12004,#12005,#10076,.T.);
#15137=EDGE_CURVE('',#12005,#12006,#6677,.T.);
#15138=EDGE_CURVE('',#12006,#12007,#10077,.T.);
#15139=EDGE_CURVE('',#12007,#12008,#6678,.T.);
#15140=EDGE_CURVE('',#12008,#12009,#10078,.T.);
#15141=EDGE_CURVE('',#12009,#12010,#10079,.T.);
#15142=EDGE_CURVE('',#12010,#12011,#10080,.T.);
#15143=EDGE_CURVE('',#12011,#12012,#6679,.T.);
#15144=EDGE_CURVE('',#12012,#12013,#10081,.T.);
#15145=EDGE_CURVE('',#12013,#12014,#6680,.T.);
#15146=EDGE_CURVE('',#12014,#12015,#10082,.T.);
#15147=EDGE_CURVE('',#12015,#12016,#6681,.T.);
#15148=EDGE_CURVE('',#12016,#12017,#10083,.T.);
#15149=EDGE_CURVE('',#12017,#12018,#10084,.T.);
#15150=EDGE_CURVE('',#12018,#12019,#10085,.T.);
#15151=EDGE_CURVE('',#12019,#12020,#6682,.T.);
#15152=EDGE_CURVE('',#12020,#12021,#6683,.T.);
#15153=EDGE_CURVE('',#12021,#12022,#6684,.T.);
#15154=EDGE_CURVE('',#12022,#12023,#10086,.T.);
#15155=EDGE_CURVE('',#12023,#12024,#10087,.T.);
#15156=EDGE_CURVE('',#12024,#12025,#10088,.T.);
#15157=EDGE_CURVE('',#12025,#12026,#6685,.T.);
#15158=EDGE_CURVE('',#12026,#12027,#10089,.T.);
#15159=EDGE_CURVE('',#12027,#12028,#6686,.T.);
#15160=EDGE_CURVE('',#12028,#12029,#10090,.T.);
#15161=EDGE_CURVE('',#12029,#12030,#6687,.T.);
#15162=EDGE_CURVE('',#12030,#12031,#10091,.T.);
#15163=EDGE_CURVE('',#12031,#12032,#10092,.T.);
#15164=EDGE_CURVE('',#12032,#12033,#10093,.T.);
#15165=EDGE_CURVE('',#12033,#12034,#6688,.T.);
#15166=EDGE_CURVE('',#12034,#12035,#10094,.T.);
#15167=EDGE_CURVE('',#12035,#12036,#6689,.T.);
#15168=EDGE_CURVE('',#12036,#12037,#10095,.T.);
#15169=EDGE_CURVE('',#12037,#11994,#6690,.T.);
#15170=EDGE_CURVE('',#11992,#12038,#6691,.T.);
#15171=EDGE_CURVE('',#12038,#11974,#6692,.T.);
#15172=EDGE_CURVE('',#12039,#11984,#6693,.T.);
#15173=EDGE_CURVE('',#12039,#11973,#6694,.T.);
#15174=EDGE_CURVE('',#12040,#12041,#6695,.T.);
#15175=EDGE_CURVE('',#11981,#12041,#6696,.T.);
#15176=EDGE_CURVE('',#12039,#12040,#6697,.T.);
#15177=EDGE_CURVE('',#12040,#12042,#6698,.T.);
#15178=EDGE_CURVE('',#12042,#12043,#6699,.T.);
#15179=EDGE_CURVE('',#12043,#12041,#6700,.T.);
#15180=EDGE_CURVE('',#12044,#12038,#6701,.T.);
#15181=EDGE_CURVE('',#11993,#12045,#6702,.T.);
#15182=EDGE_CURVE('',#12045,#12044,#6703,.T.);
#15183=EDGE_CURVE('',#12045,#12046,#6704,.T.);
#15184=EDGE_CURVE('',#12046,#12047,#6705,.T.);
#15185=EDGE_CURVE('',#12044,#12047,#6706,.T.);
#15186=EDGE_CURVE('',#11682,#12043,#152,.T.);
#15187=EDGE_CURVE('',#11985,#11684,#153,.T.);
#15188=EDGE_CURVE('',#12048,#11988,#10096,.T.);
#15189=EDGE_CURVE('',#12049,#11992,#6707,.T.);
#15190=EDGE_CURVE('',#12049,#12050,#6708,.T.);
#15191=EDGE_CURVE('',#12048,#12050,#6709,.T.);
#15192=EDGE_CURVE('',#12051,#12052,#6710,.T.);
#15193=EDGE_CURVE('',#12052,#12048,#6711,.T.);
#15194=EDGE_CURVE('',#12050,#12051,#6712,.T.);
#15195=EDGE_CURVE('',#11685,#12053,#154,.T.);
#15196=EDGE_CURVE('',#12054,#11687,#6713,.T.);
#15197=EDGE_CURVE('',#12053,#12054,#6714,.T.);
#15198=EDGE_CURVE('',#12055,#12056,#6715,.T.);
#15199=EDGE_CURVE('',#12055,#12053,#6716,.T.);
#15200=EDGE_CURVE('',#12054,#12056,#6717,.T.);
#15201=EDGE_CURVE('',#12056,#12057,#6718,.T.);
#15202=EDGE_CURVE('',#11984,#12057,#6719,.T.);
#15203=EDGE_CURVE('',#11986,#12055,#10097,.T.);
#15204=EDGE_CURVE('',#12052,#12058,#155,.T.);
#15205=EDGE_CURVE('',#12059,#12051,#6720,.T.);
#15206=EDGE_CURVE('',#12058,#12059,#6721,.T.);
#15207=EDGE_CURVE('',#12046,#11678,#156,.T.);
#15208=EDGE_CURVE('',#11679,#11989,#157,.T.);
#15209=EDGE_CURVE('',#12060,#12061,#6722,.T.);
#15210=EDGE_CURVE('',#11995,#12061,#6723,.T.);
#15211=EDGE_CURVE('',#11994,#12060,#6724,.T.);
#15212=EDGE_CURVE('',#12061,#12062,#6725,.T.);
#15213=EDGE_CURVE('',#11996,#12062,#6726,.T.);
#15214=EDGE_CURVE('',#12062,#12063,#6727,.T.);
#15215=EDGE_CURVE('',#11997,#12063,#6728,.T.);
#15216=EDGE_CURVE('',#12063,#12064,#6729,.T.);
#15217=EDGE_CURVE('',#11998,#12064,#6730,.T.);
#15218=EDGE_CURVE('',#12064,#12065,#6731,.T.);
#15219=EDGE_CURVE('',#11999,#12065,#6732,.T.);
#15220=EDGE_CURVE('',#12065,#12066,#6733,.T.);
#15221=EDGE_CURVE('',#12000,#12066,#6734,.T.);
#15222=EDGE_CURVE('',#12066,#12067,#6735,.T.);
#15223=EDGE_CURVE('',#12001,#12067,#6736,.T.);
#15224=EDGE_CURVE('',#12067,#12068,#6737,.T.);
#15225=EDGE_CURVE('',#12002,#12068,#6738,.T.);
#15226=EDGE_CURVE('',#12068,#12069,#6739,.T.);
#15227=EDGE_CURVE('',#12003,#12069,#6740,.T.);
#15228=EDGE_CURVE('',#12069,#12070,#6741,.T.);
#15229=EDGE_CURVE('',#12004,#12070,#6742,.T.);
#15230=EDGE_CURVE('',#12070,#12071,#10098,.T.);
#15231=EDGE_CURVE('',#12005,#12071,#6743,.T.);
#15232=EDGE_CURVE('',#12071,#12072,#6744,.T.);
#15233=EDGE_CURVE('',#12006,#12072,#6745,.T.);
#15234=EDGE_CURVE('',#12072,#12073,#10099,.T.);
#15235=EDGE_CURVE('',#12007,#12073,#6746,.T.);
#15236=EDGE_CURVE('',#12073,#12074,#6747,.T.);
#15237=EDGE_CURVE('',#12008,#12074,#6748,.T.);
#15238=EDGE_CURVE('',#12074,#12075,#10100,.T.);
#15239=EDGE_CURVE('',#12009,#12075,#6749,.T.);
#15240=EDGE_CURVE('',#12075,#12076,#10101,.T.);
#15241=EDGE_CURVE('',#12010,#12076,#6750,.T.);
#15242=EDGE_CURVE('',#12076,#12077,#10102,.T.);
#15243=EDGE_CURVE('',#12011,#12077,#6751,.T.);
#15244=EDGE_CURVE('',#12077,#12078,#6752,.T.);
#15245=EDGE_CURVE('',#12012,#12078,#6753,.T.);
#15246=EDGE_CURVE('',#12078,#12079,#10103,.T.);
#15247=EDGE_CURVE('',#12013,#12079,#6754,.T.);
#15248=EDGE_CURVE('',#12079,#12080,#6755,.T.);
#15249=EDGE_CURVE('',#12014,#12080,#6756,.T.);
#15250=EDGE_CURVE('',#12080,#12081,#10104,.T.);
#15251=EDGE_CURVE('',#12015,#12081,#6757,.T.);
#15252=EDGE_CURVE('',#12081,#12082,#6758,.T.);
#15253=EDGE_CURVE('',#12016,#12082,#6759,.T.);
#15254=EDGE_CURVE('',#12082,#12083,#10105,.T.);
#15255=EDGE_CURVE('',#12017,#12083,#6760,.T.);
#15256=EDGE_CURVE('',#12083,#12084,#10106,.T.);
#15257=EDGE_CURVE('',#12018,#12084,#6761,.T.);
#15258=EDGE_CURVE('',#12084,#12085,#10107,.T.);
#15259=EDGE_CURVE('',#12019,#12085,#6762,.T.);
#15260=EDGE_CURVE('',#12085,#12086,#6763,.T.);
#15261=EDGE_CURVE('',#12020,#12086,#6764,.T.);
#15262=EDGE_CURVE('',#12086,#12087,#6765,.T.);
#15263=EDGE_CURVE('',#12021,#12087,#6766,.T.);
#15264=EDGE_CURVE('',#12087,#12088,#6767,.T.);
#15265=EDGE_CURVE('',#12022,#12088,#6768,.T.);
#15266=EDGE_CURVE('',#12088,#12089,#10108,.T.);
#15267=EDGE_CURVE('',#12023,#12089,#6769,.T.);
#15268=EDGE_CURVE('',#12089,#12090,#10109,.T.);
#15269=EDGE_CURVE('',#12024,#12090,#6770,.T.);
#15270=EDGE_CURVE('',#12090,#12091,#10110,.T.);
#15271=EDGE_CURVE('',#12025,#12091,#6771,.T.);
#15272=EDGE_CURVE('',#12091,#12092,#6772,.T.);
#15273=EDGE_CURVE('',#12026,#12092,#6773,.T.);
#15274=EDGE_CURVE('',#12092,#12093,#10111,.T.);
#15275=EDGE_CURVE('',#12027,#12093,#6774,.T.);
#15276=EDGE_CURVE('',#12093,#12094,#6775,.T.);
#15277=EDGE_CURVE('',#12028,#12094,#6776,.T.);
#15278=EDGE_CURVE('',#12094,#12095,#10112,.T.);
#15279=EDGE_CURVE('',#12029,#12095,#6777,.T.);
#15280=EDGE_CURVE('',#12095,#12096,#6778,.T.);
#15281=EDGE_CURVE('',#12030,#12096,#6779,.T.);
#15282=EDGE_CURVE('',#12096,#12097,#10113,.T.);
#15283=EDGE_CURVE('',#12031,#12097,#6780,.T.);
#15284=EDGE_CURVE('',#12097,#12098,#10114,.T.);
#15285=EDGE_CURVE('',#12032,#12098,#6781,.T.);
#15286=EDGE_CURVE('',#12098,#12099,#10115,.T.);
#15287=EDGE_CURVE('',#12033,#12099,#6782,.T.);
#15288=EDGE_CURVE('',#12099,#12100,#6783,.T.);
#15289=EDGE_CURVE('',#12034,#12100,#6784,.T.);
#15290=EDGE_CURVE('',#12100,#12101,#10116,.T.);
#15291=EDGE_CURVE('',#12035,#12101,#6785,.T.);
#15292=EDGE_CURVE('',#12101,#12102,#6786,.T.);
#15293=EDGE_CURVE('',#12036,#12102,#6787,.T.);
#15294=EDGE_CURVE('',#12102,#12103,#10117,.T.);
#15295=EDGE_CURVE('',#12037,#12103,#6788,.T.);
#15296=EDGE_CURVE('',#12103,#12060,#6789,.T.);
#15297=EDGE_CURVE('',#12104,#12105,#6790,.T.);
#15298=EDGE_CURVE('',#12105,#12106,#6791,.T.);
#15299=EDGE_CURVE('',#12106,#12107,#6792,.T.);
#15300=EDGE_CURVE('',#12107,#12104,#6793,.T.);
#15301=EDGE_CURVE('',#12108,#12105,#6794,.T.);
#15302=EDGE_CURVE('',#12108,#12109,#6795,.T.);
#15303=EDGE_CURVE('',#12106,#12109,#6796,.T.);
#15304=EDGE_CURVE('',#12110,#12108,#6797,.T.);
#15305=EDGE_CURVE('',#12111,#12110,#6798,.T.);
#15306=EDGE_CURVE('',#12109,#12111,#6799,.T.);
#15307=EDGE_CURVE('',#12112,#12110,#6800,.T.);
#15308=EDGE_CURVE('',#12113,#12112,#6801,.T.);
#15309=EDGE_CURVE('',#12111,#12113,#6802,.T.);
#15310=EDGE_CURVE('',#12114,#12112,#6803,.T.);
#15311=EDGE_CURVE('',#12115,#12114,#6804,.T.);
#15312=EDGE_CURVE('',#12113,#12115,#6805,.T.);
#15313=EDGE_CURVE('',#12116,#12117,#6806,.T.);
#15314=EDGE_CURVE('',#12118,#12116,#6807,.T.);
#15315=EDGE_CURVE('',#12119,#12118,#6808,.T.);
#15316=EDGE_CURVE('',#12119,#12117,#6809,.T.);
#15317=EDGE_CURVE('',#12120,#12116,#6810,.T.);
#15318=EDGE_CURVE('',#12121,#12120,#6811,.T.);
#15319=EDGE_CURVE('',#12118,#12121,#6812,.T.);
#15320=EDGE_CURVE('',#12122,#12120,#6813,.T.);
#15321=EDGE_CURVE('',#12123,#12122,#6814,.T.);
#15322=EDGE_CURVE('',#12121,#12123,#6815,.T.);
#15323=EDGE_CURVE('',#12123,#12107,#6816,.T.);
#15324=EDGE_CURVE('',#12104,#12122,#6817,.T.);
#15325=EDGE_CURVE('',#12049,#12124,#6818,.T.);
#15326=EDGE_CURVE('',#12038,#12125,#6819,.T.);
#15327=EDGE_CURVE('',#12125,#12126,#6820,.T.);
#15328=EDGE_CURVE('',#12126,#12124,#6821,.T.);
#15329=EDGE_CURVE('',#12126,#12127,#6822,.T.);
#15330=EDGE_CURVE('',#12127,#12128,#6823,.T.);
#15331=EDGE_CURVE('',#12124,#12128,#6824,.T.);
#15332=EDGE_CURVE('',#12129,#12130,#6825,.T.);
#15333=EDGE_CURVE('',#12128,#12130,#6826,.T.);
#15334=EDGE_CURVE('',#12127,#12129,#6827,.T.);
#15335=EDGE_CURVE('',#12131,#12132,#6828,.T.);
#15336=EDGE_CURVE('',#12132,#12130,#6829,.T.);
#15337=EDGE_CURVE('',#12131,#12129,#6830,.T.);
#15338=EDGE_CURVE('',#12133,#12134,#6831,.T.);
#15339=EDGE_CURVE('',#12134,#12132,#6832,.T.);
#15340=EDGE_CURVE('',#12133,#12131,#6833,.T.);
#15341=EDGE_CURVE('',#12135,#12136,#6834,.T.);
#15342=EDGE_CURVE('',#12136,#12134,#6835,.T.);
#15343=EDGE_CURVE('',#12135,#12133,#6836,.T.);
#15344=EDGE_CURVE('',#12135,#12137,#6837,.T.);
#15345=EDGE_CURVE('',#12137,#12138,#6838,.T.);
#15346=EDGE_CURVE('',#12136,#12138,#6839,.T.);
#15347=EDGE_CURVE('',#12139,#12140,#6840,.T.);
#15348=EDGE_CURVE('',#12140,#12138,#6841,.T.);
#15349=EDGE_CURVE('',#12139,#12137,#6842,.T.);
#15350=EDGE_CURVE('',#12141,#12142,#6843,.T.);
#15351=EDGE_CURVE('',#12142,#12140,#6844,.T.);
#15352=EDGE_CURVE('',#12141,#12139,#6845,.T.);
#15353=EDGE_CURVE('',#12143,#12144,#6846,.T.);
#15354=EDGE_CURVE('',#12144,#12142,#6847,.T.);
#15355=EDGE_CURVE('',#12143,#12141,#6848,.T.);
#15356=EDGE_CURVE('',#12143,#12145,#6849,.T.);
#15357=EDGE_CURVE('',#12145,#12146,#6850,.T.);
#15358=EDGE_CURVE('',#12144,#12146,#6851,.T.);
#15359=EDGE_CURVE('',#12145,#12147,#6852,.T.);
#15360=EDGE_CURVE('',#12147,#12148,#6853,.T.);
#15361=EDGE_CURVE('',#12146,#12148,#6854,.T.);
#15362=EDGE_CURVE('',#12147,#12149,#6855,.T.);
#15363=EDGE_CURVE('',#12149,#12150,#6856,.T.);
#15364=EDGE_CURVE('',#12148,#12150,#6857,.T.);
#15365=EDGE_CURVE('',#12149,#12151,#6858,.T.);
#15366=EDGE_CURVE('',#12151,#12152,#6859,.T.);
#15367=EDGE_CURVE('',#12150,#12152,#6860,.T.);
#15368=EDGE_CURVE('',#12151,#12153,#6861,.T.);
#15369=EDGE_CURVE('',#12153,#12039,#6862,.T.);
#15370=EDGE_CURVE('',#12152,#12057,#6863,.T.);
#15371=EDGE_CURVE('',#12154,#12042,#10118,.T.);
#15372=EDGE_CURVE('',#12153,#12155,#6864,.T.);
#15373=EDGE_CURVE('',#12154,#12155,#6865,.T.);
#15374=EDGE_CURVE('',#12156,#12157,#6866,.T.);
#15375=EDGE_CURVE('',#12157,#12154,#6867,.T.);
#15376=EDGE_CURVE('',#12155,#12156,#6868,.T.);
#15377=EDGE_CURVE('',#12157,#12158,#158,.T.);
#15378=EDGE_CURVE('',#12156,#12159,#6869,.T.);
#15379=EDGE_CURVE('',#12159,#12158,#6870,.T.);
#15380=EDGE_CURVE('',#11675,#12160,#159,.T.);
#15381=EDGE_CURVE('',#11677,#12161,#6871,.T.);
#15382=EDGE_CURVE('',#12160,#12161,#6872,.T.);
#15383=EDGE_CURVE('',#12162,#12163,#6873,.T.);
#15384=EDGE_CURVE('',#12162,#12160,#6874,.T.);
#15385=EDGE_CURVE('',#12161,#12163,#6875,.T.);
#15386=EDGE_CURVE('',#12163,#12125,#6876,.T.);
#15387=EDGE_CURVE('',#12047,#12162,#10119,.T.);
#15388=EDGE_CURVE('',#12158,#11681,#160,.T.);
#15389=EDGE_CURVE('',#12159,#12164,#6877,.T.);
#15390=EDGE_CURVE('',#12164,#11681,#6878,.T.);
#15391=EDGE_CURVE('',#12117,#12165,#6879,.T.);
#15392=EDGE_CURVE('',#12166,#12119,#6880,.T.);
#15393=EDGE_CURVE('',#12166,#12165,#6881,.T.);
#15394=EDGE_CURVE('',#12167,#12114,#6882,.T.);
#15395=EDGE_CURVE('',#12168,#12167,#6883,.T.);
#15396=EDGE_CURVE('',#12115,#12168,#6884,.T.);
#15397=EDGE_CURVE('',#11686,#12166,#6885,.T.);
#15398=EDGE_CURVE('',#12168,#12169,#6886,.T.);
#15399=EDGE_CURVE('',#12169,#12059,#6887,.T.);
#15400=EDGE_CURVE('',#12058,#11680,#161,.T.);
#15401=EDGE_CURVE('',#11680,#12169,#6888,.T.);
#15402=EDGE_CURVE('',#12165,#12170,#6889,.T.);
#15403=EDGE_CURVE('',#12170,#12171,#6890,.T.);
#15404=EDGE_CURVE('',#12171,#12172,#10120,.T.);
#15405=EDGE_CURVE('',#12172,#12173,#6891,.T.);
#15406=EDGE_CURVE('',#12173,#12174,#10121,.T.);
#15407=EDGE_CURVE('',#12174,#12175,#6892,.T.);
#15408=EDGE_CURVE('',#12175,#12176,#10122,.T.);
#15409=EDGE_CURVE('',#12176,#12177,#10123,.T.);
#15410=EDGE_CURVE('',#12177,#12178,#10124,.T.);
#15411=EDGE_CURVE('',#12178,#12179,#6893,.T.);
#15412=EDGE_CURVE('',#12179,#12180,#10125,.T.);
#15413=EDGE_CURVE('',#12180,#12181,#6894,.T.);
#15414=EDGE_CURVE('',#12181,#12182,#10126,.T.);
#15415=EDGE_CURVE('',#12182,#12183,#6895,.T.);
#15416=EDGE_CURVE('',#12183,#12184,#10127,.T.);
#15417=EDGE_CURVE('',#12184,#12185,#10128,.T.);
#15418=EDGE_CURVE('',#12185,#12186,#10129,.T.);
#15419=EDGE_CURVE('',#12186,#12187,#6896,.T.);
#15420=EDGE_CURVE('',#12187,#12188,#6897,.T.);
#15421=EDGE_CURVE('',#12188,#12189,#6898,.T.);
#15422=EDGE_CURVE('',#12189,#12190,#10130,.T.);
#15423=EDGE_CURVE('',#12190,#12191,#10131,.T.);
#15424=EDGE_CURVE('',#12191,#12192,#10132,.T.);
#15425=EDGE_CURVE('',#12192,#12193,#6899,.T.);
#15426=EDGE_CURVE('',#12193,#12194,#10133,.T.);
#15427=EDGE_CURVE('',#12194,#12195,#6900,.T.);
#15428=EDGE_CURVE('',#12195,#12196,#10134,.T.);
#15429=EDGE_CURVE('',#12196,#12197,#6901,.T.);
#15430=EDGE_CURVE('',#12197,#12198,#10135,.T.);
#15431=EDGE_CURVE('',#12198,#12199,#10136,.T.);
#15432=EDGE_CURVE('',#12199,#12200,#10137,.T.);
#15433=EDGE_CURVE('',#12200,#12201,#6902,.T.);
#15434=EDGE_CURVE('',#12201,#12202,#10138,.T.);
#15435=EDGE_CURVE('',#12202,#12203,#6903,.T.);
#15436=EDGE_CURVE('',#12203,#12204,#10139,.T.);
#15437=EDGE_CURVE('',#12204,#12205,#6904,.T.);
#15438=EDGE_CURVE('',#12205,#12167,#6905,.T.);
#15439=EDGE_CURVE('',#12206,#11676,#6906,.T.);
#15440=EDGE_CURVE('',#12207,#12206,#6907,.T.);
#15441=EDGE_CURVE('',#12208,#12207,#6908,.T.);
#15442=EDGE_CURVE('',#12209,#12208,#6909,.T.);
#15443=EDGE_CURVE('',#12210,#12209,#6910,.T.);
#15444=EDGE_CURVE('',#12210,#12211,#6911,.T.);
#15445=EDGE_CURVE('',#12212,#12211,#6912,.T.);
#15446=EDGE_CURVE('',#12212,#12213,#6913,.T.);
#15447=EDGE_CURVE('',#12214,#12213,#6914,.T.);
#15448=EDGE_CURVE('',#12215,#12214,#6915,.T.);
#15449=EDGE_CURVE('',#12216,#12215,#6916,.T.);
#15450=EDGE_CURVE('',#12217,#12216,#6917,.T.);
#15451=EDGE_CURVE('',#12164,#12217,#6918,.T.);
#15452=EDGE_CURVE('',#12218,#12219,#6919,.T.);
#15453=EDGE_CURVE('',#12218,#12213,#6920,.T.);
#15454=EDGE_CURVE('',#12219,#12212,#6921,.T.);
#15455=EDGE_CURVE('',#12220,#12221,#6922,.T.);
#15456=EDGE_CURVE('',#12221,#12209,#6923,.T.);
#15457=EDGE_CURVE('',#12220,#12208,#6924,.T.);
#15458=EDGE_CURVE('',#12222,#12220,#6925,.T.);
#15459=EDGE_CURVE('',#12222,#12207,#6926,.T.);
#15460=EDGE_CURVE('',#12223,#12222,#6927,.T.);
#15461=EDGE_CURVE('',#12223,#12206,#6928,.T.);
#15462=EDGE_CURVE('',#12221,#12224,#6929,.T.);
#15463=EDGE_CURVE('',#12210,#12224,#6930,.T.);
#15464=EDGE_CURVE('',#12225,#12203,#6931,.T.);
#15465=EDGE_CURVE('',#12225,#12226,#10140,.T.);
#15466=EDGE_CURVE('',#12204,#12226,#6932,.T.);
#15467=EDGE_CURVE('',#12227,#12201,#6933,.T.);
#15468=EDGE_CURVE('',#12227,#12228,#10141,.T.);
#15469=EDGE_CURVE('',#12202,#12228,#6934,.T.);
#15470=EDGE_CURVE('',#12228,#12225,#6935,.T.);
#15471=EDGE_CURVE('',#12226,#12229,#6936,.T.);
#15472=EDGE_CURVE('',#12229,#12205,#6937,.T.);
#15473=EDGE_CURVE('',#12229,#12223,#6938,.T.);
#15474=EDGE_CURVE('',#12230,#12231,#10142,.T.);
#15475=EDGE_CURVE('',#12200,#12231,#6939,.T.);
#15476=EDGE_CURVE('',#12230,#12199,#6940,.T.);
#15477=EDGE_CURVE('',#12232,#12233,#10143,.T.);
#15478=EDGE_CURVE('',#12198,#12233,#6941,.T.);
#15479=EDGE_CURVE('',#12232,#12197,#6942,.T.);
#15480=EDGE_CURVE('',#12233,#12230,#10144,.T.);
#15481=EDGE_CURVE('',#12234,#12235,#10145,.T.);
#15482=EDGE_CURVE('',#12196,#12235,#6943,.T.);
#15483=EDGE_CURVE('',#12234,#12195,#6944,.T.);
#15484=EDGE_CURVE('',#12236,#12237,#10146,.T.);
#15485=EDGE_CURVE('',#12194,#12237,#6945,.T.);
#15486=EDGE_CURVE('',#12236,#12193,#6946,.T.);
#15487=EDGE_CURVE('',#12237,#12234,#6947,.T.);
#15488=EDGE_CURVE('',#12235,#12232,#6948,.T.);
#15489=EDGE_CURVE('',#12238,#12239,#10147,.T.);
#15490=EDGE_CURVE('',#12192,#12239,#6949,.T.);
#15491=EDGE_CURVE('',#12238,#12191,#6950,.T.);
#15492=EDGE_CURVE('',#12240,#12241,#10148,.T.);
#15493=EDGE_CURVE('',#12190,#12241,#6951,.T.);
#15494=EDGE_CURVE('',#12240,#12189,#6952,.T.);
#15495=EDGE_CURVE('',#12241,#12238,#10149,.T.);
#15496=EDGE_CURVE('',#12242,#12187,#6953,.T.);
#15497=EDGE_CURVE('',#12242,#12243,#6954,.T.);
#15498=EDGE_CURVE('',#12243,#12188,#6955,.T.);
#15499=EDGE_CURVE('',#12243,#12240,#6956,.T.);
#15500=EDGE_CURVE('',#12244,#12245,#10150,.T.);
#15501=EDGE_CURVE('',#12186,#12245,#6957,.T.);
#15502=EDGE_CURVE('',#12244,#12185,#6958,.T.);
#15503=EDGE_CURVE('',#12246,#12247,#10151,.T.);
#15504=EDGE_CURVE('',#12184,#12247,#6959,.T.);
#15505=EDGE_CURVE('',#12246,#12183,#6960,.T.);
#15506=EDGE_CURVE('',#12247,#12244,#10152,.T.);
#15507=EDGE_CURVE('',#12248,#12249,#10153,.T.);
#15508=EDGE_CURVE('',#12182,#12249,#6961,.T.);
#15509=EDGE_CURVE('',#12248,#12181,#6962,.T.);
#15510=EDGE_CURVE('',#12250,#12251,#10154,.T.);
#15511=EDGE_CURVE('',#12180,#12251,#6963,.T.);
#15512=EDGE_CURVE('',#12250,#12179,#6964,.T.);
#15513=EDGE_CURVE('',#12251,#12248,#6965,.T.);
#15514=EDGE_CURVE('',#12249,#12246,#6966,.T.);
#15515=EDGE_CURVE('',#12245,#12242,#6967,.T.);
#15516=EDGE_CURVE('',#12252,#12253,#10155,.T.);
#15517=EDGE_CURVE('',#12178,#12253,#6968,.T.);
#15518=EDGE_CURVE('',#12252,#12177,#6969,.T.);
#15519=EDGE_CURVE('',#12254,#12255,#10156,.T.);
#15520=EDGE_CURVE('',#12176,#12255,#6970,.T.);
#15521=EDGE_CURVE('',#12254,#12175,#6971,.T.);
#15522=EDGE_CURVE('',#12255,#12252,#10157,.T.);
#15523=EDGE_CURVE('',#12256,#12173,#6972,.T.);
#15524=EDGE_CURVE('',#12256,#12257,#10158,.T.);
#15525=EDGE_CURVE('',#12174,#12257,#6973,.T.);
#15526=EDGE_CURVE('',#12258,#12171,#6974,.T.);
#15527=EDGE_CURVE('',#12258,#12259,#10159,.T.);
#15528=EDGE_CURVE('',#12172,#12259,#6975,.T.);
#15529=EDGE_CURVE('',#12260,#12261,#6976,.T.);
#15530=EDGE_CURVE('',#12261,#12217,#6977,.T.);
#15531=EDGE_CURVE('',#12260,#12216,#6978,.T.);
#15532=EDGE_CURVE('',#12262,#12260,#6979,.T.);
#15533=EDGE_CURVE('',#12262,#12215,#6980,.T.);
#15534=EDGE_CURVE('',#12263,#12262,#6981,.T.);
#15535=EDGE_CURVE('',#12263,#12214,#6982,.T.);
#15536=EDGE_CURVE('',#12218,#12263,#6983,.T.);
#15537=EDGE_CURVE('',#12261,#12264,#6984,.T.);
#15538=EDGE_CURVE('',#12264,#12170,#6985,.T.);
#15539=EDGE_CURVE('',#12264,#12258,#6986,.T.);
#15540=EDGE_CURVE('',#12259,#12256,#6987,.T.);
#15541=EDGE_CURVE('',#12257,#12254,#6988,.T.);
#15542=EDGE_CURVE('',#12253,#12250,#6989,.T.);
#15543=EDGE_CURVE('',#12239,#12236,#6990,.T.);
#15544=EDGE_CURVE('',#12231,#12227,#6991,.T.);
#15545=EDGE_CURVE('',#12265,#12224,#6992,.T.);
#15546=EDGE_CURVE('',#12211,#12265,#6993,.T.);
#15547=EDGE_CURVE('',#12265,#12219,#6994,.T.);
#15548=EDGE_CURVE('',#12266,#11929,#6995,.T.);
#15549=EDGE_CURVE('',#12266,#11874,#6996,.T.);
#15550=EDGE_CURVE('',#12267,#12266,#10160,.T.);
#15551=EDGE_CURVE('',#12267,#11875,#6997,.T.);
#15552=EDGE_CURVE('',#11930,#12267,#6998,.T.);
#20092=ORIENTED_EDGE('',*,*,#14591,.F.);
#20093=ORIENTED_EDGE('',*,*,#14592,.T.);
#20094=ORIENTED_EDGE('',*,*,#14593,.T.);
#20095=ORIENTED_EDGE('',*,*,#14592,.F.);
#20096=ORIENTED_EDGE('',*,*,#14594,.F.);
#20097=ORIENTED_EDGE('',*,*,#14595,.T.);
#20098=ORIENTED_EDGE('',*,*,#14596,.T.);
#20099=ORIENTED_EDGE('',*,*,#14595,.F.);
#20100=ORIENTED_EDGE('',*,*,#14597,.F.);
#20101=ORIENTED_EDGE('',*,*,#14598,.T.);
#20102=ORIENTED_EDGE('',*,*,#14599,.T.);
#20103=ORIENTED_EDGE('',*,*,#14598,.F.);
#20104=ORIENTED_EDGE('',*,*,#14600,.T.);
#20105=ORIENTED_EDGE('',*,*,#14591,.T.);
#20106=ORIENTED_EDGE('',*,*,#14600,.F.);
#20107=ORIENTED_EDGE('',*,*,#14601,.T.);
#20108=ORIENTED_EDGE('',*,*,#14594,.T.);
#20109=ORIENTED_EDGE('',*,*,#14601,.F.);
#20110=ORIENTED_EDGE('',*,*,#14602,.F.);
#20111=ORIENTED_EDGE('',*,*,#14603,.T.);
#20112=ORIENTED_EDGE('',*,*,#14604,.T.);
#20113=ORIENTED_EDGE('',*,*,#14603,.F.);
#20114=ORIENTED_EDGE('',*,*,#14605,.F.);
#20115=ORIENTED_EDGE('',*,*,#14606,.T.);
#20116=ORIENTED_EDGE('',*,*,#14607,.T.);
#20117=ORIENTED_EDGE('',*,*,#14606,.F.);
#20118=ORIENTED_EDGE('',*,*,#14608,.F.);
#20119=ORIENTED_EDGE('',*,*,#14609,.T.);
#20120=ORIENTED_EDGE('',*,*,#14610,.T.);
#20121=ORIENTED_EDGE('',*,*,#14609,.F.);
#20122=ORIENTED_EDGE('',*,*,#14611,.F.);
#20123=ORIENTED_EDGE('',*,*,#14612,.T.);
#20124=ORIENTED_EDGE('',*,*,#14613,.T.);
#20125=ORIENTED_EDGE('',*,*,#14612,.F.);
#20126=ORIENTED_EDGE('',*,*,#14614,.F.);
#20127=ORIENTED_EDGE('',*,*,#14615,.T.);
#20128=ORIENTED_EDGE('',*,*,#14616,.T.);
#20129=ORIENTED_EDGE('',*,*,#14615,.F.);
#20130=ORIENTED_EDGE('',*,*,#14617,.F.);
#20131=ORIENTED_EDGE('',*,*,#14618,.T.);
#20132=ORIENTED_EDGE('',*,*,#14619,.T.);
#20133=ORIENTED_EDGE('',*,*,#14618,.F.);
#20134=ORIENTED_EDGE('',*,*,#14620,.F.);
#20135=ORIENTED_EDGE('',*,*,#14621,.T.);
#20136=ORIENTED_EDGE('',*,*,#14622,.T.);
#20137=ORIENTED_EDGE('',*,*,#14621,.F.);
#20138=ORIENTED_EDGE('',*,*,#14623,.F.);
#20139=ORIENTED_EDGE('',*,*,#14624,.T.);
#20140=ORIENTED_EDGE('',*,*,#14625,.T.);
#20141=ORIENTED_EDGE('',*,*,#14626,.T.);
#20142=ORIENTED_EDGE('',*,*,#14627,.T.);
#20143=ORIENTED_EDGE('',*,*,#14628,.F.);
#20144=ORIENTED_EDGE('',*,*,#14624,.F.);
#20145=ORIENTED_EDGE('',*,*,#14629,.T.);
#20146=ORIENTED_EDGE('',*,*,#14614,.T.);
#20147=ORIENTED_EDGE('',*,*,#14629,.F.);
#20148=ORIENTED_EDGE('',*,*,#14630,.T.);
#20149=ORIENTED_EDGE('',*,*,#14617,.T.);
#20150=ORIENTED_EDGE('',*,*,#14630,.F.);
#20151=ORIENTED_EDGE('',*,*,#14631,.F.);
#20152=ORIENTED_EDGE('',*,*,#14632,.T.);
#20153=ORIENTED_EDGE('',*,*,#14633,.T.);
#20154=ORIENTED_EDGE('',*,*,#14634,.T.);
#20155=ORIENTED_EDGE('',*,*,#14635,.F.);
#20156=ORIENTED_EDGE('',*,*,#14636,.T.);
#20157=ORIENTED_EDGE('',*,*,#14632,.F.);
#20158=ORIENTED_EDGE('',*,*,#14637,.F.);
#20159=ORIENTED_EDGE('',*,*,#14638,.F.);
#20160=ORIENTED_EDGE('',*,*,#14639,.F.);
#20161=ORIENTED_EDGE('',*,*,#14640,.T.);
#20162=ORIENTED_EDGE('',*,*,#14641,.F.);
#20163=ORIENTED_EDGE('',*,*,#14642,.F.);
#20164=ORIENTED_EDGE('',*,*,#14640,.F.);
#20165=ORIENTED_EDGE('',*,*,#14643,.F.);
#20166=ORIENTED_EDGE('',*,*,#14644,.F.);
#20167=ORIENTED_EDGE('',*,*,#14645,.F.);
#20168=ORIENTED_EDGE('',*,*,#14646,.T.);
#20169=ORIENTED_EDGE('',*,*,#14647,.T.);
#20170=ORIENTED_EDGE('',*,*,#14641,.T.);
#20171=ORIENTED_EDGE('',*,*,#14642,.T.);
#20172=ORIENTED_EDGE('',*,*,#14647,.F.);
#20173=ORIENTED_EDGE('',*,*,#14648,.F.);
#20174=ORIENTED_EDGE('',*,*,#14649,.T.);
#20175=ORIENTED_EDGE('',*,*,#14650,.T.);
#20176=ORIENTED_EDGE('',*,*,#14649,.F.);
#20177=ORIENTED_EDGE('',*,*,#14651,.F.);
#20178=ORIENTED_EDGE('',*,*,#14652,.F.);
#20179=ORIENTED_EDGE('',*,*,#14653,.T.);
#20180=ORIENTED_EDGE('',*,*,#14654,.T.);
#20181=ORIENTED_EDGE('',*,*,#14655,.F.);
#20182=ORIENTED_EDGE('',*,*,#14656,.T.);
#20183=ORIENTED_EDGE('',*,*,#14657,.F.);
#20184=ORIENTED_EDGE('',*,*,#14658,.F.);
#20185=ORIENTED_EDGE('',*,*,#14659,.F.);
#20186=ORIENTED_EDGE('',*,*,#14660,.T.);
#20187=ORIENTED_EDGE('',*,*,#14661,.F.);
#20188=ORIENTED_EDGE('',*,*,#14662,.F.);
#20189=ORIENTED_EDGE('',*,*,#14663,.F.);
#20190=ORIENTED_EDGE('',*,*,#14664,.T.);
#20191=ORIENTED_EDGE('',*,*,#14665,.F.);
#20192=ORIENTED_EDGE('',*,*,#14666,.F.);
#20193=ORIENTED_EDGE('',*,*,#14667,.F.);
#20194=ORIENTED_EDGE('',*,*,#14668,.T.);
#20195=ORIENTED_EDGE('',*,*,#14669,.T.);
#20196=ORIENTED_EDGE('',*,*,#14670,.T.);
#20197=ORIENTED_EDGE('',*,*,#14671,.F.);
#20198=ORIENTED_EDGE('',*,*,#14672,.T.);
#20199=ORIENTED_EDGE('',*,*,#14673,.T.);
#20200=ORIENTED_EDGE('',*,*,#14674,.T.);
#20201=ORIENTED_EDGE('',*,*,#14675,.F.);
#20202=ORIENTED_EDGE('',*,*,#14676,.T.);
#20203=ORIENTED_EDGE('',*,*,#14677,.T.);
#20204=ORIENTED_EDGE('',*,*,#14678,.T.);
#20205=ORIENTED_EDGE('',*,*,#14679,.F.);
#20206=ORIENTED_EDGE('',*,*,#14680,.T.);
#20207=ORIENTED_EDGE('',*,*,#14681,.T.);
#20208=ORIENTED_EDGE('',*,*,#14682,.T.);
#20209=ORIENTED_EDGE('',*,*,#14683,.F.);
#20210=ORIENTED_EDGE('',*,*,#14684,.T.);
#20211=ORIENTED_EDGE('',*,*,#14685,.T.);
#20212=ORIENTED_EDGE('',*,*,#14686,.T.);
#20213=ORIENTED_EDGE('',*,*,#14687,.F.);
#20214=ORIENTED_EDGE('',*,*,#14688,.T.);
#20215=ORIENTED_EDGE('',*,*,#14689,.T.);
#20216=ORIENTED_EDGE('',*,*,#14690,.T.);
#20217=ORIENTED_EDGE('',*,*,#14691,.F.);
#20218=ORIENTED_EDGE('',*,*,#14692,.T.);
#20219=ORIENTED_EDGE('',*,*,#14693,.T.);
#20220=ORIENTED_EDGE('',*,*,#14694,.T.);
#20221=ORIENTED_EDGE('',*,*,#14695,.F.);
#20222=ORIENTED_EDGE('',*,*,#14696,.T.);
#20223=ORIENTED_EDGE('',*,*,#14697,.T.);
#20224=ORIENTED_EDGE('',*,*,#14698,.T.);
#20225=ORIENTED_EDGE('',*,*,#14699,.F.);
#20226=ORIENTED_EDGE('',*,*,#14700,.F.);
#20227=ORIENTED_EDGE('',*,*,#14701,.T.);
#20228=ORIENTED_EDGE('',*,*,#14702,.T.);
#20229=ORIENTED_EDGE('',*,*,#14703,.F.);
#20230=ORIENTED_EDGE('',*,*,#14704,.F.);
#20231=ORIENTED_EDGE('',*,*,#14705,.T.);
#20232=ORIENTED_EDGE('',*,*,#14700,.T.);
#20233=ORIENTED_EDGE('',*,*,#14706,.F.);
#20234=ORIENTED_EDGE('',*,*,#14707,.F.);
#20235=ORIENTED_EDGE('',*,*,#14708,.T.);
#20236=ORIENTED_EDGE('',*,*,#14709,.T.);
#20237=ORIENTED_EDGE('',*,*,#14710,.F.);
#20238=ORIENTED_EDGE('',*,*,#14711,.T.);
#20239=ORIENTED_EDGE('',*,*,#14712,.T.);
#20240=ORIENTED_EDGE('',*,*,#14707,.T.);
#20241=ORIENTED_EDGE('',*,*,#14713,.F.);
#20242=ORIENTED_EDGE('',*,*,#14714,.T.);
#20243=ORIENTED_EDGE('',*,*,#14715,.T.);
#20244=ORIENTED_EDGE('',*,*,#14716,.T.);
#20245=ORIENTED_EDGE('',*,*,#14717,.F.);
#20246=ORIENTED_EDGE('',*,*,#14718,.T.);
#20247=ORIENTED_EDGE('',*,*,#14719,.T.);
#20248=ORIENTED_EDGE('',*,*,#14720,.T.);
#20249=ORIENTED_EDGE('',*,*,#14721,.F.);
#20250=ORIENTED_EDGE('',*,*,#14722,.T.);
#20251=ORIENTED_EDGE('',*,*,#14723,.T.);
#20252=ORIENTED_EDGE('',*,*,#14724,.T.);
#20253=ORIENTED_EDGE('',*,*,#14725,.F.);
#20254=ORIENTED_EDGE('',*,*,#14726,.F.);
#20255=ORIENTED_EDGE('',*,*,#14727,.T.);
#20256=ORIENTED_EDGE('',*,*,#14728,.T.);
#20257=ORIENTED_EDGE('',*,*,#14729,.F.);
#20258=ORIENTED_EDGE('',*,*,#14682,.F.);
#20259=ORIENTED_EDGE('',*,*,#14730,.T.);
#20260=ORIENTED_EDGE('',*,*,#14726,.T.);
#20261=ORIENTED_EDGE('',*,*,#14731,.F.);
#20262=ORIENTED_EDGE('',*,*,#14732,.T.);
#20263=ORIENTED_EDGE('',*,*,#14733,.T.);
#20264=ORIENTED_EDGE('',*,*,#14734,.T.);
#20265=ORIENTED_EDGE('',*,*,#14735,.F.);
#20266=ORIENTED_EDGE('',*,*,#14736,.T.);
#20267=ORIENTED_EDGE('',*,*,#14737,.T.);
#20268=ORIENTED_EDGE('',*,*,#14738,.T.);
#20269=ORIENTED_EDGE('',*,*,#14739,.F.);
#20270=ORIENTED_EDGE('',*,*,#14740,.T.);
#20271=ORIENTED_EDGE('',*,*,#14741,.T.);
#20272=ORIENTED_EDGE('',*,*,#14742,.T.);
#20273=ORIENTED_EDGE('',*,*,#14743,.F.);
#20274=ORIENTED_EDGE('',*,*,#14744,.T.);
#20275=ORIENTED_EDGE('',*,*,#14745,.T.);
#20276=ORIENTED_EDGE('',*,*,#14746,.T.);
#20277=ORIENTED_EDGE('',*,*,#14747,.F.);
#20278=ORIENTED_EDGE('',*,*,#14716,.F.);
#20279=ORIENTED_EDGE('',*,*,#14748,.F.);
#20280=ORIENTED_EDGE('',*,*,#14711,.F.);
#20281=ORIENTED_EDGE('',*,*,#14749,.F.);
#20282=ORIENTED_EDGE('',*,*,#14702,.F.);
#20283=ORIENTED_EDGE('',*,*,#14750,.F.);
#20284=ORIENTED_EDGE('',*,*,#14696,.F.);
#20285=ORIENTED_EDGE('',*,*,#14718,.F.);
#20286=ORIENTED_EDGE('',*,*,#14751,.F.);
#20287=ORIENTED_EDGE('',*,*,#14724,.F.);
#20288=ORIENTED_EDGE('',*,*,#14752,.F.);
#20289=ORIENTED_EDGE('',*,*,#14722,.F.);
#20290=ORIENTED_EDGE('',*,*,#14753,.F.);
#20291=ORIENTED_EDGE('',*,*,#14674,.F.);
#20292=ORIENTED_EDGE('',*,*,#14754,.F.);
#20293=ORIENTED_EDGE('',*,*,#14672,.F.);
#20294=ORIENTED_EDGE('',*,*,#14755,.F.);
#20295=ORIENTED_EDGE('',*,*,#14742,.F.);
#20296=ORIENTED_EDGE('',*,*,#14756,.F.);
#20297=ORIENTED_EDGE('',*,*,#14740,.F.);
#20298=ORIENTED_EDGE('',*,*,#14757,.F.);
#20299=ORIENTED_EDGE('',*,*,#14728,.F.);
#20300=ORIENTED_EDGE('',*,*,#14758,.F.);
#20301=ORIENTED_EDGE('',*,*,#14744,.F.);
#20302=ORIENTED_EDGE('',*,*,#14759,.F.);
#20303=ORIENTED_EDGE('',*,*,#14720,.F.);
#20304=ORIENTED_EDGE('',*,*,#14760,.F.);
#20305=ORIENTED_EDGE('',*,*,#14668,.F.);
#20306=ORIENTED_EDGE('',*,*,#14761,.F.);
#20307=ORIENTED_EDGE('',*,*,#14746,.F.);
#20308=ORIENTED_EDGE('',*,*,#14762,.F.);
#20309=ORIENTED_EDGE('',*,*,#14763,.F.);
#20310=ORIENTED_EDGE('',*,*,#14670,.F.);
#20311=ORIENTED_EDGE('',*,*,#14764,.F.);
#20312=ORIENTED_EDGE('',*,*,#14714,.F.);
#20313=ORIENTED_EDGE('',*,*,#14765,.F.);
#20314=ORIENTED_EDGE('',*,*,#14698,.F.);
#20315=ORIENTED_EDGE('',*,*,#14766,.F.);
#20316=ORIENTED_EDGE('',*,*,#14692,.F.);
#20317=ORIENTED_EDGE('',*,*,#14736,.F.);
#20318=ORIENTED_EDGE('',*,*,#14767,.F.);
#20319=ORIENTED_EDGE('',*,*,#14694,.F.);
#20320=ORIENTED_EDGE('',*,*,#14768,.F.);
#20321=ORIENTED_EDGE('',*,*,#14676,.F.);
#20322=ORIENTED_EDGE('',*,*,#14769,.F.);
#20323=ORIENTED_EDGE('',*,*,#14738,.F.);
#20324=ORIENTED_EDGE('',*,*,#14770,.F.);
#20325=ORIENTED_EDGE('',*,*,#14688,.F.);
#20326=ORIENTED_EDGE('',*,*,#14771,.F.);
#20327=ORIENTED_EDGE('',*,*,#14678,.F.);
#20328=ORIENTED_EDGE('',*,*,#14772,.F.);
#20329=ORIENTED_EDGE('',*,*,#14684,.F.);
#20330=ORIENTED_EDGE('',*,*,#14773,.F.);
#20331=ORIENTED_EDGE('',*,*,#14690,.F.);
#20332=ORIENTED_EDGE('',*,*,#14774,.F.);
#20333=ORIENTED_EDGE('',*,*,#14732,.F.);
#20334=ORIENTED_EDGE('',*,*,#14775,.F.);
#20335=ORIENTED_EDGE('',*,*,#14686,.F.);
#20336=ORIENTED_EDGE('',*,*,#14776,.F.);
#20337=ORIENTED_EDGE('',*,*,#14680,.F.);
#20338=ORIENTED_EDGE('',*,*,#14777,.F.);
#20339=ORIENTED_EDGE('',*,*,#14734,.F.);
#20340=ORIENTED_EDGE('',*,*,#14778,.F.);
#20341=ORIENTED_EDGE('',*,*,#14648,.T.);
#20342=ORIENTED_EDGE('',*,*,#14646,.F.);
#20343=ORIENTED_EDGE('',*,*,#14779,.T.);
#20344=ORIENTED_EDGE('',*,*,#14780,.F.);
#20345=ORIENTED_EDGE('',*,*,#14781,.F.);
#20346=ORIENTED_EDGE('',*,*,#14782,.F.);
#20347=ORIENTED_EDGE('',*,*,#14783,.T.);
#20348=ORIENTED_EDGE('',*,*,#14784,.T.);
#20349=ORIENTED_EDGE('',*,*,#14785,.T.);
#20350=ORIENTED_EDGE('',*,*,#14782,.T.);
#20351=ORIENTED_EDGE('',*,*,#14786,.T.);
#20352=ORIENTED_EDGE('',*,*,#14787,.T.);
#20353=ORIENTED_EDGE('',*,*,#14788,.T.);
#20354=ORIENTED_EDGE('',*,*,#14708,.F.);
#20355=ORIENTED_EDGE('',*,*,#14712,.F.);
#20356=ORIENTED_EDGE('',*,*,#14748,.T.);
#20357=ORIENTED_EDGE('',*,*,#14715,.F.);
#20358=ORIENTED_EDGE('',*,*,#14764,.T.);
#20359=ORIENTED_EDGE('',*,*,#14669,.F.);
#20360=ORIENTED_EDGE('',*,*,#14762,.T.);
#20361=ORIENTED_EDGE('',*,*,#14745,.F.);
#20362=ORIENTED_EDGE('',*,*,#14760,.T.);
#20363=ORIENTED_EDGE('',*,*,#14719,.F.);
#20364=ORIENTED_EDGE('',*,*,#14752,.T.);
#20365=ORIENTED_EDGE('',*,*,#14723,.F.);
#20366=ORIENTED_EDGE('',*,*,#14754,.T.);
#20367=ORIENTED_EDGE('',*,*,#14673,.F.);
#20368=ORIENTED_EDGE('',*,*,#14756,.T.);
#20369=ORIENTED_EDGE('',*,*,#14741,.F.);
#20370=ORIENTED_EDGE('',*,*,#14758,.T.);
#20371=ORIENTED_EDGE('',*,*,#14727,.F.);
#20372=ORIENTED_EDGE('',*,*,#14730,.F.);
#20373=ORIENTED_EDGE('',*,*,#14681,.F.);
#20374=ORIENTED_EDGE('',*,*,#14778,.T.);
#20375=ORIENTED_EDGE('',*,*,#14733,.F.);
#20376=ORIENTED_EDGE('',*,*,#14776,.T.);
#20377=ORIENTED_EDGE('',*,*,#14685,.F.);
#20378=ORIENTED_EDGE('',*,*,#14774,.T.);
#20379=ORIENTED_EDGE('',*,*,#14689,.F.);
#20380=ORIENTED_EDGE('',*,*,#14772,.T.);
#20381=ORIENTED_EDGE('',*,*,#14677,.F.);
#20382=ORIENTED_EDGE('',*,*,#14770,.T.);
#20383=ORIENTED_EDGE('',*,*,#14737,.F.);
#20384=ORIENTED_EDGE('',*,*,#14768,.T.);
#20385=ORIENTED_EDGE('',*,*,#14693,.F.);
#20386=ORIENTED_EDGE('',*,*,#14766,.T.);
#20387=ORIENTED_EDGE('',*,*,#14697,.F.);
#20388=ORIENTED_EDGE('',*,*,#14750,.T.);
#20389=ORIENTED_EDGE('',*,*,#14701,.F.);
#20390=ORIENTED_EDGE('',*,*,#14705,.F.);
#20391=ORIENTED_EDGE('',*,*,#14650,.F.);
#20392=ORIENTED_EDGE('',*,*,#14789,.T.);
#20393=ORIENTED_EDGE('',*,*,#14790,.F.);
#20394=ORIENTED_EDGE('',*,*,#14779,.F.);
#20395=ORIENTED_EDGE('',*,*,#14785,.F.);
#20396=ORIENTED_EDGE('',*,*,#14791,.T.);
#20397=ORIENTED_EDGE('',*,*,#14792,.F.);
#20398=ORIENTED_EDGE('',*,*,#14789,.F.);
#20399=ORIENTED_EDGE('',*,*,#14784,.F.);
#20400=ORIENTED_EDGE('',*,*,#14704,.T.);
#20401=ORIENTED_EDGE('',*,*,#14793,.F.);
#20402=ORIENTED_EDGE('',*,*,#14791,.F.);
#20403=ORIENTED_EDGE('',*,*,#14783,.F.);
#20404=ORIENTED_EDGE('',*,*,#14794,.T.);
#20405=ORIENTED_EDGE('',*,*,#14795,.F.);
#20406=ORIENTED_EDGE('',*,*,#14709,.F.);
#20407=ORIENTED_EDGE('',*,*,#14788,.F.);
#20408=ORIENTED_EDGE('',*,*,#14796,.T.);
#20409=ORIENTED_EDGE('',*,*,#14797,.F.);
#20410=ORIENTED_EDGE('',*,*,#14794,.F.);
#20411=ORIENTED_EDGE('',*,*,#14787,.F.);
#20412=ORIENTED_EDGE('',*,*,#14781,.T.);
#20413=ORIENTED_EDGE('',*,*,#14798,.F.);
#20414=ORIENTED_EDGE('',*,*,#14796,.F.);
#20415=ORIENTED_EDGE('',*,*,#14786,.F.);
#20416=ORIENTED_EDGE('',*,*,#14799,.T.);
#20417=ORIENTED_EDGE('',*,*,#14645,.T.);
#20418=ORIENTED_EDGE('',*,*,#14800,.F.);
#20419=ORIENTED_EDGE('',*,*,#14801,.F.);
#20420=ORIENTED_EDGE('',*,*,#14637,.T.);
#20421=ORIENTED_EDGE('',*,*,#14799,.F.);
#20422=ORIENTED_EDGE('',*,*,#14802,.F.);
#20423=ORIENTED_EDGE('',*,*,#14803,.T.);
#20424=ORIENTED_EDGE('',*,*,#14804,.T.);
#20425=ORIENTED_EDGE('',*,*,#14638,.T.);
#20426=ORIENTED_EDGE('',*,*,#14803,.F.);
#20427=ORIENTED_EDGE('',*,*,#14805,.F.);
#20428=ORIENTED_EDGE('',*,*,#14806,.T.);
#20429=ORIENTED_EDGE('',*,*,#14639,.T.);
#20430=ORIENTED_EDGE('',*,*,#14804,.F.);
#20431=ORIENTED_EDGE('',*,*,#14807,.F.);
#20432=ORIENTED_EDGE('',*,*,#14808,.T.);
#20433=ORIENTED_EDGE('',*,*,#14643,.T.);
#20434=ORIENTED_EDGE('',*,*,#14806,.F.);
#20435=ORIENTED_EDGE('',*,*,#14809,.F.);
#20436=ORIENTED_EDGE('',*,*,#14800,.T.);
#20437=ORIENTED_EDGE('',*,*,#14644,.T.);
#20438=ORIENTED_EDGE('',*,*,#14808,.F.);
#20439=ORIENTED_EDGE('',*,*,#14810,.F.);
#20440=ORIENTED_EDGE('',*,*,#14801,.T.);
#20441=ORIENTED_EDGE('',*,*,#14810,.T.);
#20442=ORIENTED_EDGE('',*,*,#14809,.T.);
#20443=ORIENTED_EDGE('',*,*,#14807,.T.);
#20444=ORIENTED_EDGE('',*,*,#14805,.T.);
#20445=ORIENTED_EDGE('',*,*,#14802,.T.);
#20446=ORIENTED_EDGE('',*,*,#14710,.T.);
#20447=ORIENTED_EDGE('',*,*,#14706,.T.);
#20448=ORIENTED_EDGE('',*,*,#14795,.T.);
#20449=ORIENTED_EDGE('',*,*,#14797,.T.);
#20450=ORIENTED_EDGE('',*,*,#14798,.T.);
#20451=ORIENTED_EDGE('',*,*,#14780,.T.);
#20452=ORIENTED_EDGE('',*,*,#14790,.T.);
#20453=ORIENTED_EDGE('',*,*,#14792,.T.);
#20454=ORIENTED_EDGE('',*,*,#14793,.T.);
#20455=ORIENTED_EDGE('',*,*,#14703,.T.);
#20456=ORIENTED_EDGE('',*,*,#14699,.T.);
#20457=ORIENTED_EDGE('',*,*,#14749,.T.);
#20458=ORIENTED_EDGE('',*,*,#14695,.T.);
#20459=ORIENTED_EDGE('',*,*,#14765,.T.);
#20460=ORIENTED_EDGE('',*,*,#14691,.T.);
#20461=ORIENTED_EDGE('',*,*,#14767,.T.);
#20462=ORIENTED_EDGE('',*,*,#14735,.T.);
#20463=ORIENTED_EDGE('',*,*,#14769,.T.);
#20464=ORIENTED_EDGE('',*,*,#14675,.T.);
#20465=ORIENTED_EDGE('',*,*,#14771,.T.);
#20466=ORIENTED_EDGE('',*,*,#14687,.T.);
#20467=ORIENTED_EDGE('',*,*,#14773,.T.);
#20468=ORIENTED_EDGE('',*,*,#14683,.T.);
#20469=ORIENTED_EDGE('',*,*,#14775,.T.);
#20470=ORIENTED_EDGE('',*,*,#14731,.T.);
#20471=ORIENTED_EDGE('',*,*,#14777,.T.);
#20472=ORIENTED_EDGE('',*,*,#14679,.T.);
#20473=ORIENTED_EDGE('',*,*,#14729,.T.);
#20474=ORIENTED_EDGE('',*,*,#14725,.T.);
#20475=ORIENTED_EDGE('',*,*,#14757,.T.);
#20476=ORIENTED_EDGE('',*,*,#14739,.T.);
#20477=ORIENTED_EDGE('',*,*,#14755,.T.);
#20478=ORIENTED_EDGE('',*,*,#14671,.T.);
#20479=ORIENTED_EDGE('',*,*,#14753,.T.);
#20480=ORIENTED_EDGE('',*,*,#14721,.T.);
#20481=ORIENTED_EDGE('',*,*,#14751,.T.);
#20482=ORIENTED_EDGE('',*,*,#14717,.T.);
#20483=ORIENTED_EDGE('',*,*,#14759,.T.);
#20484=ORIENTED_EDGE('',*,*,#14743,.T.);
#20485=ORIENTED_EDGE('',*,*,#14761,.T.);
#20486=ORIENTED_EDGE('',*,*,#14667,.T.);
#20487=ORIENTED_EDGE('',*,*,#14763,.T.);
#20488=ORIENTED_EDGE('',*,*,#14713,.T.);
#20489=ORIENTED_EDGE('',*,*,#14747,.T.);
#20490=ORIENTED_EDGE('',*,*,#14811,.F.);
#20491=ORIENTED_EDGE('',*,*,#14812,.F.);
#20492=ORIENTED_EDGE('',*,*,#14813,.F.);
#20493=ORIENTED_EDGE('',*,*,#14814,.F.);
#20494=ORIENTED_EDGE('',*,*,#14815,.F.);
#20495=ORIENTED_EDGE('',*,*,#14816,.F.);
#20496=ORIENTED_EDGE('',*,*,#14817,.F.);
#20497=ORIENTED_EDGE('',*,*,#14818,.F.);
#20498=ORIENTED_EDGE('',*,*,#14819,.F.);
#20499=ORIENTED_EDGE('',*,*,#14820,.F.);
#20500=ORIENTED_EDGE('',*,*,#14821,.F.);
#20501=ORIENTED_EDGE('',*,*,#14822,.F.);
#20502=ORIENTED_EDGE('',*,*,#14823,.F.);
#20503=ORIENTED_EDGE('',*,*,#14824,.F.);
#20504=ORIENTED_EDGE('',*,*,#14825,.F.);
#20505=ORIENTED_EDGE('',*,*,#14826,.F.);
#20506=ORIENTED_EDGE('',*,*,#14827,.F.);
#20507=ORIENTED_EDGE('',*,*,#14828,.F.);
#20508=ORIENTED_EDGE('',*,*,#14829,.F.);
#20509=ORIENTED_EDGE('',*,*,#14830,.F.);
#20510=ORIENTED_EDGE('',*,*,#14831,.F.);
#20511=ORIENTED_EDGE('',*,*,#14832,.F.);
#20512=ORIENTED_EDGE('',*,*,#14833,.F.);
#20513=ORIENTED_EDGE('',*,*,#14834,.F.);
#20514=ORIENTED_EDGE('',*,*,#14835,.F.);
#20515=ORIENTED_EDGE('',*,*,#14836,.F.);
#20516=ORIENTED_EDGE('',*,*,#14837,.F.);
#20517=ORIENTED_EDGE('',*,*,#14838,.F.);
#20518=ORIENTED_EDGE('',*,*,#14839,.F.);
#20519=ORIENTED_EDGE('',*,*,#14840,.F.);
#20520=ORIENTED_EDGE('',*,*,#14841,.F.);
#20521=ORIENTED_EDGE('',*,*,#14842,.F.);
#20522=ORIENTED_EDGE('',*,*,#14843,.F.);
#20523=ORIENTED_EDGE('',*,*,#14844,.F.);
#20524=ORIENTED_EDGE('',*,*,#14845,.F.);
#20525=ORIENTED_EDGE('',*,*,#14846,.F.);
#20526=ORIENTED_EDGE('',*,*,#14847,.F.);
#20527=ORIENTED_EDGE('',*,*,#14848,.F.);
#20528=ORIENTED_EDGE('',*,*,#14849,.F.);
#20529=ORIENTED_EDGE('',*,*,#14850,.F.);
#20530=ORIENTED_EDGE('',*,*,#14851,.F.);
#20531=ORIENTED_EDGE('',*,*,#14852,.F.);
#20532=ORIENTED_EDGE('',*,*,#14853,.F.);
#20533=ORIENTED_EDGE('',*,*,#14854,.F.);
#20534=ORIENTED_EDGE('',*,*,#14855,.F.);
#20535=ORIENTED_EDGE('',*,*,#14856,.F.);
#20536=ORIENTED_EDGE('',*,*,#14811,.T.);
#20537=ORIENTED_EDGE('',*,*,#14857,.T.);
#20538=ORIENTED_EDGE('',*,*,#14858,.F.);
#20539=ORIENTED_EDGE('',*,*,#14859,.F.);
#20540=ORIENTED_EDGE('',*,*,#14812,.T.);
#20541=ORIENTED_EDGE('',*,*,#14856,.T.);
#20542=ORIENTED_EDGE('',*,*,#14860,.F.);
#20543=ORIENTED_EDGE('',*,*,#14861,.F.);
#20544=ORIENTED_EDGE('',*,*,#14813,.T.);
#20545=ORIENTED_EDGE('',*,*,#14859,.T.);
#20546=ORIENTED_EDGE('',*,*,#14862,.F.);
#20547=ORIENTED_EDGE('',*,*,#14863,.F.);
#20548=ORIENTED_EDGE('',*,*,#14814,.T.);
#20549=ORIENTED_EDGE('',*,*,#14861,.T.);
#20550=ORIENTED_EDGE('',*,*,#14864,.F.);
#20551=ORIENTED_EDGE('',*,*,#14865,.F.);
#20552=ORIENTED_EDGE('',*,*,#14815,.T.);
#20553=ORIENTED_EDGE('',*,*,#14863,.T.);
#20554=ORIENTED_EDGE('',*,*,#14866,.F.);
#20555=ORIENTED_EDGE('',*,*,#14867,.F.);
#20556=ORIENTED_EDGE('',*,*,#14816,.T.);
#20557=ORIENTED_EDGE('',*,*,#14865,.T.);
#20558=ORIENTED_EDGE('',*,*,#14868,.F.);
#20559=ORIENTED_EDGE('',*,*,#14869,.F.);
#20560=ORIENTED_EDGE('',*,*,#14817,.T.);
#20561=ORIENTED_EDGE('',*,*,#14867,.T.);
#20562=ORIENTED_EDGE('',*,*,#14870,.F.);
#20563=ORIENTED_EDGE('',*,*,#14871,.F.);
#20564=ORIENTED_EDGE('',*,*,#14818,.T.);
#20565=ORIENTED_EDGE('',*,*,#14869,.T.);
#20566=ORIENTED_EDGE('',*,*,#14872,.F.);
#20567=ORIENTED_EDGE('',*,*,#14873,.F.);
#20568=ORIENTED_EDGE('',*,*,#14819,.T.);
#20569=ORIENTED_EDGE('',*,*,#14871,.T.);
#20570=ORIENTED_EDGE('',*,*,#14874,.F.);
#20571=ORIENTED_EDGE('',*,*,#14875,.F.);
#20572=ORIENTED_EDGE('',*,*,#14820,.T.);
#20573=ORIENTED_EDGE('',*,*,#14873,.T.);
#20574=ORIENTED_EDGE('',*,*,#14876,.F.);
#20575=ORIENTED_EDGE('',*,*,#14877,.F.);
#20576=ORIENTED_EDGE('',*,*,#14821,.T.);
#20577=ORIENTED_EDGE('',*,*,#14875,.T.);
#20578=ORIENTED_EDGE('',*,*,#14878,.F.);
#20579=ORIENTED_EDGE('',*,*,#14879,.F.);
#20580=ORIENTED_EDGE('',*,*,#14822,.T.);
#20581=ORIENTED_EDGE('',*,*,#14877,.T.);
#20582=ORIENTED_EDGE('',*,*,#14880,.F.);
#20583=ORIENTED_EDGE('',*,*,#14881,.F.);
#20584=ORIENTED_EDGE('',*,*,#14823,.T.);
#20585=ORIENTED_EDGE('',*,*,#14879,.T.);
#20586=ORIENTED_EDGE('',*,*,#14882,.F.);
#20587=ORIENTED_EDGE('',*,*,#14883,.F.);
#20588=ORIENTED_EDGE('',*,*,#14824,.T.);
#20589=ORIENTED_EDGE('',*,*,#14881,.T.);
#20590=ORIENTED_EDGE('',*,*,#14884,.F.);
#20591=ORIENTED_EDGE('',*,*,#14885,.F.);
#20592=ORIENTED_EDGE('',*,*,#14825,.T.);
#20593=ORIENTED_EDGE('',*,*,#14883,.T.);
#20594=ORIENTED_EDGE('',*,*,#14886,.F.);
#20595=ORIENTED_EDGE('',*,*,#14887,.F.);
#20596=ORIENTED_EDGE('',*,*,#14826,.T.);
#20597=ORIENTED_EDGE('',*,*,#14885,.T.);
#20598=ORIENTED_EDGE('',*,*,#14888,.F.);
#20599=ORIENTED_EDGE('',*,*,#14889,.F.);
#20600=ORIENTED_EDGE('',*,*,#14827,.T.);
#20601=ORIENTED_EDGE('',*,*,#14887,.T.);
#20602=ORIENTED_EDGE('',*,*,#14890,.F.);
#20603=ORIENTED_EDGE('',*,*,#14891,.F.);
#20604=ORIENTED_EDGE('',*,*,#14828,.T.);
#20605=ORIENTED_EDGE('',*,*,#14889,.T.);
#20606=ORIENTED_EDGE('',*,*,#14892,.F.);
#20607=ORIENTED_EDGE('',*,*,#14893,.F.);
#20608=ORIENTED_EDGE('',*,*,#14829,.T.);
#20609=ORIENTED_EDGE('',*,*,#14891,.T.);
#20610=ORIENTED_EDGE('',*,*,#14894,.F.);
#20611=ORIENTED_EDGE('',*,*,#14895,.F.);
#20612=ORIENTED_EDGE('',*,*,#14830,.T.);
#20613=ORIENTED_EDGE('',*,*,#14893,.T.);
#20614=ORIENTED_EDGE('',*,*,#14896,.F.);
#20615=ORIENTED_EDGE('',*,*,#14897,.F.);
#20616=ORIENTED_EDGE('',*,*,#14831,.T.);
#20617=ORIENTED_EDGE('',*,*,#14895,.T.);
#20618=ORIENTED_EDGE('',*,*,#14898,.F.);
#20619=ORIENTED_EDGE('',*,*,#14899,.F.);
#20620=ORIENTED_EDGE('',*,*,#14832,.T.);
#20621=ORIENTED_EDGE('',*,*,#14897,.T.);
#20622=ORIENTED_EDGE('',*,*,#14900,.F.);
#20623=ORIENTED_EDGE('',*,*,#14901,.F.);
#20624=ORIENTED_EDGE('',*,*,#14833,.T.);
#20625=ORIENTED_EDGE('',*,*,#14899,.T.);
#20626=ORIENTED_EDGE('',*,*,#14902,.F.);
#20627=ORIENTED_EDGE('',*,*,#14903,.F.);
#20628=ORIENTED_EDGE('',*,*,#14834,.T.);
#20629=ORIENTED_EDGE('',*,*,#14901,.T.);
#20630=ORIENTED_EDGE('',*,*,#14904,.F.);
#20631=ORIENTED_EDGE('',*,*,#14905,.F.);
#20632=ORIENTED_EDGE('',*,*,#14835,.T.);
#20633=ORIENTED_EDGE('',*,*,#14903,.T.);
#20634=ORIENTED_EDGE('',*,*,#14906,.F.);
#20635=ORIENTED_EDGE('',*,*,#14907,.F.);
#20636=ORIENTED_EDGE('',*,*,#14836,.T.);
#20637=ORIENTED_EDGE('',*,*,#14905,.T.);
#20638=ORIENTED_EDGE('',*,*,#14908,.F.);
#20639=ORIENTED_EDGE('',*,*,#14909,.F.);
#20640=ORIENTED_EDGE('',*,*,#14837,.T.);
#20641=ORIENTED_EDGE('',*,*,#14907,.T.);
#20642=ORIENTED_EDGE('',*,*,#14910,.F.);
#20643=ORIENTED_EDGE('',*,*,#14911,.F.);
#20644=ORIENTED_EDGE('',*,*,#14838,.T.);
#20645=ORIENTED_EDGE('',*,*,#14909,.T.);
#20646=ORIENTED_EDGE('',*,*,#14912,.F.);
#20647=ORIENTED_EDGE('',*,*,#14913,.F.);
#20648=ORIENTED_EDGE('',*,*,#14839,.T.);
#20649=ORIENTED_EDGE('',*,*,#14911,.T.);
#20650=ORIENTED_EDGE('',*,*,#14914,.F.);
#20651=ORIENTED_EDGE('',*,*,#14915,.F.);
#20652=ORIENTED_EDGE('',*,*,#14840,.T.);
#20653=ORIENTED_EDGE('',*,*,#14913,.T.);
#20654=ORIENTED_EDGE('',*,*,#14916,.F.);
#20655=ORIENTED_EDGE('',*,*,#14917,.F.);
#20656=ORIENTED_EDGE('',*,*,#14841,.T.);
#20657=ORIENTED_EDGE('',*,*,#14915,.T.);
#20658=ORIENTED_EDGE('',*,*,#14918,.F.);
#20659=ORIENTED_EDGE('',*,*,#14919,.F.);
#20660=ORIENTED_EDGE('',*,*,#14842,.T.);
#20661=ORIENTED_EDGE('',*,*,#14917,.T.);
#20662=ORIENTED_EDGE('',*,*,#14920,.F.);
#20663=ORIENTED_EDGE('',*,*,#14921,.F.);
#20664=ORIENTED_EDGE('',*,*,#14843,.T.);
#20665=ORIENTED_EDGE('',*,*,#14919,.T.);
#20666=ORIENTED_EDGE('',*,*,#14922,.F.);
#20667=ORIENTED_EDGE('',*,*,#14923,.F.);
#20668=ORIENTED_EDGE('',*,*,#14844,.T.);
#20669=ORIENTED_EDGE('',*,*,#14921,.T.);
#20670=ORIENTED_EDGE('',*,*,#14924,.F.);
#20671=ORIENTED_EDGE('',*,*,#14925,.F.);
#20672=ORIENTED_EDGE('',*,*,#14845,.T.);
#20673=ORIENTED_EDGE('',*,*,#14923,.T.);
#20674=ORIENTED_EDGE('',*,*,#14926,.F.);
#20675=ORIENTED_EDGE('',*,*,#14927,.F.);
#20676=ORIENTED_EDGE('',*,*,#14846,.T.);
#20677=ORIENTED_EDGE('',*,*,#14925,.T.);
#20678=ORIENTED_EDGE('',*,*,#14928,.F.);
#20679=ORIENTED_EDGE('',*,*,#14929,.F.);
#20680=ORIENTED_EDGE('',*,*,#14847,.T.);
#20681=ORIENTED_EDGE('',*,*,#14927,.T.);
#20682=ORIENTED_EDGE('',*,*,#14930,.F.);
#20683=ORIENTED_EDGE('',*,*,#14931,.F.);
#20684=ORIENTED_EDGE('',*,*,#14848,.T.);
#20685=ORIENTED_EDGE('',*,*,#14929,.T.);
#20686=ORIENTED_EDGE('',*,*,#14932,.F.);
#20687=ORIENTED_EDGE('',*,*,#14933,.F.);
#20688=ORIENTED_EDGE('',*,*,#14849,.T.);
#20689=ORIENTED_EDGE('',*,*,#14931,.T.);
#20690=ORIENTED_EDGE('',*,*,#14934,.F.);
#20691=ORIENTED_EDGE('',*,*,#14935,.F.);
#20692=ORIENTED_EDGE('',*,*,#14850,.T.);
#20693=ORIENTED_EDGE('',*,*,#14933,.T.);
#20694=ORIENTED_EDGE('',*,*,#14936,.F.);
#20695=ORIENTED_EDGE('',*,*,#14937,.F.);
#20696=ORIENTED_EDGE('',*,*,#14851,.T.);
#20697=ORIENTED_EDGE('',*,*,#14935,.T.);
#20698=ORIENTED_EDGE('',*,*,#14938,.F.);
#20699=ORIENTED_EDGE('',*,*,#14939,.F.);
#20700=ORIENTED_EDGE('',*,*,#14852,.T.);
#20701=ORIENTED_EDGE('',*,*,#14937,.T.);
#20702=ORIENTED_EDGE('',*,*,#14940,.F.);
#20703=ORIENTED_EDGE('',*,*,#14941,.F.);
#20704=ORIENTED_EDGE('',*,*,#14853,.T.);
#20705=ORIENTED_EDGE('',*,*,#14939,.T.);
#20706=ORIENTED_EDGE('',*,*,#14942,.F.);
#20707=ORIENTED_EDGE('',*,*,#14857,.F.);
#20708=ORIENTED_EDGE('',*,*,#14854,.T.);
#20709=ORIENTED_EDGE('',*,*,#14941,.T.);
#20710=ORIENTED_EDGE('',*,*,#14631,.T.);
#20711=ORIENTED_EDGE('',*,*,#14636,.F.);
#20712=ORIENTED_EDGE('',*,*,#14943,.T.);
#20713=ORIENTED_EDGE('',*,*,#14944,.T.);
#20714=ORIENTED_EDGE('',*,*,#14945,.T.);
#20715=ORIENTED_EDGE('',*,*,#14946,.F.);
#20716=ORIENTED_EDGE('',*,*,#14947,.F.);
#20717=ORIENTED_EDGE('',*,*,#14948,.F.);
#20718=ORIENTED_EDGE('',*,*,#14949,.F.);
#20719=ORIENTED_EDGE('',*,*,#14950,.F.);
#20720=ORIENTED_EDGE('',*,*,#14951,.F.);
#20721=ORIENTED_EDGE('',*,*,#14952,.F.);
#20722=ORIENTED_EDGE('',*,*,#14953,.F.);
#20723=ORIENTED_EDGE('',*,*,#14954,.T.);
#20724=ORIENTED_EDGE('',*,*,#14955,.T.);
#20725=ORIENTED_EDGE('',*,*,#14956,.T.);
#20726=ORIENTED_EDGE('',*,*,#14957,.T.);
#20727=ORIENTED_EDGE('',*,*,#14958,.T.);
#20728=ORIENTED_EDGE('',*,*,#14959,.T.);
#20729=ORIENTED_EDGE('',*,*,#14960,.T.);
#20730=ORIENTED_EDGE('',*,*,#14961,.T.);
#20731=ORIENTED_EDGE('',*,*,#14962,.T.);
#20732=ORIENTED_EDGE('',*,*,#14963,.T.);
#20733=ORIENTED_EDGE('',*,*,#14964,.T.);
#20734=ORIENTED_EDGE('',*,*,#14965,.T.);
#20735=ORIENTED_EDGE('',*,*,#14966,.T.);
#20736=ORIENTED_EDGE('',*,*,#14967,.T.);
#20737=ORIENTED_EDGE('',*,*,#14968,.T.);
#20738=ORIENTED_EDGE('',*,*,#14969,.T.);
#20739=ORIENTED_EDGE('',*,*,#14970,.T.);
#20740=ORIENTED_EDGE('',*,*,#14971,.T.);
#20741=ORIENTED_EDGE('',*,*,#14972,.T.);
#20742=ORIENTED_EDGE('',*,*,#14973,.T.);
#20743=ORIENTED_EDGE('',*,*,#14974,.T.);
#20744=ORIENTED_EDGE('',*,*,#14975,.T.);
#20745=ORIENTED_EDGE('',*,*,#14976,.T.);
#20746=ORIENTED_EDGE('',*,*,#14977,.T.);
#20747=ORIENTED_EDGE('',*,*,#14978,.T.);
#20748=ORIENTED_EDGE('',*,*,#14979,.T.);
#20749=ORIENTED_EDGE('',*,*,#14980,.T.);
#20750=ORIENTED_EDGE('',*,*,#14981,.T.);
#20751=ORIENTED_EDGE('',*,*,#14982,.T.);
#20752=ORIENTED_EDGE('',*,*,#14983,.T.);
#20753=ORIENTED_EDGE('',*,*,#14984,.T.);
#20754=ORIENTED_EDGE('',*,*,#14985,.T.);
#20755=ORIENTED_EDGE('',*,*,#14986,.T.);
#20756=ORIENTED_EDGE('',*,*,#14987,.T.);
#20757=ORIENTED_EDGE('',*,*,#14988,.T.);
#20758=ORIENTED_EDGE('',*,*,#14989,.T.);
#20759=ORIENTED_EDGE('',*,*,#14990,.T.);
#20760=ORIENTED_EDGE('',*,*,#14991,.F.);
#20761=ORIENTED_EDGE('',*,*,#14992,.F.);
#20762=ORIENTED_EDGE('',*,*,#14993,.F.);
#20763=ORIENTED_EDGE('',*,*,#14994,.T.);
#20764=ORIENTED_EDGE('',*,*,#14633,.F.);
#20765=ORIENTED_EDGE('',*,*,#14945,.F.);
#20766=ORIENTED_EDGE('',*,*,#14995,.T.);
#20767=ORIENTED_EDGE('',*,*,#14996,.T.);
#20768=ORIENTED_EDGE('',*,*,#14997,.F.);
#20769=ORIENTED_EDGE('',*,*,#14943,.F.);
#20770=ORIENTED_EDGE('',*,*,#14635,.T.);
#20771=ORIENTED_EDGE('',*,*,#14998,.T.);
#20772=ORIENTED_EDGE('',*,*,#14995,.F.);
#20773=ORIENTED_EDGE('',*,*,#14944,.F.);
#20774=ORIENTED_EDGE('',*,*,#14997,.T.);
#20775=ORIENTED_EDGE('',*,*,#14623,.T.);
#20776=ORIENTED_EDGE('',*,*,#14625,.F.);
#20777=ORIENTED_EDGE('',*,*,#14999,.T.);
#20778=ORIENTED_EDGE('',*,*,#15000,.T.);
#20779=ORIENTED_EDGE('',*,*,#15001,.T.);
#20780=ORIENTED_EDGE('',*,*,#15002,.T.);
#20781=ORIENTED_EDGE('',*,*,#15003,.T.);
#20782=ORIENTED_EDGE('',*,*,#14990,.F.);
#20783=ORIENTED_EDGE('',*,*,#15004,.F.);
#20784=ORIENTED_EDGE('',*,*,#15003,.F.);
#20785=ORIENTED_EDGE('',*,*,#15005,.T.);
#20786=ORIENTED_EDGE('',*,*,#15006,.T.);
#20787=ORIENTED_EDGE('',*,*,#14991,.T.);
#20788=ORIENTED_EDGE('',*,*,#15006,.F.);
#20789=ORIENTED_EDGE('',*,*,#15007,.T.);
#20790=ORIENTED_EDGE('',*,*,#15008,.T.);
#20791=ORIENTED_EDGE('',*,*,#14992,.T.);
#20792=ORIENTED_EDGE('',*,*,#15008,.F.);
#20793=ORIENTED_EDGE('',*,*,#15009,.T.);
#20794=ORIENTED_EDGE('',*,*,#15010,.T.);
#20795=ORIENTED_EDGE('',*,*,#14993,.T.);
#20796=ORIENTED_EDGE('',*,*,#15011,.F.);
#20797=ORIENTED_EDGE('',*,*,#15012,.T.);
#20798=ORIENTED_EDGE('',*,*,#14946,.T.);
#20799=ORIENTED_EDGE('',*,*,#15010,.F.);
#20800=ORIENTED_EDGE('',*,*,#15013,.T.);
#20801=ORIENTED_EDGE('',*,*,#15014,.T.);
#20802=ORIENTED_EDGE('',*,*,#14950,.T.);
#20803=ORIENTED_EDGE('',*,*,#15015,.F.);
#20804=ORIENTED_EDGE('',*,*,#15014,.F.);
#20805=ORIENTED_EDGE('',*,*,#15016,.T.);
#20806=ORIENTED_EDGE('',*,*,#15017,.T.);
#20807=ORIENTED_EDGE('',*,*,#14951,.T.);
#20808=ORIENTED_EDGE('',*,*,#15017,.F.);
#20809=ORIENTED_EDGE('',*,*,#15018,.T.);
#20810=ORIENTED_EDGE('',*,*,#15019,.T.);
#20811=ORIENTED_EDGE('',*,*,#14952,.T.);
#20812=ORIENTED_EDGE('',*,*,#15019,.F.);
#20813=ORIENTED_EDGE('',*,*,#15020,.T.);
#20814=ORIENTED_EDGE('',*,*,#15021,.T.);
#20815=ORIENTED_EDGE('',*,*,#14953,.T.);
#20816=ORIENTED_EDGE('',*,*,#15022,.T.);
#20817=ORIENTED_EDGE('',*,*,#15023,.T.);
#20818=ORIENTED_EDGE('',*,*,#14954,.F.);
#20819=ORIENTED_EDGE('',*,*,#15021,.F.);
#20820=ORIENTED_EDGE('',*,*,#15024,.T.);
#20821=ORIENTED_EDGE('',*,*,#15025,.T.);
#20822=ORIENTED_EDGE('',*,*,#14955,.F.);
#20823=ORIENTED_EDGE('',*,*,#15023,.F.);
#20824=ORIENTED_EDGE('',*,*,#15026,.T.);
#20825=ORIENTED_EDGE('',*,*,#15027,.F.);
#20826=ORIENTED_EDGE('',*,*,#14956,.F.);
#20827=ORIENTED_EDGE('',*,*,#15025,.F.);
#20828=ORIENTED_EDGE('',*,*,#15028,.T.);
#20829=ORIENTED_EDGE('',*,*,#15029,.T.);
#20830=ORIENTED_EDGE('',*,*,#14957,.F.);
#20831=ORIENTED_EDGE('',*,*,#15027,.T.);
#20832=ORIENTED_EDGE('',*,*,#15030,.T.);
#20833=ORIENTED_EDGE('',*,*,#15031,.F.);
#20834=ORIENTED_EDGE('',*,*,#14958,.F.);
#20835=ORIENTED_EDGE('',*,*,#15029,.F.);
#20836=ORIENTED_EDGE('',*,*,#15032,.T.);
#20837=ORIENTED_EDGE('',*,*,#15033,.T.);
#20838=ORIENTED_EDGE('',*,*,#14959,.F.);
#20839=ORIENTED_EDGE('',*,*,#15031,.T.);
#20840=ORIENTED_EDGE('',*,*,#15033,.F.);
#20841=ORIENTED_EDGE('',*,*,#15034,.T.);
#20842=ORIENTED_EDGE('',*,*,#15035,.F.);
#20843=ORIENTED_EDGE('',*,*,#14960,.F.);
#20844=ORIENTED_EDGE('',*,*,#15036,.T.);
#20845=ORIENTED_EDGE('',*,*,#15037,.T.);
#20846=ORIENTED_EDGE('',*,*,#14961,.F.);
#20847=ORIENTED_EDGE('',*,*,#15035,.T.);
#20848=ORIENTED_EDGE('',*,*,#15037,.F.);
#20849=ORIENTED_EDGE('',*,*,#15038,.T.);
#20850=ORIENTED_EDGE('',*,*,#15039,.F.);
#20851=ORIENTED_EDGE('',*,*,#14962,.F.);
#20852=ORIENTED_EDGE('',*,*,#15040,.T.);
#20853=ORIENTED_EDGE('',*,*,#15041,.T.);
#20854=ORIENTED_EDGE('',*,*,#14963,.F.);
#20855=ORIENTED_EDGE('',*,*,#15039,.T.);
#20856=ORIENTED_EDGE('',*,*,#15041,.F.);
#20857=ORIENTED_EDGE('',*,*,#15042,.T.);
#20858=ORIENTED_EDGE('',*,*,#15043,.F.);
#20859=ORIENTED_EDGE('',*,*,#14964,.F.);
#20860=ORIENTED_EDGE('',*,*,#15044,.T.);
#20861=ORIENTED_EDGE('',*,*,#15045,.T.);
#20862=ORIENTED_EDGE('',*,*,#14965,.F.);
#20863=ORIENTED_EDGE('',*,*,#15043,.T.);
#20864=ORIENTED_EDGE('',*,*,#15045,.F.);
#20865=ORIENTED_EDGE('',*,*,#15046,.T.);
#20866=ORIENTED_EDGE('',*,*,#15047,.F.);
#20867=ORIENTED_EDGE('',*,*,#14966,.F.);
#20868=ORIENTED_EDGE('',*,*,#15048,.T.);
#20869=ORIENTED_EDGE('',*,*,#15049,.T.);
#20870=ORIENTED_EDGE('',*,*,#14967,.F.);
#20871=ORIENTED_EDGE('',*,*,#15047,.T.);
#20872=ORIENTED_EDGE('',*,*,#15049,.F.);
#20873=ORIENTED_EDGE('',*,*,#15050,.T.);
#20874=ORIENTED_EDGE('',*,*,#15051,.F.);
#20875=ORIENTED_EDGE('',*,*,#14968,.F.);
#20876=ORIENTED_EDGE('',*,*,#15052,.T.);
#20877=ORIENTED_EDGE('',*,*,#15053,.T.);
#20878=ORIENTED_EDGE('',*,*,#14969,.F.);
#20879=ORIENTED_EDGE('',*,*,#15051,.T.);
#20880=ORIENTED_EDGE('',*,*,#15053,.F.);
#20881=ORIENTED_EDGE('',*,*,#15054,.T.);
#20882=ORIENTED_EDGE('',*,*,#15055,.F.);
#20883=ORIENTED_EDGE('',*,*,#14970,.F.);
#20884=ORIENTED_EDGE('',*,*,#15056,.T.);
#20885=ORIENTED_EDGE('',*,*,#15057,.T.);
#20886=ORIENTED_EDGE('',*,*,#14971,.F.);
#20887=ORIENTED_EDGE('',*,*,#15055,.T.);
#20888=ORIENTED_EDGE('',*,*,#15058,.T.);
#20889=ORIENTED_EDGE('',*,*,#15059,.T.);
#20890=ORIENTED_EDGE('',*,*,#14972,.F.);
#20891=ORIENTED_EDGE('',*,*,#15057,.F.);
#20892=ORIENTED_EDGE('',*,*,#15060,.T.);
#20893=ORIENTED_EDGE('',*,*,#15061,.T.);
#20894=ORIENTED_EDGE('',*,*,#14973,.F.);
#20895=ORIENTED_EDGE('',*,*,#15059,.F.);
#20896=ORIENTED_EDGE('',*,*,#15061,.F.);
#20897=ORIENTED_EDGE('',*,*,#15062,.T.);
#20898=ORIENTED_EDGE('',*,*,#15063,.F.);
#20899=ORIENTED_EDGE('',*,*,#14974,.F.);
#20900=ORIENTED_EDGE('',*,*,#15064,.T.);
#20901=ORIENTED_EDGE('',*,*,#15065,.T.);
#20902=ORIENTED_EDGE('',*,*,#14975,.F.);
#20903=ORIENTED_EDGE('',*,*,#15063,.T.);
#20904=ORIENTED_EDGE('',*,*,#15065,.F.);
#20905=ORIENTED_EDGE('',*,*,#15066,.T.);
#20906=ORIENTED_EDGE('',*,*,#15067,.F.);
#20907=ORIENTED_EDGE('',*,*,#14976,.F.);
#20908=ORIENTED_EDGE('',*,*,#15068,.T.);
#20909=ORIENTED_EDGE('',*,*,#15069,.T.);
#20910=ORIENTED_EDGE('',*,*,#14977,.F.);
#20911=ORIENTED_EDGE('',*,*,#15067,.T.);
#20912=ORIENTED_EDGE('',*,*,#15069,.F.);
#20913=ORIENTED_EDGE('',*,*,#15070,.T.);
#20914=ORIENTED_EDGE('',*,*,#15071,.F.);
#20915=ORIENTED_EDGE('',*,*,#14978,.F.);
#20916=ORIENTED_EDGE('',*,*,#15072,.T.);
#20917=ORIENTED_EDGE('',*,*,#15073,.T.);
#20918=ORIENTED_EDGE('',*,*,#14979,.F.);
#20919=ORIENTED_EDGE('',*,*,#15071,.T.);
#20920=ORIENTED_EDGE('',*,*,#15073,.F.);
#20921=ORIENTED_EDGE('',*,*,#15074,.T.);
#20922=ORIENTED_EDGE('',*,*,#15075,.F.);
#20923=ORIENTED_EDGE('',*,*,#14980,.F.);
#20924=ORIENTED_EDGE('',*,*,#15076,.T.);
#20925=ORIENTED_EDGE('',*,*,#15077,.T.);
#20926=ORIENTED_EDGE('',*,*,#14981,.F.);
#20927=ORIENTED_EDGE('',*,*,#15075,.T.);
#20928=ORIENTED_EDGE('',*,*,#15077,.F.);
#20929=ORIENTED_EDGE('',*,*,#15078,.T.);
#20930=ORIENTED_EDGE('',*,*,#15079,.F.);
#20931=ORIENTED_EDGE('',*,*,#14982,.F.);
#20932=ORIENTED_EDGE('',*,*,#15080,.T.);
#20933=ORIENTED_EDGE('',*,*,#15081,.T.);
#20934=ORIENTED_EDGE('',*,*,#14983,.F.);
#20935=ORIENTED_EDGE('',*,*,#15079,.T.);
#20936=ORIENTED_EDGE('',*,*,#15081,.F.);
#20937=ORIENTED_EDGE('',*,*,#15082,.T.);
#20938=ORIENTED_EDGE('',*,*,#15083,.F.);
#20939=ORIENTED_EDGE('',*,*,#14984,.F.);
#20940=ORIENTED_EDGE('',*,*,#15084,.T.);
#20941=ORIENTED_EDGE('',*,*,#15085,.T.);
#20942=ORIENTED_EDGE('',*,*,#14985,.F.);
#20943=ORIENTED_EDGE('',*,*,#15083,.T.);
#20944=ORIENTED_EDGE('',*,*,#15086,.T.);
#20945=ORIENTED_EDGE('',*,*,#15087,.F.);
#20946=ORIENTED_EDGE('',*,*,#14986,.F.);
#20947=ORIENTED_EDGE('',*,*,#15085,.F.);
#20948=ORIENTED_EDGE('',*,*,#15088,.T.);
#20949=ORIENTED_EDGE('',*,*,#15089,.T.);
#20950=ORIENTED_EDGE('',*,*,#14987,.F.);
#20951=ORIENTED_EDGE('',*,*,#15087,.T.);
#20952=ORIENTED_EDGE('',*,*,#15090,.T.);
#20953=ORIENTED_EDGE('',*,*,#15091,.F.);
#20954=ORIENTED_EDGE('',*,*,#14988,.F.);
#20955=ORIENTED_EDGE('',*,*,#15089,.F.);
#20956=ORIENTED_EDGE('',*,*,#15092,.T.);
#20957=ORIENTED_EDGE('',*,*,#15004,.T.);
#20958=ORIENTED_EDGE('',*,*,#14989,.F.);
#20959=ORIENTED_EDGE('',*,*,#15091,.T.);
#20960=ORIENTED_EDGE('',*,*,#14620,.T.);
#20961=ORIENTED_EDGE('',*,*,#14998,.F.);
#20962=ORIENTED_EDGE('',*,*,#14996,.F.);
#20963=ORIENTED_EDGE('',*,*,#14634,.F.);
#20964=ORIENTED_EDGE('',*,*,#14994,.F.);
#20965=ORIENTED_EDGE('',*,*,#15093,.T.);
#20966=ORIENTED_EDGE('',*,*,#15094,.T.);
#20967=ORIENTED_EDGE('',*,*,#15095,.T.);
#20968=ORIENTED_EDGE('',*,*,#15096,.T.);
#20969=ORIENTED_EDGE('',*,*,#15097,.T.);
#20970=ORIENTED_EDGE('',*,*,#15098,.T.);
#20971=ORIENTED_EDGE('',*,*,#15099,.T.);
#20972=ORIENTED_EDGE('',*,*,#15100,.F.);
#20973=ORIENTED_EDGE('',*,*,#15101,.T.);
#20974=ORIENTED_EDGE('',*,*,#14626,.F.);
#20975=ORIENTED_EDGE('',*,*,#15001,.F.);
#20976=ORIENTED_EDGE('',*,*,#15102,.T.);
#20977=ORIENTED_EDGE('',*,*,#15103,.T.);
#20978=ORIENTED_EDGE('',*,*,#15104,.F.);
#20979=ORIENTED_EDGE('',*,*,#14999,.F.);
#20980=ORIENTED_EDGE('',*,*,#14628,.T.);
#20981=ORIENTED_EDGE('',*,*,#15105,.T.);
#20982=ORIENTED_EDGE('',*,*,#15102,.F.);
#20983=ORIENTED_EDGE('',*,*,#15000,.F.);
#20984=ORIENTED_EDGE('',*,*,#15104,.T.);
#20985=ORIENTED_EDGE('',*,*,#15106,.F.);
#20986=ORIENTED_EDGE('',*,*,#15093,.F.);
#20987=ORIENTED_EDGE('',*,*,#15107,.F.);
#20988=ORIENTED_EDGE('',*,*,#15108,.F.);
#20989=ORIENTED_EDGE('',*,*,#15106,.T.);
#20990=ORIENTED_EDGE('',*,*,#15109,.F.);
#20991=ORIENTED_EDGE('',*,*,#15110,.T.);
#20992=ORIENTED_EDGE('',*,*,#15111,.T.);
#20993=ORIENTED_EDGE('',*,*,#15112,.F.);
#20994=ORIENTED_EDGE('',*,*,#15094,.F.);
#20995=ORIENTED_EDGE('',*,*,#15113,.T.);
#20996=ORIENTED_EDGE('',*,*,#15114,.T.);
#20997=ORIENTED_EDGE('',*,*,#15115,.F.);
#20998=ORIENTED_EDGE('',*,*,#15110,.F.);
#20999=ORIENTED_EDGE('',*,*,#15116,.T.);
#21000=ORIENTED_EDGE('',*,*,#15117,.T.);
#21001=ORIENTED_EDGE('',*,*,#15118,.T.);
#21002=ORIENTED_EDGE('',*,*,#15119,.F.);
#21003=ORIENTED_EDGE('',*,*,#15119,.T.);
#21004=ORIENTED_EDGE('',*,*,#15120,.F.);
#21005=ORIENTED_EDGE('',*,*,#15121,.T.);
#21006=ORIENTED_EDGE('',*,*,#15098,.F.);
#21007=ORIENTED_EDGE('',*,*,#15122,.F.);
#21008=ORIENTED_EDGE('',*,*,#15123,.T.);
#21009=ORIENTED_EDGE('',*,*,#15121,.F.);
#21010=ORIENTED_EDGE('',*,*,#15124,.F.);
#21011=ORIENTED_EDGE('',*,*,#15125,.T.);
#21012=ORIENTED_EDGE('',*,*,#15099,.F.);
#21013=ORIENTED_EDGE('',*,*,#15092,.F.);
#21014=ORIENTED_EDGE('',*,*,#15090,.F.);
#21015=ORIENTED_EDGE('',*,*,#15088,.F.);
#21016=ORIENTED_EDGE('',*,*,#15086,.F.);
#21017=ORIENTED_EDGE('',*,*,#15084,.F.);
#21018=ORIENTED_EDGE('',*,*,#15082,.F.);
#21019=ORIENTED_EDGE('',*,*,#15080,.F.);
#21020=ORIENTED_EDGE('',*,*,#15078,.F.);
#21021=ORIENTED_EDGE('',*,*,#15076,.F.);
#21022=ORIENTED_EDGE('',*,*,#15074,.F.);
#21023=ORIENTED_EDGE('',*,*,#15072,.F.);
#21024=ORIENTED_EDGE('',*,*,#15070,.F.);
#21025=ORIENTED_EDGE('',*,*,#15068,.F.);
#21026=ORIENTED_EDGE('',*,*,#15066,.F.);
#21027=ORIENTED_EDGE('',*,*,#15064,.F.);
#21028=ORIENTED_EDGE('',*,*,#15062,.F.);
#21029=ORIENTED_EDGE('',*,*,#15060,.F.);
#21030=ORIENTED_EDGE('',*,*,#15058,.F.);
#21031=ORIENTED_EDGE('',*,*,#15056,.F.);
#21032=ORIENTED_EDGE('',*,*,#15054,.F.);
#21033=ORIENTED_EDGE('',*,*,#15052,.F.);
#21034=ORIENTED_EDGE('',*,*,#15050,.F.);
#21035=ORIENTED_EDGE('',*,*,#15048,.F.);
#21036=ORIENTED_EDGE('',*,*,#15046,.F.);
#21037=ORIENTED_EDGE('',*,*,#15044,.F.);
#21038=ORIENTED_EDGE('',*,*,#15042,.F.);
#21039=ORIENTED_EDGE('',*,*,#15040,.F.);
#21040=ORIENTED_EDGE('',*,*,#15038,.F.);
#21041=ORIENTED_EDGE('',*,*,#15036,.F.);
#21042=ORIENTED_EDGE('',*,*,#15034,.F.);
#21043=ORIENTED_EDGE('',*,*,#15032,.F.);
#21044=ORIENTED_EDGE('',*,*,#15030,.F.);
#21045=ORIENTED_EDGE('',*,*,#15028,.F.);
#21046=ORIENTED_EDGE('',*,*,#15026,.F.);
#21047=ORIENTED_EDGE('',*,*,#15024,.F.);
#21048=ORIENTED_EDGE('',*,*,#15022,.F.);
#21049=ORIENTED_EDGE('',*,*,#15020,.F.);
#21050=ORIENTED_EDGE('',*,*,#15018,.F.);
#21051=ORIENTED_EDGE('',*,*,#15016,.F.);
#21052=ORIENTED_EDGE('',*,*,#15013,.F.);
#21053=ORIENTED_EDGE('',*,*,#15009,.F.);
#21054=ORIENTED_EDGE('',*,*,#15007,.F.);
#21055=ORIENTED_EDGE('',*,*,#15005,.F.);
#21056=ORIENTED_EDGE('',*,*,#15002,.F.);
#21057=ORIENTED_EDGE('',*,*,#15126,.T.);
#21058=ORIENTED_EDGE('',*,*,#15127,.T.);
#21059=ORIENTED_EDGE('',*,*,#15128,.T.);
#21060=ORIENTED_EDGE('',*,*,#15129,.T.);
#21061=ORIENTED_EDGE('',*,*,#15130,.T.);
#21062=ORIENTED_EDGE('',*,*,#15131,.T.);
#21063=ORIENTED_EDGE('',*,*,#15132,.T.);
#21064=ORIENTED_EDGE('',*,*,#15133,.T.);
#21065=ORIENTED_EDGE('',*,*,#15134,.T.);
#21066=ORIENTED_EDGE('',*,*,#15135,.T.);
#21067=ORIENTED_EDGE('',*,*,#15136,.T.);
#21068=ORIENTED_EDGE('',*,*,#15137,.T.);
#21069=ORIENTED_EDGE('',*,*,#15138,.T.);
#21070=ORIENTED_EDGE('',*,*,#15139,.T.);
#21071=ORIENTED_EDGE('',*,*,#15140,.T.);
#21072=ORIENTED_EDGE('',*,*,#15141,.T.);
#21073=ORIENTED_EDGE('',*,*,#15142,.T.);
#21074=ORIENTED_EDGE('',*,*,#15143,.T.);
#21075=ORIENTED_EDGE('',*,*,#15144,.T.);
#21076=ORIENTED_EDGE('',*,*,#15145,.T.);
#21077=ORIENTED_EDGE('',*,*,#15146,.T.);
#21078=ORIENTED_EDGE('',*,*,#15147,.T.);
#21079=ORIENTED_EDGE('',*,*,#15148,.T.);
#21080=ORIENTED_EDGE('',*,*,#15149,.T.);
#21081=ORIENTED_EDGE('',*,*,#15150,.T.);
#21082=ORIENTED_EDGE('',*,*,#15151,.T.);
#21083=ORIENTED_EDGE('',*,*,#15152,.T.);
#21084=ORIENTED_EDGE('',*,*,#15153,.T.);
#21085=ORIENTED_EDGE('',*,*,#15154,.T.);
#21086=ORIENTED_EDGE('',*,*,#15155,.T.);
#21087=ORIENTED_EDGE('',*,*,#15156,.T.);
#21088=ORIENTED_EDGE('',*,*,#15157,.T.);
#21089=ORIENTED_EDGE('',*,*,#15158,.T.);
#21090=ORIENTED_EDGE('',*,*,#15159,.T.);
#21091=ORIENTED_EDGE('',*,*,#15160,.T.);
#21092=ORIENTED_EDGE('',*,*,#15161,.T.);
#21093=ORIENTED_EDGE('',*,*,#15162,.T.);
#21094=ORIENTED_EDGE('',*,*,#15163,.T.);
#21095=ORIENTED_EDGE('',*,*,#15164,.T.);
#21096=ORIENTED_EDGE('',*,*,#15165,.T.);
#21097=ORIENTED_EDGE('',*,*,#15166,.T.);
#21098=ORIENTED_EDGE('',*,*,#15167,.T.);
#21099=ORIENTED_EDGE('',*,*,#15168,.T.);
#21100=ORIENTED_EDGE('',*,*,#15169,.T.);
#21101=ORIENTED_EDGE('',*,*,#15170,.F.);
#21102=ORIENTED_EDGE('',*,*,#15122,.T.);
#21103=ORIENTED_EDGE('',*,*,#15097,.F.);
#21104=ORIENTED_EDGE('',*,*,#15171,.F.);
#21105=ORIENTED_EDGE('',*,*,#15095,.F.);
#21106=ORIENTED_EDGE('',*,*,#15112,.T.);
#21107=ORIENTED_EDGE('',*,*,#15172,.F.);
#21108=ORIENTED_EDGE('',*,*,#15173,.T.);
#21109=ORIENTED_EDGE('',*,*,#15174,.T.);
#21110=ORIENTED_EDGE('',*,*,#15175,.F.);
#21111=ORIENTED_EDGE('',*,*,#15107,.T.);
#21112=ORIENTED_EDGE('',*,*,#15096,.F.);
#21113=ORIENTED_EDGE('',*,*,#15173,.F.);
#21114=ORIENTED_EDGE('',*,*,#15176,.T.);
#21115=ORIENTED_EDGE('',*,*,#15177,.T.);
#21116=ORIENTED_EDGE('',*,*,#15178,.T.);
#21117=ORIENTED_EDGE('',*,*,#15179,.T.);
#21118=ORIENTED_EDGE('',*,*,#15174,.F.);
#21119=ORIENTED_EDGE('',*,*,#15180,.T.);
#21120=ORIENTED_EDGE('',*,*,#15171,.T.);
#21121=ORIENTED_EDGE('',*,*,#15100,.T.);
#21122=ORIENTED_EDGE('',*,*,#15125,.F.);
#21123=ORIENTED_EDGE('',*,*,#15181,.T.);
#21124=ORIENTED_EDGE('',*,*,#15182,.T.);
#21125=ORIENTED_EDGE('',*,*,#15183,.T.);
#21126=ORIENTED_EDGE('',*,*,#15184,.T.);
#21127=ORIENTED_EDGE('',*,*,#15185,.F.);
#21128=ORIENTED_EDGE('',*,*,#15182,.F.);
#21129=ORIENTED_EDGE('',*,*,#14597,.T.);
#21130=ORIENTED_EDGE('',*,*,#15105,.F.);
#21131=ORIENTED_EDGE('',*,*,#15103,.F.);
#21132=ORIENTED_EDGE('',*,*,#14627,.F.);
#21133=ORIENTED_EDGE('',*,*,#15101,.F.);
#21134=ORIENTED_EDGE('',*,*,#15186,.F.);
#21135=ORIENTED_EDGE('',*,*,#14662,.T.);
#21136=ORIENTED_EDGE('',*,*,#15187,.F.);
#21137=ORIENTED_EDGE('',*,*,#15113,.F.);
#21138=ORIENTED_EDGE('',*,*,#15109,.T.);
#21139=ORIENTED_EDGE('',*,*,#15108,.T.);
#21140=ORIENTED_EDGE('',*,*,#15175,.T.);
#21141=ORIENTED_EDGE('',*,*,#15179,.F.);
#21142=ORIENTED_EDGE('',*,*,#15188,.T.);
#21143=ORIENTED_EDGE('',*,*,#15116,.F.);
#21144=ORIENTED_EDGE('',*,*,#15123,.F.);
#21145=ORIENTED_EDGE('',*,*,#15189,.F.);
#21146=ORIENTED_EDGE('',*,*,#15190,.T.);
#21147=ORIENTED_EDGE('',*,*,#15191,.F.);
#21148=ORIENTED_EDGE('',*,*,#14605,.T.);
#21149=ORIENTED_EDGE('',*,*,#15192,.T.);
#21150=ORIENTED_EDGE('',*,*,#15193,.T.);
#21151=ORIENTED_EDGE('',*,*,#15191,.T.);
#21152=ORIENTED_EDGE('',*,*,#15194,.T.);
#21153=ORIENTED_EDGE('',*,*,#15195,.F.);
#21154=ORIENTED_EDGE('',*,*,#14666,.T.);
#21155=ORIENTED_EDGE('',*,*,#15196,.F.);
#21156=ORIENTED_EDGE('',*,*,#15197,.F.);
#21157=ORIENTED_EDGE('',*,*,#15198,.F.);
#21158=ORIENTED_EDGE('',*,*,#15199,.T.);
#21159=ORIENTED_EDGE('',*,*,#15197,.T.);
#21160=ORIENTED_EDGE('',*,*,#15200,.T.);
#21161=ORIENTED_EDGE('',*,*,#15201,.T.);
#21162=ORIENTED_EDGE('',*,*,#15202,.F.);
#21163=ORIENTED_EDGE('',*,*,#15111,.F.);
#21164=ORIENTED_EDGE('',*,*,#15115,.T.);
#21165=ORIENTED_EDGE('',*,*,#15203,.T.);
#21166=ORIENTED_EDGE('',*,*,#15198,.T.);
#21167=ORIENTED_EDGE('',*,*,#14611,.T.);
#21168=ORIENTED_EDGE('',*,*,#15204,.F.);
#21169=ORIENTED_EDGE('',*,*,#15192,.F.);
#21170=ORIENTED_EDGE('',*,*,#15205,.F.);
#21171=ORIENTED_EDGE('',*,*,#15206,.F.);
#21172=ORIENTED_EDGE('',*,*,#15207,.F.);
#21173=ORIENTED_EDGE('',*,*,#15183,.F.);
#21174=ORIENTED_EDGE('',*,*,#15181,.F.);
#21175=ORIENTED_EDGE('',*,*,#15124,.T.);
#21176=ORIENTED_EDGE('',*,*,#15120,.T.);
#21177=ORIENTED_EDGE('',*,*,#15118,.F.);
#21178=ORIENTED_EDGE('',*,*,#15208,.F.);
#21179=ORIENTED_EDGE('',*,*,#14656,.F.);
#21180=ORIENTED_EDGE('',*,*,#15209,.T.);
#21181=ORIENTED_EDGE('',*,*,#15210,.F.);
#21182=ORIENTED_EDGE('',*,*,#15126,.F.);
#21183=ORIENTED_EDGE('',*,*,#15211,.T.);
#21184=ORIENTED_EDGE('',*,*,#15212,.T.);
#21185=ORIENTED_EDGE('',*,*,#15213,.F.);
#21186=ORIENTED_EDGE('',*,*,#15127,.F.);
#21187=ORIENTED_EDGE('',*,*,#15210,.T.);
#21188=ORIENTED_EDGE('',*,*,#15214,.T.);
#21189=ORIENTED_EDGE('',*,*,#15215,.F.);
#21190=ORIENTED_EDGE('',*,*,#15128,.F.);
#21191=ORIENTED_EDGE('',*,*,#15213,.T.);
#21192=ORIENTED_EDGE('',*,*,#15216,.T.);
#21193=ORIENTED_EDGE('',*,*,#15217,.F.);
#21194=ORIENTED_EDGE('',*,*,#15129,.F.);
#21195=ORIENTED_EDGE('',*,*,#15215,.T.);
#21196=ORIENTED_EDGE('',*,*,#15218,.T.);
#21197=ORIENTED_EDGE('',*,*,#15219,.F.);
#21198=ORIENTED_EDGE('',*,*,#15130,.F.);
#21199=ORIENTED_EDGE('',*,*,#15217,.T.);
#21200=ORIENTED_EDGE('',*,*,#15220,.T.);
#21201=ORIENTED_EDGE('',*,*,#15221,.F.);
#21202=ORIENTED_EDGE('',*,*,#15131,.F.);
#21203=ORIENTED_EDGE('',*,*,#15219,.T.);
#21204=ORIENTED_EDGE('',*,*,#15222,.T.);
#21205=ORIENTED_EDGE('',*,*,#15223,.F.);
#21206=ORIENTED_EDGE('',*,*,#15132,.F.);
#21207=ORIENTED_EDGE('',*,*,#15221,.T.);
#21208=ORIENTED_EDGE('',*,*,#15224,.T.);
#21209=ORIENTED_EDGE('',*,*,#15225,.F.);
#21210=ORIENTED_EDGE('',*,*,#15133,.F.);
#21211=ORIENTED_EDGE('',*,*,#15223,.T.);
#21212=ORIENTED_EDGE('',*,*,#15226,.T.);
#21213=ORIENTED_EDGE('',*,*,#15227,.F.);
#21214=ORIENTED_EDGE('',*,*,#15134,.F.);
#21215=ORIENTED_EDGE('',*,*,#15225,.T.);
#21216=ORIENTED_EDGE('',*,*,#15228,.T.);
#21217=ORIENTED_EDGE('',*,*,#15229,.F.);
#21218=ORIENTED_EDGE('',*,*,#15135,.F.);
#21219=ORIENTED_EDGE('',*,*,#15227,.T.);
#21220=ORIENTED_EDGE('',*,*,#15230,.T.);
#21221=ORIENTED_EDGE('',*,*,#15231,.F.);
#21222=ORIENTED_EDGE('',*,*,#15136,.F.);
#21223=ORIENTED_EDGE('',*,*,#15229,.T.);
#21224=ORIENTED_EDGE('',*,*,#15232,.T.);
#21225=ORIENTED_EDGE('',*,*,#15233,.F.);
#21226=ORIENTED_EDGE('',*,*,#15137,.F.);
#21227=ORIENTED_EDGE('',*,*,#15231,.T.);
#21228=ORIENTED_EDGE('',*,*,#15234,.T.);
#21229=ORIENTED_EDGE('',*,*,#15235,.F.);
#21230=ORIENTED_EDGE('',*,*,#15138,.F.);
#21231=ORIENTED_EDGE('',*,*,#15233,.T.);
#21232=ORIENTED_EDGE('',*,*,#15236,.T.);
#21233=ORIENTED_EDGE('',*,*,#15237,.F.);
#21234=ORIENTED_EDGE('',*,*,#15139,.F.);
#21235=ORIENTED_EDGE('',*,*,#15235,.T.);
#21236=ORIENTED_EDGE('',*,*,#15238,.T.);
#21237=ORIENTED_EDGE('',*,*,#15239,.F.);
#21238=ORIENTED_EDGE('',*,*,#15140,.F.);
#21239=ORIENTED_EDGE('',*,*,#15237,.T.);
#21240=ORIENTED_EDGE('',*,*,#15240,.T.);
#21241=ORIENTED_EDGE('',*,*,#15241,.F.);
#21242=ORIENTED_EDGE('',*,*,#15141,.F.);
#21243=ORIENTED_EDGE('',*,*,#15239,.T.);
#21244=ORIENTED_EDGE('',*,*,#15242,.T.);
#21245=ORIENTED_EDGE('',*,*,#15243,.F.);
#21246=ORIENTED_EDGE('',*,*,#15142,.F.);
#21247=ORIENTED_EDGE('',*,*,#15241,.T.);
#21248=ORIENTED_EDGE('',*,*,#15244,.T.);
#21249=ORIENTED_EDGE('',*,*,#15245,.F.);
#21250=ORIENTED_EDGE('',*,*,#15143,.F.);
#21251=ORIENTED_EDGE('',*,*,#15243,.T.);
#21252=ORIENTED_EDGE('',*,*,#15246,.T.);
#21253=ORIENTED_EDGE('',*,*,#15247,.F.);
#21254=ORIENTED_EDGE('',*,*,#15144,.F.);
#21255=ORIENTED_EDGE('',*,*,#15245,.T.);
#21256=ORIENTED_EDGE('',*,*,#15248,.T.);
#21257=ORIENTED_EDGE('',*,*,#15249,.F.);
#21258=ORIENTED_EDGE('',*,*,#15145,.F.);
#21259=ORIENTED_EDGE('',*,*,#15247,.T.);
#21260=ORIENTED_EDGE('',*,*,#15250,.T.);
#21261=ORIENTED_EDGE('',*,*,#15251,.F.);
#21262=ORIENTED_EDGE('',*,*,#15146,.F.);
#21263=ORIENTED_EDGE('',*,*,#15249,.T.);
#21264=ORIENTED_EDGE('',*,*,#15252,.T.);
#21265=ORIENTED_EDGE('',*,*,#15253,.F.);
#21266=ORIENTED_EDGE('',*,*,#15147,.F.);
#21267=ORIENTED_EDGE('',*,*,#15251,.T.);
#21268=ORIENTED_EDGE('',*,*,#15254,.T.);
#21269=ORIENTED_EDGE('',*,*,#15255,.F.);
#21270=ORIENTED_EDGE('',*,*,#15148,.F.);
#21271=ORIENTED_EDGE('',*,*,#15253,.T.);
#21272=ORIENTED_EDGE('',*,*,#15256,.T.);
#21273=ORIENTED_EDGE('',*,*,#15257,.F.);
#21274=ORIENTED_EDGE('',*,*,#15149,.F.);
#21275=ORIENTED_EDGE('',*,*,#15255,.T.);
#21276=ORIENTED_EDGE('',*,*,#15258,.T.);
#21277=ORIENTED_EDGE('',*,*,#15259,.F.);
#21278=ORIENTED_EDGE('',*,*,#15150,.F.);
#21279=ORIENTED_EDGE('',*,*,#15257,.T.);
#21280=ORIENTED_EDGE('',*,*,#15260,.T.);
#21281=ORIENTED_EDGE('',*,*,#15261,.F.);
#21282=ORIENTED_EDGE('',*,*,#15151,.F.);
#21283=ORIENTED_EDGE('',*,*,#15259,.T.);
#21284=ORIENTED_EDGE('',*,*,#15262,.T.);
#21285=ORIENTED_EDGE('',*,*,#15263,.F.);
#21286=ORIENTED_EDGE('',*,*,#15152,.F.);
#21287=ORIENTED_EDGE('',*,*,#15261,.T.);
#21288=ORIENTED_EDGE('',*,*,#15264,.T.);
#21289=ORIENTED_EDGE('',*,*,#15265,.F.);
#21290=ORIENTED_EDGE('',*,*,#15153,.F.);
#21291=ORIENTED_EDGE('',*,*,#15263,.T.);
#21292=ORIENTED_EDGE('',*,*,#15266,.T.);
#21293=ORIENTED_EDGE('',*,*,#15267,.F.);
#21294=ORIENTED_EDGE('',*,*,#15154,.F.);
#21295=ORIENTED_EDGE('',*,*,#15265,.T.);
#21296=ORIENTED_EDGE('',*,*,#15268,.T.);
#21297=ORIENTED_EDGE('',*,*,#15269,.F.);
#21298=ORIENTED_EDGE('',*,*,#15155,.F.);
#21299=ORIENTED_EDGE('',*,*,#15267,.T.);
#21300=ORIENTED_EDGE('',*,*,#15270,.T.);
#21301=ORIENTED_EDGE('',*,*,#15271,.F.);
#21302=ORIENTED_EDGE('',*,*,#15156,.F.);
#21303=ORIENTED_EDGE('',*,*,#15269,.T.);
#21304=ORIENTED_EDGE('',*,*,#15272,.T.);
#21305=ORIENTED_EDGE('',*,*,#15273,.F.);
#21306=ORIENTED_EDGE('',*,*,#15157,.F.);
#21307=ORIENTED_EDGE('',*,*,#15271,.T.);
#21308=ORIENTED_EDGE('',*,*,#15274,.T.);
#21309=ORIENTED_EDGE('',*,*,#15275,.F.);
#21310=ORIENTED_EDGE('',*,*,#15158,.F.);
#21311=ORIENTED_EDGE('',*,*,#15273,.T.);
#21312=ORIENTED_EDGE('',*,*,#15276,.T.);
#21313=ORIENTED_EDGE('',*,*,#15277,.F.);
#21314=ORIENTED_EDGE('',*,*,#15159,.F.);
#21315=ORIENTED_EDGE('',*,*,#15275,.T.);
#21316=ORIENTED_EDGE('',*,*,#15278,.T.);
#21317=ORIENTED_EDGE('',*,*,#15279,.F.);
#21318=ORIENTED_EDGE('',*,*,#15160,.F.);
#21319=ORIENTED_EDGE('',*,*,#15277,.T.);
#21320=ORIENTED_EDGE('',*,*,#15280,.T.);
#21321=ORIENTED_EDGE('',*,*,#15281,.F.);
#21322=ORIENTED_EDGE('',*,*,#15161,.F.);
#21323=ORIENTED_EDGE('',*,*,#15279,.T.);
#21324=ORIENTED_EDGE('',*,*,#15282,.T.);
#21325=ORIENTED_EDGE('',*,*,#15283,.F.);
#21326=ORIENTED_EDGE('',*,*,#15162,.F.);
#21327=ORIENTED_EDGE('',*,*,#15281,.T.);
#21328=ORIENTED_EDGE('',*,*,#15284,.T.);
#21329=ORIENTED_EDGE('',*,*,#15285,.F.);
#21330=ORIENTED_EDGE('',*,*,#15163,.F.);
#21331=ORIENTED_EDGE('',*,*,#15283,.T.);
#21332=ORIENTED_EDGE('',*,*,#15286,.T.);
#21333=ORIENTED_EDGE('',*,*,#15287,.F.);
#21334=ORIENTED_EDGE('',*,*,#15164,.F.);
#21335=ORIENTED_EDGE('',*,*,#15285,.T.);
#21336=ORIENTED_EDGE('',*,*,#15288,.T.);
#21337=ORIENTED_EDGE('',*,*,#15289,.F.);
#21338=ORIENTED_EDGE('',*,*,#15165,.F.);
#21339=ORIENTED_EDGE('',*,*,#15287,.T.);
#21340=ORIENTED_EDGE('',*,*,#15290,.T.);
#21341=ORIENTED_EDGE('',*,*,#15291,.F.);
#21342=ORIENTED_EDGE('',*,*,#15166,.F.);
#21343=ORIENTED_EDGE('',*,*,#15289,.T.);
#21344=ORIENTED_EDGE('',*,*,#15292,.T.);
#21345=ORIENTED_EDGE('',*,*,#15293,.F.);
#21346=ORIENTED_EDGE('',*,*,#15167,.F.);
#21347=ORIENTED_EDGE('',*,*,#15291,.T.);
#21348=ORIENTED_EDGE('',*,*,#15294,.T.);
#21349=ORIENTED_EDGE('',*,*,#15295,.F.);
#21350=ORIENTED_EDGE('',*,*,#15168,.F.);
#21351=ORIENTED_EDGE('',*,*,#15293,.T.);
#21352=ORIENTED_EDGE('',*,*,#15296,.T.);
#21353=ORIENTED_EDGE('',*,*,#15211,.F.);
#21354=ORIENTED_EDGE('',*,*,#15169,.F.);
#21355=ORIENTED_EDGE('',*,*,#15295,.T.);
#21356=ORIENTED_EDGE('',*,*,#15297,.T.);
#21357=ORIENTED_EDGE('',*,*,#15298,.T.);
#21358=ORIENTED_EDGE('',*,*,#15299,.T.);
#21359=ORIENTED_EDGE('',*,*,#15300,.T.);
#21360=ORIENTED_EDGE('',*,*,#14622,.F.);
#21361=ORIENTED_EDGE('',*,*,#15301,.F.);
#21362=ORIENTED_EDGE('',*,*,#15302,.T.);
#21363=ORIENTED_EDGE('',*,*,#15303,.F.);
#21364=ORIENTED_EDGE('',*,*,#15298,.F.);
#21365=ORIENTED_EDGE('',*,*,#15304,.F.);
#21366=ORIENTED_EDGE('',*,*,#15305,.F.);
#21367=ORIENTED_EDGE('',*,*,#15306,.F.);
#21368=ORIENTED_EDGE('',*,*,#15302,.F.);
#21369=ORIENTED_EDGE('',*,*,#15307,.F.);
#21370=ORIENTED_EDGE('',*,*,#15308,.F.);
#21371=ORIENTED_EDGE('',*,*,#15309,.F.);
#21372=ORIENTED_EDGE('',*,*,#15305,.T.);
#21373=ORIENTED_EDGE('',*,*,#15310,.F.);
#21374=ORIENTED_EDGE('',*,*,#15311,.F.);
#21375=ORIENTED_EDGE('',*,*,#15312,.F.);
#21376=ORIENTED_EDGE('',*,*,#15308,.T.);
#21377=ORIENTED_EDGE('',*,*,#14619,.F.);
#21378=ORIENTED_EDGE('',*,*,#15313,.F.);
#21379=ORIENTED_EDGE('',*,*,#15314,.F.);
#21380=ORIENTED_EDGE('',*,*,#15315,.F.);
#21381=ORIENTED_EDGE('',*,*,#15316,.T.);
#21382=ORIENTED_EDGE('',*,*,#14616,.F.);
#21383=ORIENTED_EDGE('',*,*,#15317,.F.);
#21384=ORIENTED_EDGE('',*,*,#15318,.F.);
#21385=ORIENTED_EDGE('',*,*,#15319,.F.);
#21386=ORIENTED_EDGE('',*,*,#15314,.T.);
#21387=ORIENTED_EDGE('',*,*,#15320,.F.);
#21388=ORIENTED_EDGE('',*,*,#15321,.F.);
#21389=ORIENTED_EDGE('',*,*,#15322,.F.);
#21390=ORIENTED_EDGE('',*,*,#15318,.T.);
#21391=ORIENTED_EDGE('',*,*,#15323,.F.);
#21392=ORIENTED_EDGE('',*,*,#15321,.T.);
#21393=ORIENTED_EDGE('',*,*,#15324,.F.);
#21394=ORIENTED_EDGE('',*,*,#15300,.F.);
#21395=ORIENTED_EDGE('',*,*,#15325,.F.);
#21396=ORIENTED_EDGE('',*,*,#15189,.T.);
#21397=ORIENTED_EDGE('',*,*,#15170,.T.);
#21398=ORIENTED_EDGE('',*,*,#15326,.T.);
#21399=ORIENTED_EDGE('',*,*,#15327,.T.);
#21400=ORIENTED_EDGE('',*,*,#15328,.T.);
#21401=ORIENTED_EDGE('',*,*,#15328,.F.);
#21402=ORIENTED_EDGE('',*,*,#15329,.T.);
#21403=ORIENTED_EDGE('',*,*,#15330,.T.);
#21404=ORIENTED_EDGE('',*,*,#15331,.F.);
#21405=ORIENTED_EDGE('',*,*,#15332,.T.);
#21406=ORIENTED_EDGE('',*,*,#15333,.F.);
#21407=ORIENTED_EDGE('',*,*,#15330,.F.);
#21408=ORIENTED_EDGE('',*,*,#15334,.T.);
#21409=ORIENTED_EDGE('',*,*,#14604,.F.);
#21410=ORIENTED_EDGE('',*,*,#14607,.F.);
#21411=ORIENTED_EDGE('',*,*,#15335,.T.);
#21412=ORIENTED_EDGE('',*,*,#15336,.T.);
#21413=ORIENTED_EDGE('',*,*,#15332,.F.);
#21414=ORIENTED_EDGE('',*,*,#15337,.F.);
#21415=ORIENTED_EDGE('',*,*,#15338,.T.);
#21416=ORIENTED_EDGE('',*,*,#15339,.T.);
#21417=ORIENTED_EDGE('',*,*,#15335,.F.);
#21418=ORIENTED_EDGE('',*,*,#15340,.F.);
#21419=ORIENTED_EDGE('',*,*,#15341,.T.);
#21420=ORIENTED_EDGE('',*,*,#15342,.T.);
#21421=ORIENTED_EDGE('',*,*,#15338,.F.);
#21422=ORIENTED_EDGE('',*,*,#15343,.F.);
#21423=ORIENTED_EDGE('',*,*,#15341,.F.);
#21424=ORIENTED_EDGE('',*,*,#15344,.T.);
#21425=ORIENTED_EDGE('',*,*,#15345,.T.);
#21426=ORIENTED_EDGE('',*,*,#15346,.F.);
#21427=ORIENTED_EDGE('',*,*,#15347,.T.);
#21428=ORIENTED_EDGE('',*,*,#15348,.T.);
#21429=ORIENTED_EDGE('',*,*,#15345,.F.);
#21430=ORIENTED_EDGE('',*,*,#15349,.F.);
#21431=ORIENTED_EDGE('',*,*,#15350,.T.);
#21432=ORIENTED_EDGE('',*,*,#15351,.T.);
#21433=ORIENTED_EDGE('',*,*,#15347,.F.);
#21434=ORIENTED_EDGE('',*,*,#15352,.F.);
#21435=ORIENTED_EDGE('',*,*,#15353,.T.);
#21436=ORIENTED_EDGE('',*,*,#15354,.T.);
#21437=ORIENTED_EDGE('',*,*,#15350,.F.);
#21438=ORIENTED_EDGE('',*,*,#15355,.F.);
#21439=ORIENTED_EDGE('',*,*,#15353,.F.);
#21440=ORIENTED_EDGE('',*,*,#15356,.T.);
#21441=ORIENTED_EDGE('',*,*,#15357,.T.);
#21442=ORIENTED_EDGE('',*,*,#15358,.F.);
#21443=ORIENTED_EDGE('',*,*,#14610,.F.);
#21444=ORIENTED_EDGE('',*,*,#14613,.F.);
#21445=ORIENTED_EDGE('',*,*,#15357,.F.);
#21446=ORIENTED_EDGE('',*,*,#15359,.T.);
#21447=ORIENTED_EDGE('',*,*,#15360,.T.);
#21448=ORIENTED_EDGE('',*,*,#15361,.F.);
#21449=ORIENTED_EDGE('',*,*,#15360,.F.);
#21450=ORIENTED_EDGE('',*,*,#15362,.T.);
#21451=ORIENTED_EDGE('',*,*,#15363,.T.);
#21452=ORIENTED_EDGE('',*,*,#15364,.F.);
#21453=ORIENTED_EDGE('',*,*,#15363,.F.);
#21454=ORIENTED_EDGE('',*,*,#15365,.T.);
#21455=ORIENTED_EDGE('',*,*,#15366,.T.);
#21456=ORIENTED_EDGE('',*,*,#15367,.F.);
#21457=ORIENTED_EDGE('',*,*,#15368,.T.);
#21458=ORIENTED_EDGE('',*,*,#15369,.T.);
#21459=ORIENTED_EDGE('',*,*,#15172,.T.);
#21460=ORIENTED_EDGE('',*,*,#15202,.T.);
#21461=ORIENTED_EDGE('',*,*,#15370,.F.);
#21462=ORIENTED_EDGE('',*,*,#15366,.F.);
#21463=ORIENTED_EDGE('',*,*,#15371,.T.);
#21464=ORIENTED_EDGE('',*,*,#15177,.F.);
#21465=ORIENTED_EDGE('',*,*,#15176,.F.);
#21466=ORIENTED_EDGE('',*,*,#15369,.F.);
#21467=ORIENTED_EDGE('',*,*,#15372,.T.);
#21468=ORIENTED_EDGE('',*,*,#15373,.F.);
#21469=ORIENTED_EDGE('',*,*,#14608,.T.);
#21470=ORIENTED_EDGE('',*,*,#15374,.T.);
#21471=ORIENTED_EDGE('',*,*,#15375,.T.);
#21472=ORIENTED_EDGE('',*,*,#15373,.T.);
#21473=ORIENTED_EDGE('',*,*,#15376,.T.);
#21474=ORIENTED_EDGE('',*,*,#15377,.F.);
#21475=ORIENTED_EDGE('',*,*,#15374,.F.);
#21476=ORIENTED_EDGE('',*,*,#15378,.T.);
#21477=ORIENTED_EDGE('',*,*,#15379,.T.);
#21478=ORIENTED_EDGE('',*,*,#15380,.F.);
#21479=ORIENTED_EDGE('',*,*,#14654,.F.);
#21480=ORIENTED_EDGE('',*,*,#15381,.T.);
#21481=ORIENTED_EDGE('',*,*,#15382,.F.);
#21482=ORIENTED_EDGE('',*,*,#15383,.F.);
#21483=ORIENTED_EDGE('',*,*,#15384,.T.);
#21484=ORIENTED_EDGE('',*,*,#15382,.T.);
#21485=ORIENTED_EDGE('',*,*,#15385,.T.);
#21486=ORIENTED_EDGE('',*,*,#15386,.T.);
#21487=ORIENTED_EDGE('',*,*,#15326,.F.);
#21488=ORIENTED_EDGE('',*,*,#15180,.F.);
#21489=ORIENTED_EDGE('',*,*,#15185,.T.);
#21490=ORIENTED_EDGE('',*,*,#15387,.T.);
#21491=ORIENTED_EDGE('',*,*,#15383,.T.);
#21492=ORIENTED_EDGE('',*,*,#14602,.T.);
#21493=ORIENTED_EDGE('',*,*,#15388,.F.);
#21494=ORIENTED_EDGE('',*,*,#15379,.F.);
#21495=ORIENTED_EDGE('',*,*,#15389,.T.);
#21496=ORIENTED_EDGE('',*,*,#15390,.T.);
#21497=ORIENTED_EDGE('',*,*,#15391,.F.);
#21498=ORIENTED_EDGE('',*,*,#15316,.F.);
#21499=ORIENTED_EDGE('',*,*,#15392,.F.);
#21500=ORIENTED_EDGE('',*,*,#15393,.T.);
#21501=ORIENTED_EDGE('',*,*,#15394,.F.);
#21502=ORIENTED_EDGE('',*,*,#15395,.F.);
#21503=ORIENTED_EDGE('',*,*,#15396,.F.);
#21504=ORIENTED_EDGE('',*,*,#15311,.T.);
#21505=ORIENTED_EDGE('',*,*,#15201,.F.);
#21506=ORIENTED_EDGE('',*,*,#15200,.F.);
#21507=ORIENTED_EDGE('',*,*,#15196,.T.);
#21508=ORIENTED_EDGE('',*,*,#14665,.T.);
#21509=ORIENTED_EDGE('',*,*,#15397,.T.);
#21510=ORIENTED_EDGE('',*,*,#15392,.T.);
#21511=ORIENTED_EDGE('',*,*,#15315,.T.);
#21512=ORIENTED_EDGE('',*,*,#15319,.T.);
#21513=ORIENTED_EDGE('',*,*,#15322,.T.);
#21514=ORIENTED_EDGE('',*,*,#15323,.T.);
#21515=ORIENTED_EDGE('',*,*,#15299,.F.);
#21516=ORIENTED_EDGE('',*,*,#15303,.T.);
#21517=ORIENTED_EDGE('',*,*,#15306,.T.);
#21518=ORIENTED_EDGE('',*,*,#15309,.T.);
#21519=ORIENTED_EDGE('',*,*,#15312,.T.);
#21520=ORIENTED_EDGE('',*,*,#15396,.T.);
#21521=ORIENTED_EDGE('',*,*,#15398,.T.);
#21522=ORIENTED_EDGE('',*,*,#15399,.T.);
#21523=ORIENTED_EDGE('',*,*,#15205,.T.);
#21524=ORIENTED_EDGE('',*,*,#15194,.F.);
#21525=ORIENTED_EDGE('',*,*,#15190,.F.);
#21526=ORIENTED_EDGE('',*,*,#15325,.T.);
#21527=ORIENTED_EDGE('',*,*,#15331,.T.);
#21528=ORIENTED_EDGE('',*,*,#15333,.T.);
#21529=ORIENTED_EDGE('',*,*,#15336,.F.);
#21530=ORIENTED_EDGE('',*,*,#15339,.F.);
#21531=ORIENTED_EDGE('',*,*,#15342,.F.);
#21532=ORIENTED_EDGE('',*,*,#15346,.T.);
#21533=ORIENTED_EDGE('',*,*,#15348,.F.);
#21534=ORIENTED_EDGE('',*,*,#15351,.F.);
#21535=ORIENTED_EDGE('',*,*,#15354,.F.);
#21536=ORIENTED_EDGE('',*,*,#15358,.T.);
#21537=ORIENTED_EDGE('',*,*,#15361,.T.);
#21538=ORIENTED_EDGE('',*,*,#15364,.T.);
#21539=ORIENTED_EDGE('',*,*,#15367,.T.);
#21540=ORIENTED_EDGE('',*,*,#15370,.T.);
#21541=ORIENTED_EDGE('',*,*,#15400,.F.);
#21542=ORIENTED_EDGE('',*,*,#15206,.T.);
#21543=ORIENTED_EDGE('',*,*,#15399,.F.);
#21544=ORIENTED_EDGE('',*,*,#15401,.F.);
#21545=ORIENTED_EDGE('',*,*,#15324,.T.);
#21546=ORIENTED_EDGE('',*,*,#15320,.T.);
#21547=ORIENTED_EDGE('',*,*,#15317,.T.);
#21548=ORIENTED_EDGE('',*,*,#15313,.T.);
#21549=ORIENTED_EDGE('',*,*,#15391,.T.);
#21550=ORIENTED_EDGE('',*,*,#15402,.T.);
#21551=ORIENTED_EDGE('',*,*,#15403,.T.);
#21552=ORIENTED_EDGE('',*,*,#15404,.T.);
#21553=ORIENTED_EDGE('',*,*,#15405,.T.);
#21554=ORIENTED_EDGE('',*,*,#15406,.T.);
#21555=ORIENTED_EDGE('',*,*,#15407,.T.);
#21556=ORIENTED_EDGE('',*,*,#15408,.T.);
#21557=ORIENTED_EDGE('',*,*,#15409,.T.);
#21558=ORIENTED_EDGE('',*,*,#15410,.T.);
#21559=ORIENTED_EDGE('',*,*,#15411,.T.);
#21560=ORIENTED_EDGE('',*,*,#15412,.T.);
#21561=ORIENTED_EDGE('',*,*,#15413,.T.);
#21562=ORIENTED_EDGE('',*,*,#15414,.T.);
#21563=ORIENTED_EDGE('',*,*,#15415,.T.);
#21564=ORIENTED_EDGE('',*,*,#15416,.T.);
#21565=ORIENTED_EDGE('',*,*,#15417,.T.);
#21566=ORIENTED_EDGE('',*,*,#15418,.T.);
#21567=ORIENTED_EDGE('',*,*,#15419,.T.);
#21568=ORIENTED_EDGE('',*,*,#15420,.T.);
#21569=ORIENTED_EDGE('',*,*,#15421,.T.);
#21570=ORIENTED_EDGE('',*,*,#15422,.T.);
#21571=ORIENTED_EDGE('',*,*,#15423,.T.);
#21572=ORIENTED_EDGE('',*,*,#15424,.T.);
#21573=ORIENTED_EDGE('',*,*,#15425,.T.);
#21574=ORIENTED_EDGE('',*,*,#15426,.T.);
#21575=ORIENTED_EDGE('',*,*,#15427,.T.);
#21576=ORIENTED_EDGE('',*,*,#15428,.T.);
#21577=ORIENTED_EDGE('',*,*,#15429,.T.);
#21578=ORIENTED_EDGE('',*,*,#15430,.T.);
#21579=ORIENTED_EDGE('',*,*,#15431,.T.);
#21580=ORIENTED_EDGE('',*,*,#15432,.T.);
#21581=ORIENTED_EDGE('',*,*,#15433,.T.);
#21582=ORIENTED_EDGE('',*,*,#15434,.T.);
#21583=ORIENTED_EDGE('',*,*,#15435,.T.);
#21584=ORIENTED_EDGE('',*,*,#15436,.T.);
#21585=ORIENTED_EDGE('',*,*,#15437,.T.);
#21586=ORIENTED_EDGE('',*,*,#15438,.T.);
#21587=ORIENTED_EDGE('',*,*,#15394,.T.);
#21588=ORIENTED_EDGE('',*,*,#15310,.T.);
#21589=ORIENTED_EDGE('',*,*,#15307,.T.);
#21590=ORIENTED_EDGE('',*,*,#15304,.T.);
#21591=ORIENTED_EDGE('',*,*,#15301,.T.);
#21592=ORIENTED_EDGE('',*,*,#15297,.F.);
#21593=ORIENTED_EDGE('',*,*,#15296,.F.);
#21594=ORIENTED_EDGE('',*,*,#15294,.F.);
#21595=ORIENTED_EDGE('',*,*,#15292,.F.);
#21596=ORIENTED_EDGE('',*,*,#15290,.F.);
#21597=ORIENTED_EDGE('',*,*,#15288,.F.);
#21598=ORIENTED_EDGE('',*,*,#15286,.F.);
#21599=ORIENTED_EDGE('',*,*,#15284,.F.);
#21600=ORIENTED_EDGE('',*,*,#15282,.F.);
#21601=ORIENTED_EDGE('',*,*,#15280,.F.);
#21602=ORIENTED_EDGE('',*,*,#15278,.F.);
#21603=ORIENTED_EDGE('',*,*,#15276,.F.);
#21604=ORIENTED_EDGE('',*,*,#15274,.F.);
#21605=ORIENTED_EDGE('',*,*,#15272,.F.);
#21606=ORIENTED_EDGE('',*,*,#15270,.F.);
#21607=ORIENTED_EDGE('',*,*,#15268,.F.);
#21608=ORIENTED_EDGE('',*,*,#15266,.F.);
#21609=ORIENTED_EDGE('',*,*,#15264,.F.);
#21610=ORIENTED_EDGE('',*,*,#15262,.F.);
#21611=ORIENTED_EDGE('',*,*,#15260,.F.);
#21612=ORIENTED_EDGE('',*,*,#15258,.F.);
#21613=ORIENTED_EDGE('',*,*,#15256,.F.);
#21614=ORIENTED_EDGE('',*,*,#15254,.F.);
#21615=ORIENTED_EDGE('',*,*,#15252,.F.);
#21616=ORIENTED_EDGE('',*,*,#15250,.F.);
#21617=ORIENTED_EDGE('',*,*,#15248,.F.);
#21618=ORIENTED_EDGE('',*,*,#15246,.F.);
#21619=ORIENTED_EDGE('',*,*,#15244,.F.);
#21620=ORIENTED_EDGE('',*,*,#15242,.F.);
#21621=ORIENTED_EDGE('',*,*,#15240,.F.);
#21622=ORIENTED_EDGE('',*,*,#15238,.F.);
#21623=ORIENTED_EDGE('',*,*,#15236,.F.);
#21624=ORIENTED_EDGE('',*,*,#15234,.F.);
#21625=ORIENTED_EDGE('',*,*,#15232,.F.);
#21626=ORIENTED_EDGE('',*,*,#15230,.F.);
#21627=ORIENTED_EDGE('',*,*,#15228,.F.);
#21628=ORIENTED_EDGE('',*,*,#15226,.F.);
#21629=ORIENTED_EDGE('',*,*,#15224,.F.);
#21630=ORIENTED_EDGE('',*,*,#15222,.F.);
#21631=ORIENTED_EDGE('',*,*,#15220,.F.);
#21632=ORIENTED_EDGE('',*,*,#15218,.F.);
#21633=ORIENTED_EDGE('',*,*,#15216,.F.);
#21634=ORIENTED_EDGE('',*,*,#15214,.F.);
#21635=ORIENTED_EDGE('',*,*,#15212,.F.);
#21636=ORIENTED_EDGE('',*,*,#15209,.F.);
#21637=ORIENTED_EDGE('',*,*,#15386,.F.);
#21638=ORIENTED_EDGE('',*,*,#15385,.F.);
#21639=ORIENTED_EDGE('',*,*,#15381,.F.);
#21640=ORIENTED_EDGE('',*,*,#14653,.F.);
#21641=ORIENTED_EDGE('',*,*,#15439,.F.);
#21642=ORIENTED_EDGE('',*,*,#15440,.F.);
#21643=ORIENTED_EDGE('',*,*,#15441,.F.);
#21644=ORIENTED_EDGE('',*,*,#15442,.F.);
#21645=ORIENTED_EDGE('',*,*,#15443,.F.);
#21646=ORIENTED_EDGE('',*,*,#15444,.T.);
#21647=ORIENTED_EDGE('',*,*,#15445,.F.);
#21648=ORIENTED_EDGE('',*,*,#15446,.T.);
#21649=ORIENTED_EDGE('',*,*,#15447,.F.);
#21650=ORIENTED_EDGE('',*,*,#15448,.F.);
#21651=ORIENTED_EDGE('',*,*,#15449,.F.);
#21652=ORIENTED_EDGE('',*,*,#15450,.F.);
#21653=ORIENTED_EDGE('',*,*,#15451,.F.);
#21654=ORIENTED_EDGE('',*,*,#15389,.F.);
#21655=ORIENTED_EDGE('',*,*,#15378,.F.);
#21656=ORIENTED_EDGE('',*,*,#15376,.F.);
#21657=ORIENTED_EDGE('',*,*,#15372,.F.);
#21658=ORIENTED_EDGE('',*,*,#15368,.F.);
#21659=ORIENTED_EDGE('',*,*,#15365,.F.);
#21660=ORIENTED_EDGE('',*,*,#15362,.F.);
#21661=ORIENTED_EDGE('',*,*,#15359,.F.);
#21662=ORIENTED_EDGE('',*,*,#15356,.F.);
#21663=ORIENTED_EDGE('',*,*,#15355,.T.);
#21664=ORIENTED_EDGE('',*,*,#15352,.T.);
#21665=ORIENTED_EDGE('',*,*,#15349,.T.);
#21666=ORIENTED_EDGE('',*,*,#15344,.F.);
#21667=ORIENTED_EDGE('',*,*,#15343,.T.);
#21668=ORIENTED_EDGE('',*,*,#15340,.T.);
#21669=ORIENTED_EDGE('',*,*,#15337,.T.);
#21670=ORIENTED_EDGE('',*,*,#15334,.F.);
#21671=ORIENTED_EDGE('',*,*,#15329,.F.);
#21672=ORIENTED_EDGE('',*,*,#15327,.F.);
#21673=ORIENTED_EDGE('',*,*,#15452,.F.);
#21674=ORIENTED_EDGE('',*,*,#15453,.T.);
#21675=ORIENTED_EDGE('',*,*,#15446,.F.);
#21676=ORIENTED_EDGE('',*,*,#15454,.F.);
#21677=ORIENTED_EDGE('',*,*,#15455,.T.);
#21678=ORIENTED_EDGE('',*,*,#15456,.T.);
#21679=ORIENTED_EDGE('',*,*,#15442,.T.);
#21680=ORIENTED_EDGE('',*,*,#15457,.F.);
#21681=ORIENTED_EDGE('',*,*,#15458,.T.);
#21682=ORIENTED_EDGE('',*,*,#15457,.T.);
#21683=ORIENTED_EDGE('',*,*,#15441,.T.);
#21684=ORIENTED_EDGE('',*,*,#15459,.F.);
#21685=ORIENTED_EDGE('',*,*,#14593,.F.);
#21686=ORIENTED_EDGE('',*,*,#15460,.T.);
#21687=ORIENTED_EDGE('',*,*,#15459,.T.);
#21688=ORIENTED_EDGE('',*,*,#15440,.T.);
#21689=ORIENTED_EDGE('',*,*,#15461,.F.);
#21690=ORIENTED_EDGE('',*,*,#15462,.T.);
#21691=ORIENTED_EDGE('',*,*,#15463,.F.);
#21692=ORIENTED_EDGE('',*,*,#15443,.T.);
#21693=ORIENTED_EDGE('',*,*,#15456,.F.);
#21694=ORIENTED_EDGE('',*,*,#15464,.F.);
#21695=ORIENTED_EDGE('',*,*,#15465,.T.);
#21696=ORIENTED_EDGE('',*,*,#15466,.F.);
#21697=ORIENTED_EDGE('',*,*,#15436,.F.);
#21698=ORIENTED_EDGE('',*,*,#15467,.F.);
#21699=ORIENTED_EDGE('',*,*,#15468,.T.);
#21700=ORIENTED_EDGE('',*,*,#15469,.F.);
#21701=ORIENTED_EDGE('',*,*,#15434,.F.);
#21702=ORIENTED_EDGE('',*,*,#15469,.T.);
#21703=ORIENTED_EDGE('',*,*,#15470,.T.);
#21704=ORIENTED_EDGE('',*,*,#15464,.T.);
#21705=ORIENTED_EDGE('',*,*,#15435,.F.);
#21706=ORIENTED_EDGE('',*,*,#15466,.T.);
#21707=ORIENTED_EDGE('',*,*,#15471,.T.);
#21708=ORIENTED_EDGE('',*,*,#15472,.T.);
#21709=ORIENTED_EDGE('',*,*,#15437,.F.);
#21710=ORIENTED_EDGE('',*,*,#15472,.F.);
#21711=ORIENTED_EDGE('',*,*,#15473,.T.);
#21712=ORIENTED_EDGE('',*,*,#15461,.T.);
#21713=ORIENTED_EDGE('',*,*,#15439,.T.);
#21714=ORIENTED_EDGE('',*,*,#14652,.T.);
#21715=ORIENTED_EDGE('',*,*,#14658,.T.);
#21716=ORIENTED_EDGE('',*,*,#15401,.T.);
#21717=ORIENTED_EDGE('',*,*,#15398,.F.);
#21718=ORIENTED_EDGE('',*,*,#15395,.T.);
#21719=ORIENTED_EDGE('',*,*,#15438,.F.);
#21720=ORIENTED_EDGE('',*,*,#15474,.T.);
#21721=ORIENTED_EDGE('',*,*,#15475,.F.);
#21722=ORIENTED_EDGE('',*,*,#15432,.F.);
#21723=ORIENTED_EDGE('',*,*,#15476,.F.);
#21724=ORIENTED_EDGE('',*,*,#15477,.T.);
#21725=ORIENTED_EDGE('',*,*,#15478,.F.);
#21726=ORIENTED_EDGE('',*,*,#15430,.F.);
#21727=ORIENTED_EDGE('',*,*,#15479,.F.);
#21728=ORIENTED_EDGE('',*,*,#15478,.T.);
#21729=ORIENTED_EDGE('',*,*,#15480,.T.);
#21730=ORIENTED_EDGE('',*,*,#15476,.T.);
#21731=ORIENTED_EDGE('',*,*,#15431,.F.);
#21732=ORIENTED_EDGE('',*,*,#15481,.T.);
#21733=ORIENTED_EDGE('',*,*,#15482,.F.);
#21734=ORIENTED_EDGE('',*,*,#15428,.F.);
#21735=ORIENTED_EDGE('',*,*,#15483,.F.);
#21736=ORIENTED_EDGE('',*,*,#15484,.T.);
#21737=ORIENTED_EDGE('',*,*,#15485,.F.);
#21738=ORIENTED_EDGE('',*,*,#15426,.F.);
#21739=ORIENTED_EDGE('',*,*,#15486,.F.);
#21740=ORIENTED_EDGE('',*,*,#15485,.T.);
#21741=ORIENTED_EDGE('',*,*,#15487,.T.);
#21742=ORIENTED_EDGE('',*,*,#15483,.T.);
#21743=ORIENTED_EDGE('',*,*,#15427,.F.);
#21744=ORIENTED_EDGE('',*,*,#15482,.T.);
#21745=ORIENTED_EDGE('',*,*,#15488,.T.);
#21746=ORIENTED_EDGE('',*,*,#15479,.T.);
#21747=ORIENTED_EDGE('',*,*,#15429,.F.);
#21748=ORIENTED_EDGE('',*,*,#15489,.T.);
#21749=ORIENTED_EDGE('',*,*,#15490,.F.);
#21750=ORIENTED_EDGE('',*,*,#15424,.F.);
#21751=ORIENTED_EDGE('',*,*,#15491,.F.);
#21752=ORIENTED_EDGE('',*,*,#15492,.T.);
#21753=ORIENTED_EDGE('',*,*,#15493,.F.);
#21754=ORIENTED_EDGE('',*,*,#15422,.F.);
#21755=ORIENTED_EDGE('',*,*,#15494,.F.);
#21756=ORIENTED_EDGE('',*,*,#15493,.T.);
#21757=ORIENTED_EDGE('',*,*,#15495,.T.);
#21758=ORIENTED_EDGE('',*,*,#15491,.T.);
#21759=ORIENTED_EDGE('',*,*,#15423,.F.);
#21760=ORIENTED_EDGE('',*,*,#15496,.F.);
#21761=ORIENTED_EDGE('',*,*,#15497,.T.);
#21762=ORIENTED_EDGE('',*,*,#15498,.T.);
#21763=ORIENTED_EDGE('',*,*,#15420,.F.);
#21764=ORIENTED_EDGE('',*,*,#15498,.F.);
#21765=ORIENTED_EDGE('',*,*,#15499,.T.);
#21766=ORIENTED_EDGE('',*,*,#15494,.T.);
#21767=ORIENTED_EDGE('',*,*,#15421,.F.);
#21768=ORIENTED_EDGE('',*,*,#15500,.T.);
#21769=ORIENTED_EDGE('',*,*,#15501,.F.);
#21770=ORIENTED_EDGE('',*,*,#15418,.F.);
#21771=ORIENTED_EDGE('',*,*,#15502,.F.);
#21772=ORIENTED_EDGE('',*,*,#15503,.T.);
#21773=ORIENTED_EDGE('',*,*,#15504,.F.);
#21774=ORIENTED_EDGE('',*,*,#15416,.F.);
#21775=ORIENTED_EDGE('',*,*,#15505,.F.);
#21776=ORIENTED_EDGE('',*,*,#15504,.T.);
#21777=ORIENTED_EDGE('',*,*,#15506,.T.);
#21778=ORIENTED_EDGE('',*,*,#15502,.T.);
#21779=ORIENTED_EDGE('',*,*,#15417,.F.);
#21780=ORIENTED_EDGE('',*,*,#15507,.T.);
#21781=ORIENTED_EDGE('',*,*,#15508,.F.);
#21782=ORIENTED_EDGE('',*,*,#15414,.F.);
#21783=ORIENTED_EDGE('',*,*,#15509,.F.);
#21784=ORIENTED_EDGE('',*,*,#15510,.T.);
#21785=ORIENTED_EDGE('',*,*,#15511,.F.);
#21786=ORIENTED_EDGE('',*,*,#15412,.F.);
#21787=ORIENTED_EDGE('',*,*,#15512,.F.);
#21788=ORIENTED_EDGE('',*,*,#15511,.T.);
#21789=ORIENTED_EDGE('',*,*,#15513,.T.);
#21790=ORIENTED_EDGE('',*,*,#15509,.T.);
#21791=ORIENTED_EDGE('',*,*,#15413,.F.);
#21792=ORIENTED_EDGE('',*,*,#15508,.T.);
#21793=ORIENTED_EDGE('',*,*,#15514,.T.);
#21794=ORIENTED_EDGE('',*,*,#15505,.T.);
#21795=ORIENTED_EDGE('',*,*,#15415,.F.);
#21796=ORIENTED_EDGE('',*,*,#15501,.T.);
#21797=ORIENTED_EDGE('',*,*,#15515,.T.);
#21798=ORIENTED_EDGE('',*,*,#15496,.T.);
#21799=ORIENTED_EDGE('',*,*,#15419,.F.);
#21800=ORIENTED_EDGE('',*,*,#15516,.T.);
#21801=ORIENTED_EDGE('',*,*,#15517,.F.);
#21802=ORIENTED_EDGE('',*,*,#15410,.F.);
#21803=ORIENTED_EDGE('',*,*,#15518,.F.);
#21804=ORIENTED_EDGE('',*,*,#15519,.T.);
#21805=ORIENTED_EDGE('',*,*,#15520,.F.);
#21806=ORIENTED_EDGE('',*,*,#15408,.F.);
#21807=ORIENTED_EDGE('',*,*,#15521,.F.);
#21808=ORIENTED_EDGE('',*,*,#15520,.T.);
#21809=ORIENTED_EDGE('',*,*,#15522,.T.);
#21810=ORIENTED_EDGE('',*,*,#15518,.T.);
#21811=ORIENTED_EDGE('',*,*,#15409,.F.);
#21812=ORIENTED_EDGE('',*,*,#15523,.F.);
#21813=ORIENTED_EDGE('',*,*,#15524,.T.);
#21814=ORIENTED_EDGE('',*,*,#15525,.F.);
#21815=ORIENTED_EDGE('',*,*,#15406,.F.);
#21816=ORIENTED_EDGE('',*,*,#15526,.F.);
#21817=ORIENTED_EDGE('',*,*,#15527,.T.);
#21818=ORIENTED_EDGE('',*,*,#15528,.F.);
#21819=ORIENTED_EDGE('',*,*,#15404,.F.);
#21820=ORIENTED_EDGE('',*,*,#15529,.T.);
#21821=ORIENTED_EDGE('',*,*,#15530,.T.);
#21822=ORIENTED_EDGE('',*,*,#15450,.T.);
#21823=ORIENTED_EDGE('',*,*,#15531,.F.);
#21824=ORIENTED_EDGE('',*,*,#15532,.T.);
#21825=ORIENTED_EDGE('',*,*,#15531,.T.);
#21826=ORIENTED_EDGE('',*,*,#15449,.T.);
#21827=ORIENTED_EDGE('',*,*,#15533,.F.);
#21828=ORIENTED_EDGE('',*,*,#14596,.F.);
#21829=ORIENTED_EDGE('',*,*,#15534,.T.);
#21830=ORIENTED_EDGE('',*,*,#15533,.T.);
#21831=ORIENTED_EDGE('',*,*,#15448,.T.);
#21832=ORIENTED_EDGE('',*,*,#15535,.F.);
#21833=ORIENTED_EDGE('',*,*,#15536,.T.);
#21834=ORIENTED_EDGE('',*,*,#15535,.T.);
#21835=ORIENTED_EDGE('',*,*,#15447,.T.);
#21836=ORIENTED_EDGE('',*,*,#15453,.F.);
#21837=ORIENTED_EDGE('',*,*,#15530,.F.);
#21838=ORIENTED_EDGE('',*,*,#15537,.T.);
#21839=ORIENTED_EDGE('',*,*,#15538,.T.);
#21840=ORIENTED_EDGE('',*,*,#15402,.F.);
#21841=ORIENTED_EDGE('',*,*,#15393,.F.);
#21842=ORIENTED_EDGE('',*,*,#15397,.F.);
#21843=ORIENTED_EDGE('',*,*,#14664,.F.);
#21844=ORIENTED_EDGE('',*,*,#14660,.F.);
#21845=ORIENTED_EDGE('',*,*,#15390,.F.);
#21846=ORIENTED_EDGE('',*,*,#15451,.T.);
#21847=ORIENTED_EDGE('',*,*,#15538,.F.);
#21848=ORIENTED_EDGE('',*,*,#15539,.T.);
#21849=ORIENTED_EDGE('',*,*,#15526,.T.);
#21850=ORIENTED_EDGE('',*,*,#15403,.F.);
#21851=ORIENTED_EDGE('',*,*,#15528,.T.);
#21852=ORIENTED_EDGE('',*,*,#15540,.T.);
#21853=ORIENTED_EDGE('',*,*,#15523,.T.);
#21854=ORIENTED_EDGE('',*,*,#15405,.F.);
#21855=ORIENTED_EDGE('',*,*,#15525,.T.);
#21856=ORIENTED_EDGE('',*,*,#15541,.T.);
#21857=ORIENTED_EDGE('',*,*,#15521,.T.);
#21858=ORIENTED_EDGE('',*,*,#15407,.F.);
#21859=ORIENTED_EDGE('',*,*,#15517,.T.);
#21860=ORIENTED_EDGE('',*,*,#15542,.T.);
#21861=ORIENTED_EDGE('',*,*,#15512,.T.);
#21862=ORIENTED_EDGE('',*,*,#15411,.F.);
#21863=ORIENTED_EDGE('',*,*,#15490,.T.);
#21864=ORIENTED_EDGE('',*,*,#15543,.T.);
#21865=ORIENTED_EDGE('',*,*,#15486,.T.);
#21866=ORIENTED_EDGE('',*,*,#15425,.F.);
#21867=ORIENTED_EDGE('',*,*,#15475,.T.);
#21868=ORIENTED_EDGE('',*,*,#15544,.T.);
#21869=ORIENTED_EDGE('',*,*,#15467,.T.);
#21870=ORIENTED_EDGE('',*,*,#15433,.F.);
#21871=ORIENTED_EDGE('',*,*,#15444,.F.);
#21872=ORIENTED_EDGE('',*,*,#15463,.T.);
#21873=ORIENTED_EDGE('',*,*,#15545,.F.);
#21874=ORIENTED_EDGE('',*,*,#15546,.F.);
#21875=ORIENTED_EDGE('',*,*,#15445,.T.);
#21876=ORIENTED_EDGE('',*,*,#15546,.T.);
#21877=ORIENTED_EDGE('',*,*,#15547,.T.);
#21878=ORIENTED_EDGE('',*,*,#15454,.T.);
#21879=ORIENTED_EDGE('',*,*,#14599,.F.);
#21880=ORIENTED_EDGE('',*,*,#15547,.F.);
#21881=ORIENTED_EDGE('',*,*,#15545,.T.);
#21882=ORIENTED_EDGE('',*,*,#15462,.F.);
#21883=ORIENTED_EDGE('',*,*,#15455,.F.);
#21884=ORIENTED_EDGE('',*,*,#15458,.F.);
#21885=ORIENTED_EDGE('',*,*,#15460,.F.);
#21886=ORIENTED_EDGE('',*,*,#15473,.F.);
#21887=ORIENTED_EDGE('',*,*,#15471,.F.);
#21888=ORIENTED_EDGE('',*,*,#15465,.F.);
#21889=ORIENTED_EDGE('',*,*,#15470,.F.);
#21890=ORIENTED_EDGE('',*,*,#15468,.F.);
#21891=ORIENTED_EDGE('',*,*,#15544,.F.);
#21892=ORIENTED_EDGE('',*,*,#15474,.F.);
#21893=ORIENTED_EDGE('',*,*,#15480,.F.);
#21894=ORIENTED_EDGE('',*,*,#15477,.F.);
#21895=ORIENTED_EDGE('',*,*,#15488,.F.);
#21896=ORIENTED_EDGE('',*,*,#15481,.F.);
#21897=ORIENTED_EDGE('',*,*,#15487,.F.);
#21898=ORIENTED_EDGE('',*,*,#15484,.F.);
#21899=ORIENTED_EDGE('',*,*,#15543,.F.);
#21900=ORIENTED_EDGE('',*,*,#15489,.F.);
#21901=ORIENTED_EDGE('',*,*,#15495,.F.);
#21902=ORIENTED_EDGE('',*,*,#15492,.F.);
#21903=ORIENTED_EDGE('',*,*,#15499,.F.);
#21904=ORIENTED_EDGE('',*,*,#15497,.F.);
#21905=ORIENTED_EDGE('',*,*,#15515,.F.);
#21906=ORIENTED_EDGE('',*,*,#15500,.F.);
#21907=ORIENTED_EDGE('',*,*,#15506,.F.);
#21908=ORIENTED_EDGE('',*,*,#15503,.F.);
#21909=ORIENTED_EDGE('',*,*,#15514,.F.);
#21910=ORIENTED_EDGE('',*,*,#15507,.F.);
#21911=ORIENTED_EDGE('',*,*,#15513,.F.);
#21912=ORIENTED_EDGE('',*,*,#15510,.F.);
#21913=ORIENTED_EDGE('',*,*,#15542,.F.);
#21914=ORIENTED_EDGE('',*,*,#15516,.F.);
#21915=ORIENTED_EDGE('',*,*,#15522,.F.);
#21916=ORIENTED_EDGE('',*,*,#15519,.F.);
#21917=ORIENTED_EDGE('',*,*,#15541,.F.);
#21918=ORIENTED_EDGE('',*,*,#15524,.F.);
#21919=ORIENTED_EDGE('',*,*,#15540,.F.);
#21920=ORIENTED_EDGE('',*,*,#15527,.F.);
#21921=ORIENTED_EDGE('',*,*,#15539,.F.);
#21922=ORIENTED_EDGE('',*,*,#15537,.F.);
#21923=ORIENTED_EDGE('',*,*,#15529,.F.);
#21924=ORIENTED_EDGE('',*,*,#15532,.F.);
#21925=ORIENTED_EDGE('',*,*,#15534,.F.);
#21926=ORIENTED_EDGE('',*,*,#15536,.F.);
#21927=ORIENTED_EDGE('',*,*,#15452,.T.);
#21928=ORIENTED_EDGE('',*,*,#14942,.T.);
#21929=ORIENTED_EDGE('',*,*,#14940,.T.);
#21930=ORIENTED_EDGE('',*,*,#14938,.T.);
#21931=ORIENTED_EDGE('',*,*,#14936,.T.);
#21932=ORIENTED_EDGE('',*,*,#14934,.T.);
#21933=ORIENTED_EDGE('',*,*,#14932,.T.);
#21934=ORIENTED_EDGE('',*,*,#14930,.T.);
#21935=ORIENTED_EDGE('',*,*,#14928,.T.);
#21936=ORIENTED_EDGE('',*,*,#14926,.T.);
#21937=ORIENTED_EDGE('',*,*,#14924,.T.);
#21938=ORIENTED_EDGE('',*,*,#14922,.T.);
#21939=ORIENTED_EDGE('',*,*,#14920,.T.);
#21940=ORIENTED_EDGE('',*,*,#14918,.T.);
#21941=ORIENTED_EDGE('',*,*,#14916,.T.);
#21942=ORIENTED_EDGE('',*,*,#14914,.T.);
#21943=ORIENTED_EDGE('',*,*,#14912,.T.);
#21944=ORIENTED_EDGE('',*,*,#14910,.T.);
#21945=ORIENTED_EDGE('',*,*,#14908,.T.);
#21946=ORIENTED_EDGE('',*,*,#14906,.T.);
#21947=ORIENTED_EDGE('',*,*,#14904,.T.);
#21948=ORIENTED_EDGE('',*,*,#14902,.T.);
#21949=ORIENTED_EDGE('',*,*,#14900,.T.);
#21950=ORIENTED_EDGE('',*,*,#14898,.T.);
#21951=ORIENTED_EDGE('',*,*,#14896,.T.);
#21952=ORIENTED_EDGE('',*,*,#14894,.T.);
#21953=ORIENTED_EDGE('',*,*,#14892,.T.);
#21954=ORIENTED_EDGE('',*,*,#14890,.T.);
#21955=ORIENTED_EDGE('',*,*,#14888,.T.);
#21956=ORIENTED_EDGE('',*,*,#14886,.T.);
#21957=ORIENTED_EDGE('',*,*,#14884,.T.);
#21958=ORIENTED_EDGE('',*,*,#14882,.T.);
#21959=ORIENTED_EDGE('',*,*,#14880,.T.);
#21960=ORIENTED_EDGE('',*,*,#14878,.T.);
#21961=ORIENTED_EDGE('',*,*,#14876,.T.);
#21962=ORIENTED_EDGE('',*,*,#14874,.T.);
#21963=ORIENTED_EDGE('',*,*,#14872,.T.);
#21964=ORIENTED_EDGE('',*,*,#14870,.T.);
#21965=ORIENTED_EDGE('',*,*,#14868,.T.);
#21966=ORIENTED_EDGE('',*,*,#14866,.T.);
#21967=ORIENTED_EDGE('',*,*,#14864,.T.);
#21968=ORIENTED_EDGE('',*,*,#14862,.T.);
#21969=ORIENTED_EDGE('',*,*,#14860,.T.);
#21970=ORIENTED_EDGE('',*,*,#14858,.T.);
#21971=ORIENTED_EDGE('',*,*,#14855,.T.);
#21972=ORIENTED_EDGE('',*,*,#14947,.T.);
#21973=ORIENTED_EDGE('',*,*,#15012,.F.);
#21974=ORIENTED_EDGE('',*,*,#15548,.F.);
#21975=ORIENTED_EDGE('',*,*,#15549,.T.);
#21976=ORIENTED_EDGE('',*,*,#14948,.T.);
#21977=ORIENTED_EDGE('',*,*,#15549,.F.);
#21978=ORIENTED_EDGE('',*,*,#15550,.F.);
#21979=ORIENTED_EDGE('',*,*,#15551,.T.);
#21980=ORIENTED_EDGE('',*,*,#14949,.T.);
#21981=ORIENTED_EDGE('',*,*,#15551,.F.);
#21982=ORIENTED_EDGE('',*,*,#15552,.F.);
#21983=ORIENTED_EDGE('',*,*,#15015,.T.);
#21984=ORIENTED_EDGE('',*,*,#15011,.T.);
#21985=ORIENTED_EDGE('',*,*,#15552,.T.);
#21986=ORIENTED_EDGE('',*,*,#15550,.T.);
#21987=ORIENTED_EDGE('',*,*,#15548,.T.);
#21988=ORIENTED_EDGE('',*,*,#15203,.F.);
#21989=ORIENTED_EDGE('',*,*,#15114,.F.);
#21990=ORIENTED_EDGE('',*,*,#15187,.T.);
#21991=ORIENTED_EDGE('',*,*,#14661,.T.);
#21992=ORIENTED_EDGE('',*,*,#14663,.T.);
#21993=ORIENTED_EDGE('',*,*,#15195,.T.);
#21994=ORIENTED_EDGE('',*,*,#15199,.F.);
#21995=ORIENTED_EDGE('',*,*,#15371,.F.);
#21996=ORIENTED_EDGE('',*,*,#15375,.F.);
#21997=ORIENTED_EDGE('',*,*,#15377,.T.);
#21998=ORIENTED_EDGE('',*,*,#15388,.T.);
#21999=ORIENTED_EDGE('',*,*,#14659,.T.);
#22000=ORIENTED_EDGE('',*,*,#15186,.T.);
#22001=ORIENTED_EDGE('',*,*,#15178,.F.);
#22002=ORIENTED_EDGE('',*,*,#15188,.F.);
#22003=ORIENTED_EDGE('',*,*,#15193,.F.);
#22004=ORIENTED_EDGE('',*,*,#15204,.T.);
#22005=ORIENTED_EDGE('',*,*,#15400,.T.);
#22006=ORIENTED_EDGE('',*,*,#14657,.T.);
#22007=ORIENTED_EDGE('',*,*,#15208,.T.);
#22008=ORIENTED_EDGE('',*,*,#15117,.F.);
#22009=ORIENTED_EDGE('',*,*,#15207,.T.);
#22010=ORIENTED_EDGE('',*,*,#14655,.T.);
#22011=ORIENTED_EDGE('',*,*,#14651,.T.);
#22012=ORIENTED_EDGE('',*,*,#15380,.T.);
#22013=ORIENTED_EDGE('',*,*,#15384,.F.);
#22014=ORIENTED_EDGE('',*,*,#15387,.F.);
#22015=ORIENTED_EDGE('',*,*,#15184,.F.);
#22996=CYLINDRICAL_SURFACE('',#26508,2.5);
#22997=CYLINDRICAL_SURFACE('',#26511,2.5);
#22998=CYLINDRICAL_SURFACE('',#26514,3.65);
#22999=CYLINDRICAL_SURFACE('',#26519,3.32349999999999);
#23000=CYLINDRICAL_SURFACE('',#26522,3.3235);
#23001=CYLINDRICAL_SURFACE('',#26525,3.32349999999999);
#23002=CYLINDRICAL_SURFACE('',#26528,3.3235);
#23003=CYLINDRICAL_SURFACE('',#26531,2.5);
#23004=CYLINDRICAL_SURFACE('',#26534,2.5);
#23005=CYLINDRICAL_SURFACE('',#26537,3.65);
#23006=CYLINDRICAL_SURFACE('',#26540,0.500000000000006);
#23007=CYLINDRICAL_SURFACE('',#26546,0.5);
#23008=CYLINDRICAL_SURFACE('',#26552,4.);
#23009=CYLINDRICAL_SURFACE('',#26554,4.99995);
#23010=CYLINDRICAL_SURFACE('',#26584,2.3);
#23011=CYLINDRICAL_SURFACE('',#26587,2.3);
#23012=CYLINDRICAL_SURFACE('',#26590,2.3);
#23013=CYLINDRICAL_SURFACE('',#26593,2.3);
#23014=CYLINDRICAL_SURFACE('',#26596,0.5);
#23015=CYLINDRICAL_SURFACE('',#26599,0.5);
#23016=CYLINDRICAL_SURFACE('',#26602,0.5);
#23017=CYLINDRICAL_SURFACE('',#26605,0.5);
#23018=CYLINDRICAL_SURFACE('',#26608,0.5);
#23019=CYLINDRICAL_SURFACE('',#26611,0.5);
#23020=CYLINDRICAL_SURFACE('',#26614,0.5);
#23021=CYLINDRICAL_SURFACE('',#26617,0.5);
#23022=CYLINDRICAL_SURFACE('',#26620,0.5);
#23023=CYLINDRICAL_SURFACE('',#26623,0.5);
#23024=CYLINDRICAL_SURFACE('',#26626,0.5);
#23025=CYLINDRICAL_SURFACE('',#26629,0.5);
#23026=CYLINDRICAL_SURFACE('',#26632,0.5);
#23027=CYLINDRICAL_SURFACE('',#26635,0.5);
#23028=CYLINDRICAL_SURFACE('',#26638,0.5);
#23029=CYLINDRICAL_SURFACE('',#26641,0.5);
#23030=CYLINDRICAL_SURFACE('',#26682,0.450000000000001);
#23031=CYLINDRICAL_SURFACE('',#26685,0.450000000000001);
#23032=CYLINDRICAL_SURFACE('',#26688,0.55);
#23033=CYLINDRICAL_SURFACE('',#26690,2.25);
#23034=CYLINDRICAL_SURFACE('',#26692,0.549999999999998);
#23035=CYLINDRICAL_SURFACE('',#26695,0.55);
#23036=CYLINDRICAL_SURFACE('',#26698,0.55);
#23037=CYLINDRICAL_SURFACE('',#26701,0.55);
#23038=CYLINDRICAL_SURFACE('',#26703,2.25);
#23039=CYLINDRICAL_SURFACE('',#26705,0.55);
#23040=CYLINDRICAL_SURFACE('',#26710,0.550000000000001);
#23041=CYLINDRICAL_SURFACE('',#26712,2.25);
#23042=CYLINDRICAL_SURFACE('',#26714,0.550000000000002);
#23043=CYLINDRICAL_SURFACE('',#26717,0.55);
#23044=CYLINDRICAL_SURFACE('',#26720,0.55);
#23045=CYLINDRICAL_SURFACE('',#26723,0.55);
#23046=CYLINDRICAL_SURFACE('',#26725,2.25);
#23047=CYLINDRICAL_SURFACE('',#26727,0.55);
#23048=CYLINDRICAL_SURFACE('',#26730,0.450000000000001);
#23049=CYLINDRICAL_SURFACE('',#26733,0.450000000000001);
#23050=CYLINDRICAL_SURFACE('',#26772,0.5);
#23051=CYLINDRICAL_SURFACE('',#26787,0.5);
#23052=CYLINDRICAL_SURFACE('',#26790,0.5);
#23053=CYLINDRICAL_SURFACE('',#26793,0.5);
#23054=CYLINDRICAL_SURFACE('',#26795,2.3);
#23055=CYLINDRICAL_SURFACE('',#26797,0.5);
#23056=CYLINDRICAL_SURFACE('',#26800,0.5);
#23057=CYLINDRICAL_SURFACE('',#26803,0.5);
#23058=CYLINDRICAL_SURFACE('',#26806,0.5);
#23059=CYLINDRICAL_SURFACE('',#26808,2.3);
#23060=CYLINDRICAL_SURFACE('',#26810,0.5);
#23061=CYLINDRICAL_SURFACE('',#26815,0.5);
#23062=CYLINDRICAL_SURFACE('',#26817,2.3);
#23063=CYLINDRICAL_SURFACE('',#26819,0.5);
#23064=CYLINDRICAL_SURFACE('',#26822,0.5);
#23065=CYLINDRICAL_SURFACE('',#26825,0.5);
#23066=CYLINDRICAL_SURFACE('',#26828,0.5);
#23067=CYLINDRICAL_SURFACE('',#26830,2.3);
#23068=CYLINDRICAL_SURFACE('',#26832,0.5);
#23069=CYLINDRICAL_SURFACE('',#26835,0.5);
#23070=CYLINDRICAL_SURFACE('',#26838,0.5);
#23071=CYLINDRICAL_SURFACE('',#26846,0.500000000000006);
#23072=CYLINDRICAL_SURFACE('',#26848,2.);
#23073=CYLINDRICAL_SURFACE('',#26856,2.);
#23074=CYLINDRICAL_SURFACE('',#26912,0.450000000000001);
#23075=CYLINDRICAL_SURFACE('',#26915,0.450000000000001);
#23076=CYLINDRICAL_SURFACE('',#26918,0.55);
#23077=CYLINDRICAL_SURFACE('',#26920,2.25);
#23078=CYLINDRICAL_SURFACE('',#26922,0.55);
#23079=CYLINDRICAL_SURFACE('',#26925,0.55);
#23080=CYLINDRICAL_SURFACE('',#26928,0.55);
#23081=CYLINDRICAL_SURFACE('',#26931,0.550000000000002);
#23082=CYLINDRICAL_SURFACE('',#26933,2.25);
#23083=CYLINDRICAL_SURFACE('',#26935,0.55);
#23084=CYLINDRICAL_SURFACE('',#26940,0.55);
#23085=CYLINDRICAL_SURFACE('',#26942,2.25);
#23086=CYLINDRICAL_SURFACE('',#26944,0.55);
#23087=CYLINDRICAL_SURFACE('',#26947,0.55);
#23088=CYLINDRICAL_SURFACE('',#26950,0.55);
#23089=CYLINDRICAL_SURFACE('',#26953,0.549999999999998);
#23090=CYLINDRICAL_SURFACE('',#26955,2.25);
#23091=CYLINDRICAL_SURFACE('',#26957,0.550000000000001);
#23092=CYLINDRICAL_SURFACE('',#26960,0.450000000000001);
#23093=CYLINDRICAL_SURFACE('',#26963,0.450000000000001);
#23094=CYLINDRICAL_SURFACE('',#27034,0.5);
#23095=CYLINDRICAL_SURFACE('',#27036,0.5);
#23096=CYLINDRICAL_SURFACE('',#27041,0.5);
#23097=CYLINDRICAL_SURFACE('',#27043,0.5);
#23098=CYLINDRICAL_SURFACE('',#27045,2.3);
#23099=CYLINDRICAL_SURFACE('',#27047,0.5);
#23100=CYLINDRICAL_SURFACE('',#27049,0.5);
#23101=CYLINDRICAL_SURFACE('',#27053,0.5);
#23102=CYLINDRICAL_SURFACE('',#27055,0.5);
#23103=CYLINDRICAL_SURFACE('',#27057,2.3);
#23104=CYLINDRICAL_SURFACE('',#27061,0.5);
#23105=CYLINDRICAL_SURFACE('',#27063,0.5);
#23106=CYLINDRICAL_SURFACE('',#27065,2.3);
#23107=CYLINDRICAL_SURFACE('',#27067,0.5);
#23108=CYLINDRICAL_SURFACE('',#27069,0.5);
#23109=CYLINDRICAL_SURFACE('',#27074,0.5);
#23110=CYLINDRICAL_SURFACE('',#27076,0.5);
#23111=CYLINDRICAL_SURFACE('',#27078,2.3);
#23112=CYLINDRICAL_SURFACE('',#27080,0.5);
#23113=CYLINDRICAL_SURFACE('',#27082,0.5);
#23114=CYLINDRICAL_SURFACE('',#27099,4.99995);
#23115=CYLINDRICAL_SURFACE('',#27103,5.5);
#23116=CYLINDRICAL_SURFACE('',#27104,5.50000000000001);
#23117=CYLINDRICAL_SURFACE('',#27105,5.5);
#23118=CYLINDRICAL_SURFACE('',#27106,5.49999999999999);
#24014=ADVANCED_FACE('',(#3022),#22996,.F.);
#24015=ADVANCED_FACE('',(#3023),#22997,.F.);
#24016=ADVANCED_FACE('',(#3024),#22998,.F.);
#24017=ADVANCED_FACE('',(#3025),#2124,.F.);
#24018=ADVANCED_FACE('',(#3026),#2125,.F.);
#24019=ADVANCED_FACE('',(#3027),#22999,.F.);
#24020=ADVANCED_FACE('',(#3028),#23000,.F.);
#24021=ADVANCED_FACE('',(#3029),#23001,.F.);
#24022=ADVANCED_FACE('',(#3030),#23002,.F.);
#24023=ADVANCED_FACE('',(#3031),#23003,.F.);
#24024=ADVANCED_FACE('',(#3032),#23004,.F.);
#24025=ADVANCED_FACE('',(#3033),#23005,.F.);
#24026=ADVANCED_FACE('',(#3034),#23006,.F.);
#24027=ADVANCED_FACE('',(#3035),#2126,.F.);
#24028=ADVANCED_FACE('',(#3036),#2127,.F.);
#24029=ADVANCED_FACE('',(#3037),#23007,.F.);
#24030=ADVANCED_FACE('',(#3038),#252,.F.);
#24031=ADVANCED_FACE('',(#3039),#23008,.T.);
#24032=ADVANCED_FACE('',(#3040),#23009,.F.);
#24033=ADVANCED_FACE('',(#3041),#1788,.T.);
#24034=ADVANCED_FACE('',(#3042),#1789,.T.);
#24035=ADVANCED_FACE('',(#3043),#1790,.T.);
#24036=ADVANCED_FACE('',(#3044),#1791,.T.);
#24037=ADVANCED_FACE('',(#3045),#1792,.T.);
#24038=ADVANCED_FACE('',(#3046),#1793,.T.);
#24039=ADVANCED_FACE('',(#3047),#1794,.T.);
#24040=ADVANCED_FACE('',(#3048),#1795,.T.);
#24041=ADVANCED_FACE('',(#3049),#1796,.T.);
#24042=ADVANCED_FACE('',(#3050),#1797,.T.);
#24043=ADVANCED_FACE('',(#3051),#1798,.T.);
#24044=ADVANCED_FACE('',(#3052),#1799,.T.);
#24045=ADVANCED_FACE('',(#3053),#1800,.T.);
#24046=ADVANCED_FACE('',(#3054),#1801,.T.);
#24047=ADVANCED_FACE('',(#3055),#1802,.T.);
#24048=ADVANCED_FACE('',(#3056),#1803,.T.);
#24049=ADVANCED_FACE('',(#3057),#1804,.T.);
#24050=ADVANCED_FACE('',(#3058),#1805,.T.);
#24051=ADVANCED_FACE('',(#3059),#1806,.T.);
#24052=ADVANCED_FACE('',(#3060),#1807,.T.);
#24053=ADVANCED_FACE('',(#3061),#1808,.T.);
#24054=ADVANCED_FACE('',(#3062),#23010,.T.);
#24055=ADVANCED_FACE('',(#3063),#23011,.T.);
#24056=ADVANCED_FACE('',(#3064),#23012,.T.);
#24057=ADVANCED_FACE('',(#3065),#23013,.T.);
#24058=ADVANCED_FACE('',(#3066),#23014,.T.);
#24059=ADVANCED_FACE('',(#3067),#23015,.T.);
#24060=ADVANCED_FACE('',(#3068),#23016,.F.);
#24061=ADVANCED_FACE('',(#3069),#23017,.F.);
#24062=ADVANCED_FACE('',(#3070),#23018,.F.);
#24063=ADVANCED_FACE('',(#3071),#23019,.F.);
#24064=ADVANCED_FACE('',(#3072),#23020,.F.);
#24065=ADVANCED_FACE('',(#3073),#23021,.F.);
#24066=ADVANCED_FACE('',(#3074),#23022,.T.);
#24067=ADVANCED_FACE('',(#3075),#23023,.T.);
#24068=ADVANCED_FACE('',(#3076),#23024,.F.);
#24069=ADVANCED_FACE('',(#3077),#23025,.F.);
#24070=ADVANCED_FACE('',(#3078),#23026,.F.);
#24071=ADVANCED_FACE('',(#3079),#23027,.F.);
#24072=ADVANCED_FACE('',(#3080),#23028,.F.);
#24073=ADVANCED_FACE('',(#3081),#23029,.F.);
#24074=ADVANCED_FACE('',(#3082,#1293),#1809,.T.);
#24075=ADVANCED_FACE('',(#3083),#1810,.F.);
#24076=ADVANCED_FACE('',(#3084,#1294),#1811,.T.);
#24077=ADVANCED_FACE('',(#3085),#1812,.F.);
#24078=ADVANCED_FACE('',(#3086),#1813,.F.);
#24079=ADVANCED_FACE('',(#3087),#1814,.F.);
#24080=ADVANCED_FACE('',(#3088),#1815,.F.);
#24081=ADVANCED_FACE('',(#3089),#1816,.F.);
#24082=ADVANCED_FACE('',(#3090),#1817,.F.);
#24083=ADVANCED_FACE('',(#3091),#1818,.F.);
#24084=ADVANCED_FACE('',(#3092),#1819,.F.);
#24085=ADVANCED_FACE('',(#3093),#1820,.F.);
#24086=ADVANCED_FACE('',(#3094),#1821,.F.);
#24087=ADVANCED_FACE('',(#3095),#1822,.F.);
#24088=ADVANCED_FACE('',(#3096),#1823,.F.);
#24089=ADVANCED_FACE('',(#3097),#1824,.T.);
#24090=ADVANCED_FACE('',(#3098,#1295),#1825,.F.);
#24091=ADVANCED_FACE('',(#3099),#1826,.T.);
#24092=ADVANCED_FACE('',(#3100),#23030,.T.);
#24093=ADVANCED_FACE('',(#3101),#1827,.T.);
#24094=ADVANCED_FACE('',(#3102),#23031,.T.);
#24095=ADVANCED_FACE('',(#3103),#1828,.T.);
#24096=ADVANCED_FACE('',(#3104),#23032,.F.);
#24097=ADVANCED_FACE('',(#3105),#23033,.T.);
#24098=ADVANCED_FACE('',(#3106),#23034,.F.);
#24099=ADVANCED_FACE('',(#3107),#1829,.T.);
#24100=ADVANCED_FACE('',(#3108),#23035,.F.);
#24101=ADVANCED_FACE('',(#3109),#1830,.T.);
#24102=ADVANCED_FACE('',(#3110),#23036,.F.);
#24103=ADVANCED_FACE('',(#3111),#1831,.T.);
#24104=ADVANCED_FACE('',(#3112),#23037,.F.);
#24105=ADVANCED_FACE('',(#3113),#23038,.T.);
#24106=ADVANCED_FACE('',(#3114),#23039,.F.);
#24107=ADVANCED_FACE('',(#3115),#1832,.T.);
#24108=ADVANCED_FACE('',(#3116),#1833,.T.);
#24109=ADVANCED_FACE('',(#3117),#1834,.T.);
#24110=ADVANCED_FACE('',(#3118),#23040,.F.);
#24111=ADVANCED_FACE('',(#3119),#23041,.T.);
#24112=ADVANCED_FACE('',(#3120),#23042,.F.);
#24113=ADVANCED_FACE('',(#3121),#1835,.T.);
#24114=ADVANCED_FACE('',(#3122),#23043,.F.);
#24115=ADVANCED_FACE('',(#3123),#1836,.T.);
#24116=ADVANCED_FACE('',(#3124),#23044,.F.);
#24117=ADVANCED_FACE('',(#3125),#1837,.T.);
#24118=ADVANCED_FACE('',(#3126),#23045,.F.);
#24119=ADVANCED_FACE('',(#3127),#23046,.T.);
#24120=ADVANCED_FACE('',(#3128),#23047,.F.);
#24121=ADVANCED_FACE('',(#3129),#1838,.T.);
#24122=ADVANCED_FACE('',(#3130),#23048,.T.);
#24123=ADVANCED_FACE('',(#3131),#1839,.T.);
#24124=ADVANCED_FACE('',(#3132),#23049,.T.);
#24125=ADVANCED_FACE('',(#3133),#1840,.T.);
#24126=ADVANCED_FACE('',(#3134),#1841,.T.);
#24127=ADVANCED_FACE('',(#3135),#1842,.T.);
#24128=ADVANCED_FACE('',(#3136),#1843,.T.);
#24129=ADVANCED_FACE('',(#3137),#1844,.T.);
#24130=ADVANCED_FACE('',(#3138),#1845,.T.);
#24131=ADVANCED_FACE('',(#3139),#1846,.T.);
#24132=ADVANCED_FACE('',(#3140),#1847,.T.);
#24133=ADVANCED_FACE('',(#3141),#1848,.T.);
#24134=ADVANCED_FACE('',(#3142),#1849,.T.);
#24135=ADVANCED_FACE('',(#3143),#1850,.T.);
#24136=ADVANCED_FACE('',(#3144),#1851,.T.);
#24137=ADVANCED_FACE('',(#3145),#1852,.F.);
#24138=ADVANCED_FACE('',(#3146),#1853,.F.);
#24139=ADVANCED_FACE('',(#3147),#1854,.F.);
#24140=ADVANCED_FACE('',(#3148),#23050,.F.);
#24141=ADVANCED_FACE('',(#3149),#1855,.T.);
#24142=ADVANCED_FACE('',(#3150),#1856,.T.);
#24143=ADVANCED_FACE('',(#3151),#1857,.T.);
#24144=ADVANCED_FACE('',(#3152),#1858,.F.);
#24145=ADVANCED_FACE('',(#3153),#1859,.F.);
#24146=ADVANCED_FACE('',(#3154),#1860,.F.);
#24147=ADVANCED_FACE('',(#3155),#1861,.F.);
#24148=ADVANCED_FACE('',(#3156),#1862,.F.);
#24149=ADVANCED_FACE('',(#3157),#1863,.F.);
#24150=ADVANCED_FACE('',(#3158),#1864,.F.);
#24151=ADVANCED_FACE('',(#3159),#1865,.T.);
#24152=ADVANCED_FACE('',(#3160),#1866,.T.);
#24153=ADVANCED_FACE('',(#3161),#23051,.T.);
#24154=ADVANCED_FACE('',(#3162),#1867,.T.);
#24155=ADVANCED_FACE('',(#3163),#23052,.T.);
#24156=ADVANCED_FACE('',(#3164),#1868,.T.);
#24157=ADVANCED_FACE('',(#3165),#23053,.F.);
#24158=ADVANCED_FACE('',(#3166),#23054,.T.);
#24159=ADVANCED_FACE('',(#3167),#23055,.F.);
#24160=ADVANCED_FACE('',(#3168),#1869,.T.);
#24161=ADVANCED_FACE('',(#3169),#23056,.F.);
#24162=ADVANCED_FACE('',(#3170),#1870,.T.);
#24163=ADVANCED_FACE('',(#3171),#23057,.F.);
#24164=ADVANCED_FACE('',(#3172),#1871,.T.);
#24165=ADVANCED_FACE('',(#3173),#23058,.F.);
#24166=ADVANCED_FACE('',(#3174),#23059,.T.);
#24167=ADVANCED_FACE('',(#3175),#23060,.F.);
#24168=ADVANCED_FACE('',(#3176),#1872,.T.);
#24169=ADVANCED_FACE('',(#3177),#1873,.T.);
#24170=ADVANCED_FACE('',(#3178),#1874,.T.);
#24171=ADVANCED_FACE('',(#3179),#23061,.F.);
#24172=ADVANCED_FACE('',(#3180),#23062,.T.);
#24173=ADVANCED_FACE('',(#3181),#23063,.F.);
#24174=ADVANCED_FACE('',(#3182),#1875,.T.);
#24175=ADVANCED_FACE('',(#3183),#23064,.F.);
#24176=ADVANCED_FACE('',(#3184),#1876,.T.);
#24177=ADVANCED_FACE('',(#3185),#23065,.F.);
#24178=ADVANCED_FACE('',(#3186),#1877,.T.);
#24179=ADVANCED_FACE('',(#3187),#23066,.F.);
#24180=ADVANCED_FACE('',(#3188),#23067,.T.);
#24181=ADVANCED_FACE('',(#3189),#23068,.F.);
#24182=ADVANCED_FACE('',(#3190),#1878,.T.);
#24183=ADVANCED_FACE('',(#3191),#23069,.T.);
#24184=ADVANCED_FACE('',(#3192),#1879,.T.);
#24185=ADVANCED_FACE('',(#3193),#23070,.T.);
#24186=ADVANCED_FACE('',(#3194),#1880,.T.);
#24187=ADVANCED_FACE('',(#3195,#1296),#1881,.T.);
#24188=ADVANCED_FACE('',(#3196),#1882,.T.);
#24189=ADVANCED_FACE('',(#3197),#1883,.T.);
#24190=ADVANCED_FACE('',(#3198),#1884,.F.);
#24191=ADVANCED_FACE('',(#3199),#1885,.F.);
#24192=ADVANCED_FACE('',(#3200),#23071,.F.);
#24193=ADVANCED_FACE('',(#3201),#23072,.F.);
#24194=ADVANCED_FACE('',(#3202),#1886,.T.);
#24195=ADVANCED_FACE('',(#3203),#1887,.F.);
#24196=ADVANCED_FACE('',(#3204),#1888,.F.);
#24197=ADVANCED_FACE('',(#3205),#1889,.T.);
#24198=ADVANCED_FACE('',(#3206),#23073,.F.);
#24199=ADVANCED_FACE('',(#3207,#1297),#1890,.F.);
#24200=ADVANCED_FACE('',(#3208),#1891,.F.);
#24201=ADVANCED_FACE('',(#3209),#1892,.F.);
#24202=ADVANCED_FACE('',(#3210),#1893,.T.);
#24203=ADVANCED_FACE('',(#3211),#1894,.F.);
#24204=ADVANCED_FACE('',(#3212),#1895,.F.);
#24205=ADVANCED_FACE('',(#3213),#1896,.F.);
#24206=ADVANCED_FACE('',(#3214,#1298),#1897,.T.);
#24207=ADVANCED_FACE('',(#3215),#1898,.T.);
#24208=ADVANCED_FACE('',(#3216,#1299),#1899,.F.);
#24209=ADVANCED_FACE('',(#3217),#1900,.F.);
#24210=ADVANCED_FACE('',(#3218),#1901,.T.);
#24211=ADVANCED_FACE('',(#3219),#1902,.F.);
#24212=ADVANCED_FACE('',(#3220,#1300),#1903,.F.);
#24213=ADVANCED_FACE('',(#3221),#1904,.T.);
#24214=ADVANCED_FACE('',(#3222),#1905,.T.);
#24215=ADVANCED_FACE('',(#3223),#1906,.F.);
#24216=ADVANCED_FACE('',(#3224),#1907,.F.);
#24217=ADVANCED_FACE('',(#3225),#1908,.F.);
#24218=ADVANCED_FACE('',(#3226),#1909,.F.);
#24219=ADVANCED_FACE('',(#3227),#1910,.F.);
#24220=ADVANCED_FACE('',(#3228),#1911,.F.);
#24221=ADVANCED_FACE('',(#3229),#1912,.F.);
#24222=ADVANCED_FACE('',(#3230),#1913,.F.);
#24223=ADVANCED_FACE('',(#3231),#1914,.F.);
#24224=ADVANCED_FACE('',(#3232),#1915,.F.);
#24225=ADVANCED_FACE('',(#3233),#23074,.T.);
#24226=ADVANCED_FACE('',(#3234),#1916,.F.);
#24227=ADVANCED_FACE('',(#3235),#23075,.T.);
#24228=ADVANCED_FACE('',(#3236),#1917,.F.);
#24229=ADVANCED_FACE('',(#3237),#23076,.F.);
#24230=ADVANCED_FACE('',(#3238),#23077,.T.);
#24231=ADVANCED_FACE('',(#3239),#23078,.F.);
#24232=ADVANCED_FACE('',(#3240),#1918,.F.);
#24233=ADVANCED_FACE('',(#3241),#23079,.F.);
#24234=ADVANCED_FACE('',(#3242),#1919,.F.);
#24235=ADVANCED_FACE('',(#3243),#23080,.F.);
#24236=ADVANCED_FACE('',(#3244),#1920,.F.);
#24237=ADVANCED_FACE('',(#3245),#23081,.F.);
#24238=ADVANCED_FACE('',(#3246),#23082,.T.);
#24239=ADVANCED_FACE('',(#3247),#23083,.F.);
#24240=ADVANCED_FACE('',(#3248),#1921,.F.);
#24241=ADVANCED_FACE('',(#3249),#1922,.F.);
#24242=ADVANCED_FACE('',(#3250),#1923,.F.);
#24243=ADVANCED_FACE('',(#3251),#23084,.F.);
#24244=ADVANCED_FACE('',(#3252),#23085,.T.);
#24245=ADVANCED_FACE('',(#3253),#23086,.F.);
#24246=ADVANCED_FACE('',(#3254),#1924,.F.);
#24247=ADVANCED_FACE('',(#3255),#23087,.F.);
#24248=ADVANCED_FACE('',(#3256),#1925,.F.);
#24249=ADVANCED_FACE('',(#3257),#23088,.F.);
#24250=ADVANCED_FACE('',(#3258),#1926,.F.);
#24251=ADVANCED_FACE('',(#3259),#23089,.F.);
#24252=ADVANCED_FACE('',(#3260),#23090,.T.);
#24253=ADVANCED_FACE('',(#3261),#23091,.F.);
#24254=ADVANCED_FACE('',(#3262),#1927,.F.);
#24255=ADVANCED_FACE('',(#3263),#23092,.T.);
#24256=ADVANCED_FACE('',(#3264),#1928,.F.);
#24257=ADVANCED_FACE('',(#3265),#23093,.T.);
#24258=ADVANCED_FACE('',(#3266),#1929,.F.);
#24259=ADVANCED_FACE('',(#3267,#1301),#1930,.T.);
#24260=ADVANCED_FACE('',(#3268),#1931,.T.);
#24261=ADVANCED_FACE('',(#3269),#1932,.F.);
#24262=ADVANCED_FACE('',(#3270),#1933,.F.);
#24263=ADVANCED_FACE('',(#3271,#1302),#1934,.F.);
#24264=ADVANCED_FACE('',(#3272,#1303),#1935,.F.);
#24265=ADVANCED_FACE('',(#3273),#1936,.F.);
#24266=ADVANCED_FACE('',(#3274),#1937,.F.);
#24267=ADVANCED_FACE('',(#3275),#1938,.T.);
#24268=ADVANCED_FACE('',(#3276),#1939,.T.);
#24269=ADVANCED_FACE('',(#3277),#1940,.T.);
#24270=ADVANCED_FACE('',(#3278,#1304,#1305),#1941,.T.);
#24271=ADVANCED_FACE('',(#3279),#1942,.F.);
#24272=ADVANCED_FACE('',(#3280),#1943,.F.);
#24273=ADVANCED_FACE('',(#3281),#1944,.F.);
#24274=ADVANCED_FACE('',(#3282),#1945,.T.);
#24275=ADVANCED_FACE('',(#3283),#1946,.F.);
#24276=ADVANCED_FACE('',(#3284),#1947,.F.);
#24277=ADVANCED_FACE('',(#3285),#1948,.F.);
#24278=ADVANCED_FACE('',(#3286,#1306,#1307),#1949,.T.);
#24279=ADVANCED_FACE('',(#3287),#1950,.T.);
#24280=ADVANCED_FACE('',(#3288),#1951,.T.);
#24281=ADVANCED_FACE('',(#3289),#1952,.T.);
#24282=ADVANCED_FACE('',(#3290),#1953,.T.);
#24283=ADVANCED_FACE('',(#3291,#1308),#1954,.F.);
#24284=ADVANCED_FACE('',(#3292),#1955,.F.);
#24285=ADVANCED_FACE('',(#3293),#1956,.T.);
#24286=ADVANCED_FACE('',(#3294),#1957,.T.);
#24287=ADVANCED_FACE('',(#3295),#1958,.F.);
#24288=ADVANCED_FACE('',(#3296,#1309),#1959,.F.);
#24289=ADVANCED_FACE('',(#3297),#1960,.T.);
#24290=ADVANCED_FACE('',(#3298),#1961,.F.);
#24291=ADVANCED_FACE('',(#3299),#1962,.F.);
#24292=ADVANCED_FACE('',(#3300),#1963,.T.);
#24293=ADVANCED_FACE('',(#3301),#1964,.T.);
#24294=ADVANCED_FACE('',(#3302,#1310),#1965,.F.);
#24295=ADVANCED_FACE('',(#3303),#1966,.T.);
#24296=ADVANCED_FACE('',(#3304),#1967,.T.);
#24297=ADVANCED_FACE('',(#3305),#1968,.F.);
#24298=ADVANCED_FACE('',(#3306,#1311),#1969,.F.);
#24299=ADVANCED_FACE('',(#3307),#1970,.F.);
#24300=ADVANCED_FACE('',(#3308),#1971,.F.);
#24301=ADVANCED_FACE('',(#3309),#23094,.T.);
#24302=ADVANCED_FACE('',(#3310),#23095,.T.);
#24303=ADVANCED_FACE('',(#3311),#1972,.T.);
#24304=ADVANCED_FACE('',(#3312),#1973,.T.);
#24305=ADVANCED_FACE('',(#3313),#1974,.T.);
#24306=ADVANCED_FACE('',(#3314),#23096,.F.);
#24307=ADVANCED_FACE('',(#3315),#23097,.F.);
#24308=ADVANCED_FACE('',(#3316),#23098,.T.);
#24309=ADVANCED_FACE('',(#3317),#23099,.F.);
#24310=ADVANCED_FACE('',(#3318),#23100,.F.);
#24311=ADVANCED_FACE('',(#3319),#1975,.T.);
#24312=ADVANCED_FACE('',(#3320),#1976,.T.);
#24313=ADVANCED_FACE('',(#3321),#23101,.F.);
#24314=ADVANCED_FACE('',(#3322),#23102,.F.);
#24315=ADVANCED_FACE('',(#3323),#23103,.T.);
#24316=ADVANCED_FACE('',(#3324),#1977,.T.);
#24317=ADVANCED_FACE('',(#3325),#1978,.T.);
#24318=ADVANCED_FACE('',(#3326),#23104,.F.);
#24319=ADVANCED_FACE('',(#3327),#23105,.F.);
#24320=ADVANCED_FACE('',(#3328),#23106,.T.);
#24321=ADVANCED_FACE('',(#3329),#23107,.F.);
#24322=ADVANCED_FACE('',(#3330),#23108,.F.);
#24323=ADVANCED_FACE('',(#3331),#1979,.T.);
#24324=ADVANCED_FACE('',(#3332),#1980,.T.);
#24325=ADVANCED_FACE('',(#3333),#1981,.T.);
#24326=ADVANCED_FACE('',(#3334),#23109,.F.);
#24327=ADVANCED_FACE('',(#3335),#23110,.F.);
#24328=ADVANCED_FACE('',(#3336),#23111,.T.);
#24329=ADVANCED_FACE('',(#3337),#23112,.T.);
#24330=ADVANCED_FACE('',(#3338),#23113,.T.);
#24331=ADVANCED_FACE('',(#3339),#1982,.F.);
#24332=ADVANCED_FACE('',(#3340,#1312),#1983,.F.);
#24333=ADVANCED_FACE('',(#3341),#1984,.F.);
#24334=ADVANCED_FACE('',(#3342),#1985,.F.);
#24335=ADVANCED_FACE('',(#3343),#1986,.T.);
#24336=ADVANCED_FACE('',(#3344),#1987,.T.);
#24337=ADVANCED_FACE('',(#3345),#1988,.T.);
#24338=ADVANCED_FACE('',(#3346),#1989,.T.);
#24339=ADVANCED_FACE('',(#3347),#1990,.T.);
#24340=ADVANCED_FACE('',(#3348),#1991,.T.);
#24341=ADVANCED_FACE('',(#3349),#1992,.T.);
#24342=ADVANCED_FACE('',(#3350),#1993,.T.);
#24343=ADVANCED_FACE('',(#3351,#1313),#1994,.T.);
#24344=ADVANCED_FACE('',(#3352,#1314),#1995,.F.);
#24345=ADVANCED_FACE('',(#3353),#1996,.F.);
#24346=ADVANCED_FACE('',(#3354),#23114,.F.);
#24347=ADVANCED_FACE('',(#3355),#1997,.F.);
#24348=ADVANCED_FACE('',(#3356),#1998,.T.);
#24349=ADVANCED_FACE('',(#3357),#23115,.F.);
#24350=ADVANCED_FACE('',(#3358),#23116,.F.);
#24351=ADVANCED_FACE('',(#3359),#23117,.F.);
#24352=ADVANCED_FACE('',(#3360),#23118,.F.);
#24551=CLOSED_SHELL('',(#24014,#24015,#24016,#24017,#24018,#24019,#24020,
#24021,#24022,#24023,#24024,#24025,#24026,#24027,#24028,#24029,#24030,#24031,
#24032,#24033,#24034,#24035,#24036,#24037,#24038,#24039,#24040,#24041,#24042,
#24043,#24044,#24045,#24046,#24047,#24048,#24049,#24050,#24051,#24052,#24053,
#24054,#24055,#24056,#24057,#24058,#24059,#24060,#24061,#24062,#24063,#24064,
#24065,#24066,#24067,#24068,#24069,#24070,#24071,#24072,#24073,#24074,#24075,
#24076,#24077,#24078,#24079,#24080,#24081,#24082,#24083,#24084,#24085,#24086,
#24087,#24088,#24089,#24090,#24091,#24092,#24093,#24094,#24095,#24096,#24097,
#24098,#24099,#24100,#24101,#24102,#24103,#24104,#24105,#24106,#24107,#24108,
#24109,#24110,#24111,#24112,#24113,#24114,#24115,#24116,#24117,#24118,#24119,
#24120,#24121,#24122,#24123,#24124,#24125,#24126,#24127,#24128,#24129,#24130,
#24131,#24132,#24133,#24134,#24135,#24136,#24137,#24138,#24139,#24140,#24141,
#24142,#24143,#24144,#24145,#24146,#24147,#24148,#24149,#24150,#24151,#24152,
#24153,#24154,#24155,#24156,#24157,#24158,#24159,#24160,#24161,#24162,#24163,
#24164,#24165,#24166,#24167,#24168,#24169,#24170,#24171,#24172,#24173,#24174,
#24175,#24176,#24177,#24178,#24179,#24180,#24181,#24182,#24183,#24184,#24185,
#24186,#24187,#24188,#24189,#24190,#24191,#24192,#24193,#24194,#24195,#24196,
#24197,#24198,#24199,#24200,#24201,#24202,#24203,#24204,#24205,#24206,#24207,
#24208,#24209,#24210,#24211,#24212,#24213,#24214,#24215,#24216,#24217,#24218,
#24219,#24220,#24221,#24222,#24223,#24224,#24225,#24226,#24227,#24228,#24229,
#24230,#24231,#24232,#24233,#24234,#24235,#24236,#24237,#24238,#24239,#24240,
#24241,#24242,#24243,#24244,#24245,#24246,#24247,#24248,#24249,#24250,#24251,
#24252,#24253,#24254,#24255,#24256,#24257,#24258,#24259,#24260,#24261,#24262,
#24263,#24264,#24265,#24266,#24267,#24268,#24269,#24270,#24271,#24272,#24273,
#24274,#24275,#24276,#24277,#24278,#24279,#24280,#24281,#24282,#24283,#24284,
#24285,#24286,#24287,#24288,#24289,#24290,#24291,#24292,#24293,#24294,#24295,
#24296,#24297,#24298,#24299,#24300,#24301,#24302,#24303,#24304,#24305,#24306,
#24307,#24308,#24309,#24310,#24311,#24312,#24313,#24314,#24315,#24316,#24317,
#24318,#24319,#24320,#24321,#24322,#24323,#24324,#24325,#24326,#24327,#24328,
#24329,#24330,#24331,#24332,#24333,#24334,#24335,#24336,#24337,#24338,#24339,
#24340,#24341,#24342,#24343,#24344,#24345,#24346,#24347,#24348,#24349,#24350,
#24351,#24352));
#26507=AXIS2_PLACEMENT_3D('',#54036,#31779,#31780);
#26508=AXIS2_PLACEMENT_3D('',#54037,#31781,#31782);
#26509=AXIS2_PLACEMENT_3D('',#54039,#31783,#31784);
#26510=AXIS2_PLACEMENT_3D('',#54042,#31786,#31787);
#26511=AXIS2_PLACEMENT_3D('',#54043,#31788,#31789);
#26512=AXIS2_PLACEMENT_3D('',#54045,#31790,#31791);
#26513=AXIS2_PLACEMENT_3D('',#54048,#31793,#31794);
#26514=AXIS2_PLACEMENT_3D('',#54049,#31795,#31796);
#26515=AXIS2_PLACEMENT_3D('',#54051,#31797,#31798);
#26516=AXIS2_PLACEMENT_3D('',#54054,#31800,#31801);
#26517=AXIS2_PLACEMENT_3D('',#54055,#31802,#31803);
#26518=AXIS2_PLACEMENT_3D('',#54058,#31805,#31806);
#26519=AXIS2_PLACEMENT_3D('',#54061,#31808,#31809);
#26520=AXIS2_PLACEMENT_3D('',#54063,#31810,#31811);
#26521=AXIS2_PLACEMENT_3D('',#54066,#31813,#31814);
#26522=AXIS2_PLACEMENT_3D('',#54067,#31815,#31816);
#26523=AXIS2_PLACEMENT_3D('',#54069,#31817,#31818);
#26524=AXIS2_PLACEMENT_3D('',#54072,#31820,#31821);
#26525=AXIS2_PLACEMENT_3D('',#54073,#31822,#31823);
#26526=AXIS2_PLACEMENT_3D('',#54075,#31824,#31825);
#26527=AXIS2_PLACEMENT_3D('',#54078,#31827,#31828);
#26528=AXIS2_PLACEMENT_3D('',#54079,#31829,#31830);
#26529=AXIS2_PLACEMENT_3D('',#54081,#31831,#31832);
#26530=AXIS2_PLACEMENT_3D('',#54084,#31834,#31835);
#26531=AXIS2_PLACEMENT_3D('',#54085,#31836,#31837);
#26532=AXIS2_PLACEMENT_3D('',#54087,#31838,#31839);
#26533=AXIS2_PLACEMENT_3D('',#54090,#31841,#31842);
#26534=AXIS2_PLACEMENT_3D('',#54091,#31843,#31844);
#26535=AXIS2_PLACEMENT_3D('',#54093,#31845,#31846);
#26536=AXIS2_PLACEMENT_3D('',#54096,#31848,#31849);
#26537=AXIS2_PLACEMENT_3D('',#54097,#31850,#31851);
#26538=AXIS2_PLACEMENT_3D('',#54099,#31852,#31853);
#26539=AXIS2_PLACEMENT_3D('',#54102,#31855,#31856);
#26540=AXIS2_PLACEMENT_3D('',#54103,#31857,#31858);
#26541=AXIS2_PLACEMENT_3D('',#54105,#31859,#31860);
#26542=AXIS2_PLACEMENT_3D('',#54109,#31862,#31863);
#26543=AXIS2_PLACEMENT_3D('',#54113,#31865,#31866);
#26544=AXIS2_PLACEMENT_3D('',#54115,#31868,#31869);
#26545=AXIS2_PLACEMENT_3D('',#54118,#31871,#31872);
#26546=AXIS2_PLACEMENT_3D('',#54121,#31874,#31875);
#26547=AXIS2_PLACEMENT_3D('',#54123,#31876,#31877);
#26548=AXIS2_PLACEMENT_3D('',#54129,#31880,#31881);
#26549=AXIS2_PLACEMENT_3D('',#54132,#31883,#31884);
#26550=AXIS2_PLACEMENT_3D('',#54199,#31885,#31886);
#26551=AXIS2_PLACEMENT_3D('',#54200,#31887,#31888);
#26552=AXIS2_PLACEMENT_3D('',#54233,#31889,#31890);
#26553=AXIS2_PLACEMENT_3D('',#54235,#31891,#31892);
#26554=AXIS2_PLACEMENT_3D('',#54237,#31894,#31895);
#26555=AXIS2_PLACEMENT_3D('',#54239,#31896,#31897);
#26556=AXIS2_PLACEMENT_3D('',#54242,#31899,#31900);
#26557=AXIS2_PLACEMENT_3D('',#54243,#31901,#31902);
#26558=AXIS2_PLACEMENT_3D('',#54246,#31903,#31904);
#26559=AXIS2_PLACEMENT_3D('',#54252,#31908,#31909);
#26560=AXIS2_PLACEMENT_3D('',#54254,#31910,#31911);
#26561=AXIS2_PLACEMENT_3D('',#54258,#31913,#31914);
#26562=AXIS2_PLACEMENT_3D('',#54260,#31916,#31917);
#26563=AXIS2_PLACEMENT_3D('',#54263,#31918,#31919);
#26564=AXIS2_PLACEMENT_3D('',#54267,#31921,#31922);
#26565=AXIS2_PLACEMENT_3D('',#54269,#31924,#31925);
#26566=AXIS2_PLACEMENT_3D('',#54271,#31926,#31927);
#26567=AXIS2_PLACEMENT_3D('',#54277,#31931,#31932);
#26568=AXIS2_PLACEMENT_3D('',#54286,#31937,#31938);
#26569=AXIS2_PLACEMENT_3D('',#54295,#31943,#31944);
#26570=AXIS2_PLACEMENT_3D('',#54304,#31949,#31950);
#26571=AXIS2_PLACEMENT_3D('',#54313,#31955,#31956);
#26572=AXIS2_PLACEMENT_3D('',#54322,#31961,#31962);
#26573=AXIS2_PLACEMENT_3D('',#54331,#31967,#31968);
#26574=AXIS2_PLACEMENT_3D('',#54340,#31973,#31974);
#26575=AXIS2_PLACEMENT_3D('',#54349,#31979,#31980);
#26576=AXIS2_PLACEMENT_3D('',#54358,#31985,#31986);
#26577=AXIS2_PLACEMENT_3D('',#54364,#31990,#31991);
#26578=AXIS2_PLACEMENT_3D('',#54373,#31996,#31997);
#26579=AXIS2_PLACEMENT_3D('',#54379,#32001,#32002);
#26580=AXIS2_PLACEMENT_3D('',#54388,#32007,#32008);
#26581=AXIS2_PLACEMENT_3D('',#54397,#32013,#32014);
#26582=AXIS2_PLACEMENT_3D('',#54406,#32019,#32020);
#26583=AXIS2_PLACEMENT_3D('',#54415,#32025,#32026);
#26584=AXIS2_PLACEMENT_3D('',#54418,#32029,#32030);
#26585=AXIS2_PLACEMENT_3D('',#54421,#32031,#32032);
#26586=AXIS2_PLACEMENT_3D('',#54425,#32034,#32035);
#26587=AXIS2_PLACEMENT_3D('',#54427,#32037,#32038);
#26588=AXIS2_PLACEMENT_3D('',#54430,#32039,#32040);
#26589=AXIS2_PLACEMENT_3D('',#54434,#32042,#32043);
#26590=AXIS2_PLACEMENT_3D('',#54436,#32045,#32046);
#26591=AXIS2_PLACEMENT_3D('',#54439,#32047,#32048);
#26592=AXIS2_PLACEMENT_3D('',#54443,#32050,#32051);
#26593=AXIS2_PLACEMENT_3D('',#54445,#32053,#32054);
#26594=AXIS2_PLACEMENT_3D('',#54448,#32055,#32056);
#26595=AXIS2_PLACEMENT_3D('',#54452,#32058,#32059);
#26596=AXIS2_PLACEMENT_3D('',#54454,#32061,#32062);
#26597=AXIS2_PLACEMENT_3D('',#54455,#32063,#32064);
#26598=AXIS2_PLACEMENT_3D('',#54456,#32065,#32066);
#26599=AXIS2_PLACEMENT_3D('',#54457,#32067,#32068);
#26600=AXIS2_PLACEMENT_3D('',#54458,#32069,#32070);
#26601=AXIS2_PLACEMENT_3D('',#54459,#32071,#32072);
#26602=AXIS2_PLACEMENT_3D('',#54460,#32073,#32074);
#26603=AXIS2_PLACEMENT_3D('',#54461,#32075,#32076);
#26604=AXIS2_PLACEMENT_3D('',#54462,#32077,#32078);
#26605=AXIS2_PLACEMENT_3D('',#54463,#32079,#32080);
#26606=AXIS2_PLACEMENT_3D('',#54464,#32081,#32082);
#26607=AXIS2_PLACEMENT_3D('',#54465,#32083,#32084);
#26608=AXIS2_PLACEMENT_3D('',#54466,#32085,#32086);
#26609=AXIS2_PLACEMENT_3D('',#54467,#32087,#32088);
#26610=AXIS2_PLACEMENT_3D('',#54468,#32089,#32090);
#26611=AXIS2_PLACEMENT_3D('',#54469,#32091,#32092);
#26612=AXIS2_PLACEMENT_3D('',#54470,#32093,#32094);
#26613=AXIS2_PLACEMENT_3D('',#54471,#32095,#32096);
#26614=AXIS2_PLACEMENT_3D('',#54472,#32097,#32098);
#26615=AXIS2_PLACEMENT_3D('',#54473,#32099,#32100);
#26616=AXIS2_PLACEMENT_3D('',#54474,#32101,#32102);
#26617=AXIS2_PLACEMENT_3D('',#54475,#32103,#32104);
#26618=AXIS2_PLACEMENT_3D('',#54476,#32105,#32106);
#26619=AXIS2_PLACEMENT_3D('',#54477,#32107,#32108);
#26620=AXIS2_PLACEMENT_3D('',#54478,#32109,#32110);
#26621=AXIS2_PLACEMENT_3D('',#54479,#32111,#32112);
#26622=AXIS2_PLACEMENT_3D('',#54480,#32113,#32114);
#26623=AXIS2_PLACEMENT_3D('',#54481,#32115,#32116);
#26624=AXIS2_PLACEMENT_3D('',#54482,#32117,#32118);
#26625=AXIS2_PLACEMENT_3D('',#54483,#32119,#32120);
#26626=AXIS2_PLACEMENT_3D('',#54484,#32121,#32122);
#26627=AXIS2_PLACEMENT_3D('',#54485,#32123,#32124);
#26628=AXIS2_PLACEMENT_3D('',#54486,#32125,#32126);
#26629=AXIS2_PLACEMENT_3D('',#54487,#32127,#32128);
#26630=AXIS2_PLACEMENT_3D('',#54488,#32129,#32130);
#26631=AXIS2_PLACEMENT_3D('',#54489,#32131,#32132);
#26632=AXIS2_PLACEMENT_3D('',#54490,#32133,#32134);
#26633=AXIS2_PLACEMENT_3D('',#54491,#32135,#32136);
#26634=AXIS2_PLACEMENT_3D('',#54492,#32137,#32138);
#26635=AXIS2_PLACEMENT_3D('',#54493,#32139,#32140);
#26636=AXIS2_PLACEMENT_3D('',#54494,#32141,#32142);
#26637=AXIS2_PLACEMENT_3D('',#54495,#32143,#32144);
#26638=AXIS2_PLACEMENT_3D('',#54496,#32145,#32146);
#26639=AXIS2_PLACEMENT_3D('',#54497,#32147,#32148);
#26640=AXIS2_PLACEMENT_3D('',#54498,#32149,#32150);
#26641=AXIS2_PLACEMENT_3D('',#54499,#32151,#32152);
#26642=AXIS2_PLACEMENT_3D('',#54500,#32153,#32154);
#26643=AXIS2_PLACEMENT_3D('',#54501,#32155,#32156);
#26644=AXIS2_PLACEMENT_3D('',#54502,#32157,#32158);
#26645=AXIS2_PLACEMENT_3D('',#54503,#32159,#32160);
#26646=AXIS2_PLACEMENT_3D('',#54512,#32165,#32166);
#26647=AXIS2_PLACEMENT_3D('',#54523,#32173,#32174);
#26648=AXIS2_PLACEMENT_3D('',#54527,#32177,#32178);
#26649=AXIS2_PLACEMENT_3D('',#54531,#32181,#32182);
#26650=AXIS2_PLACEMENT_3D('',#54533,#32184,#32185);
#26651=AXIS2_PLACEMENT_3D('',#54537,#32188,#32189);
#26652=AXIS2_PLACEMENT_3D('',#54541,#32192,#32193);
#26653=AXIS2_PLACEMENT_3D('',#54543,#32195,#32196);
#26654=AXIS2_PLACEMENT_3D('',#54549,#32200,#32201);
#26655=AXIS2_PLACEMENT_3D('',#54553,#32204,#32205);
#26656=AXIS2_PLACEMENT_3D('',#54557,#32208,#32209);
#26657=AXIS2_PLACEMENT_3D('',#54561,#32212,#32213);
#26658=AXIS2_PLACEMENT_3D('',#54565,#32216,#32217);
#26659=AXIS2_PLACEMENT_3D('',#54567,#32219,#32220);
#26660=AXIS2_PLACEMENT_3D('',#54568,#32221,#32222);
#26661=AXIS2_PLACEMENT_3D('',#54573,#32224,#32225);
#26662=AXIS2_PLACEMENT_3D('',#54577,#32227,#32228);
#26663=AXIS2_PLACEMENT_3D('',#54581,#32230,#32231);
#26664=AXIS2_PLACEMENT_3D('',#54583,#32232,#32233);
#26665=AXIS2_PLACEMENT_3D('',#54585,#32234,#32235);
#26666=AXIS2_PLACEMENT_3D('',#54589,#32237,#32238);
#26667=AXIS2_PLACEMENT_3D('',#54593,#32240,#32241);
#26668=AXIS2_PLACEMENT_3D('',#54597,#32243,#32244);
#26669=AXIS2_PLACEMENT_3D('',#54599,#32245,#32246);
#26670=AXIS2_PLACEMENT_3D('',#54601,#32247,#32248);
#26671=AXIS2_PLACEMENT_3D('',#54609,#32252,#32253);
#26672=AXIS2_PLACEMENT_3D('',#54611,#32254,#32255);
#26673=AXIS2_PLACEMENT_3D('',#54613,#32256,#32257);
#26674=AXIS2_PLACEMENT_3D('',#54617,#32259,#32260);
#26675=AXIS2_PLACEMENT_3D('',#54621,#32262,#32263);
#26676=AXIS2_PLACEMENT_3D('',#54625,#32265,#32266);
#26677=AXIS2_PLACEMENT_3D('',#54627,#32267,#32268);
#26678=AXIS2_PLACEMENT_3D('',#54629,#32269,#32270);
#26679=AXIS2_PLACEMENT_3D('',#54633,#32272,#32273);
#26680=AXIS2_PLACEMENT_3D('',#54637,#32275,#32276);
#26681=AXIS2_PLACEMENT_3D('',#54657,#32287,#32288);
#26682=AXIS2_PLACEMENT_3D('',#54663,#32292,#32293);
#26683=AXIS2_PLACEMENT_3D('',#54665,#32294,#32295);
#26684=AXIS2_PLACEMENT_3D('',#54667,#32297,#32298);
#26685=AXIS2_PLACEMENT_3D('',#54671,#32301,#32302);
#26686=AXIS2_PLACEMENT_3D('',#54673,#32303,#32304);
#26687=AXIS2_PLACEMENT_3D('',#54675,#32306,#32307);
#26688=AXIS2_PLACEMENT_3D('',#54679,#32310,#32311);
#26689=AXIS2_PLACEMENT_3D('',#54681,#32312,#32313);
#26690=AXIS2_PLACEMENT_3D('',#54683,#32315,#32316);
#26691=AXIS2_PLACEMENT_3D('',#54685,#32317,#32318);
#26692=AXIS2_PLACEMENT_3D('',#54687,#32320,#32321);
#26693=AXIS2_PLACEMENT_3D('',#54689,#32322,#32323);
#26694=AXIS2_PLACEMENT_3D('',#54691,#32325,#32326);
#26695=AXIS2_PLACEMENT_3D('',#54695,#32329,#32330);
#26696=AXIS2_PLACEMENT_3D('',#54697,#32331,#32332);
#26697=AXIS2_PLACEMENT_3D('',#54699,#32334,#32335);
#26698=AXIS2_PLACEMENT_3D('',#54703,#32338,#32339);
#26699=AXIS2_PLACEMENT_3D('',#54705,#32340,#32341);
#26700=AXIS2_PLACEMENT_3D('',#54707,#32343,#32344);
#26701=AXIS2_PLACEMENT_3D('',#54711,#32347,#32348);
#26702=AXIS2_PLACEMENT_3D('',#54713,#32349,#32350);
#26703=AXIS2_PLACEMENT_3D('',#54715,#32352,#32353);
#26704=AXIS2_PLACEMENT_3D('',#54717,#32354,#32355);
#26705=AXIS2_PLACEMENT_3D('',#54719,#32357,#32358);
#26706=AXIS2_PLACEMENT_3D('',#54721,#32359,#32360);
#26707=AXIS2_PLACEMENT_3D('',#54723,#32362,#32363);
#26708=AXIS2_PLACEMENT_3D('',#54727,#32366,#32367);
#26709=AXIS2_PLACEMENT_3D('',#54731,#32370,#32371);
#26710=AXIS2_PLACEMENT_3D('',#54735,#32374,#32375);
#26711=AXIS2_PLACEMENT_3D('',#54737,#32376,#32377);
#26712=AXIS2_PLACEMENT_3D('',#54739,#32379,#32380);
#26713=AXIS2_PLACEMENT_3D('',#54741,#32381,#32382);
#26714=AXIS2_PLACEMENT_3D('',#54743,#32384,#32385);
#26715=AXIS2_PLACEMENT_3D('',#54745,#32386,#32387);
#26716=AXIS2_PLACEMENT_3D('',#54747,#32389,#32390);
#26717=AXIS2_PLACEMENT_3D('',#54751,#32393,#32394);
#26718=AXIS2_PLACEMENT_3D('',#54753,#32395,#32396);
#26719=AXIS2_PLACEMENT_3D('',#54755,#32398,#32399);
#26720=AXIS2_PLACEMENT_3D('',#54759,#32402,#32403);
#26721=AXIS2_PLACEMENT_3D('',#54761,#32404,#32405);
#26722=AXIS2_PLACEMENT_3D('',#54763,#32407,#32408);
#26723=AXIS2_PLACEMENT_3D('',#54767,#32411,#32412);
#26724=AXIS2_PLACEMENT_3D('',#54769,#32413,#32414);
#26725=AXIS2_PLACEMENT_3D('',#54771,#32416,#32417);
#26726=AXIS2_PLACEMENT_3D('',#54773,#32418,#32419);
#26727=AXIS2_PLACEMENT_3D('',#54775,#32421,#32422);
#26728=AXIS2_PLACEMENT_3D('',#54777,#32423,#32424);
#26729=AXIS2_PLACEMENT_3D('',#54779,#32426,#32427);
#26730=AXIS2_PLACEMENT_3D('',#54783,#32430,#32431);
#26731=AXIS2_PLACEMENT_3D('',#54785,#32432,#32433);
#26732=AXIS2_PLACEMENT_3D('',#54787,#32435,#32436);
#26733=AXIS2_PLACEMENT_3D('',#54791,#32439,#32440);
#26734=AXIS2_PLACEMENT_3D('',#54793,#32441,#32442);
#26735=AXIS2_PLACEMENT_3D('',#54795,#32444,#32445);
#26736=AXIS2_PLACEMENT_3D('',#54799,#32448,#32449);
#26737=AXIS2_PLACEMENT_3D('',#54803,#32452,#32453);
#26738=AXIS2_PLACEMENT_3D('',#54807,#32456,#32457);
#26739=AXIS2_PLACEMENT_3D('',#54811,#32460,#32461);
#26740=AXIS2_PLACEMENT_3D('',#54815,#32464,#32465);
#26741=AXIS2_PLACEMENT_3D('',#54819,#32468,#32469);
#26742=AXIS2_PLACEMENT_3D('',#54823,#32472,#32473);
#26743=AXIS2_PLACEMENT_3D('',#54827,#32476,#32477);
#26744=AXIS2_PLACEMENT_3D('',#54831,#32480,#32481);
#26745=AXIS2_PLACEMENT_3D('',#54833,#32483,#32484);
#26746=AXIS2_PLACEMENT_3D('',#54834,#32485,#32486);
#26747=AXIS2_PLACEMENT_3D('',#54838,#32488,#32489);
#26748=AXIS2_PLACEMENT_3D('',#54840,#32491,#32492);
#26749=AXIS2_PLACEMENT_3D('',#54847,#32495,#32496);
#26750=AXIS2_PLACEMENT_3D('',#54863,#32504,#32505);
#26751=AXIS2_PLACEMENT_3D('',#54867,#32507,#32508);
#26752=AXIS2_PLACEMENT_3D('',#54871,#32510,#32511);
#26753=AXIS2_PLACEMENT_3D('',#54873,#32512,#32513);
#26754=AXIS2_PLACEMENT_3D('',#54875,#32514,#32515);
#26755=AXIS2_PLACEMENT_3D('',#54879,#32517,#32518);
#26756=AXIS2_PLACEMENT_3D('',#54883,#32520,#32521);
#26757=AXIS2_PLACEMENT_3D('',#54887,#32523,#32524);
#26758=AXIS2_PLACEMENT_3D('',#54889,#32525,#32526);
#26759=AXIS2_PLACEMENT_3D('',#54891,#32527,#32528);
#26760=AXIS2_PLACEMENT_3D('',#54899,#32532,#32533);
#26761=AXIS2_PLACEMENT_3D('',#54901,#32534,#32535);
#26762=AXIS2_PLACEMENT_3D('',#54903,#32536,#32537);
#26763=AXIS2_PLACEMENT_3D('',#54907,#32539,#32540);
#26764=AXIS2_PLACEMENT_3D('',#54911,#32542,#32543);
#26765=AXIS2_PLACEMENT_3D('',#54915,#32545,#32546);
#26766=AXIS2_PLACEMENT_3D('',#54917,#32547,#32548);
#26767=AXIS2_PLACEMENT_3D('',#54919,#32549,#32550);
#26768=AXIS2_PLACEMENT_3D('',#54923,#32552,#32553);
#26769=AXIS2_PLACEMENT_3D('',#54927,#32555,#32556);
#26770=AXIS2_PLACEMENT_3D('',#54937,#32562,#32563);
#26771=AXIS2_PLACEMENT_3D('',#54941,#32566,#32567);
#26772=AXIS2_PLACEMENT_3D('',#54945,#32570,#32571);
#26773=AXIS2_PLACEMENT_3D('',#54946,#32572,#32573);
#26774=AXIS2_PLACEMENT_3D('',#54947,#32574,#32575);
#26775=AXIS2_PLACEMENT_3D('',#54948,#32576,#32577);
#26776=AXIS2_PLACEMENT_3D('',#54952,#32579,#32580);
#26777=AXIS2_PLACEMENT_3D('',#54954,#32582,#32583);
#26778=AXIS2_PLACEMENT_3D('',#54960,#32587,#32588);
#26779=AXIS2_PLACEMENT_3D('',#54964,#32591,#32592);
#26780=AXIS2_PLACEMENT_3D('',#54968,#32595,#32596);
#26781=AXIS2_PLACEMENT_3D('',#54972,#32599,#32600);
#26782=AXIS2_PLACEMENT_3D('',#54981,#32606,#32607);
#26783=AXIS2_PLACEMENT_3D('',#54985,#32610,#32611);
#26784=AXIS2_PLACEMENT_3D('',#54989,#32614,#32615);
#26785=AXIS2_PLACEMENT_3D('',#54993,#32618,#32619);
#26786=AXIS2_PLACEMENT_3D('',#54997,#32622,#32623);
#26787=AXIS2_PLACEMENT_3D('',#55001,#32626,#32627);
#26788=AXIS2_PLACEMENT_3D('',#55003,#32628,#32629);
#26789=AXIS2_PLACEMENT_3D('',#55005,#32631,#32632);
#26790=AXIS2_PLACEMENT_3D('',#55009,#32635,#32636);
#26791=AXIS2_PLACEMENT_3D('',#55011,#32637,#32638);
#26792=AXIS2_PLACEMENT_3D('',#55013,#32640,#32641);
#26793=AXIS2_PLACEMENT_3D('',#55017,#32644,#32645);
#26794=AXIS2_PLACEMENT_3D('',#55019,#32646,#32647);
#26795=AXIS2_PLACEMENT_3D('',#55021,#32649,#32650);
#26796=AXIS2_PLACEMENT_3D('',#55023,#32651,#32652);
#26797=AXIS2_PLACEMENT_3D('',#55025,#32654,#32655);
#26798=AXIS2_PLACEMENT_3D('',#55027,#32656,#32657);
#26799=AXIS2_PLACEMENT_3D('',#55029,#32659,#32660);
#26800=AXIS2_PLACEMENT_3D('',#55033,#32663,#32664);
#26801=AXIS2_PLACEMENT_3D('',#55035,#32665,#32666);
#26802=AXIS2_PLACEMENT_3D('',#55037,#32668,#32669);
#26803=AXIS2_PLACEMENT_3D('',#55041,#32672,#32673);
#26804=AXIS2_PLACEMENT_3D('',#55043,#32674,#32675);
#26805=AXIS2_PLACEMENT_3D('',#55045,#32677,#32678);
#26806=AXIS2_PLACEMENT_3D('',#55049,#32681,#32682);
#26807=AXIS2_PLACEMENT_3D('',#55051,#32683,#32684);
#26808=AXIS2_PLACEMENT_3D('',#55053,#32686,#32687);
#26809=AXIS2_PLACEMENT_3D('',#55055,#32688,#32689);
#26810=AXIS2_PLACEMENT_3D('',#55057,#32691,#32692);
#26811=AXIS2_PLACEMENT_3D('',#55059,#32693,#32694);
#26812=AXIS2_PLACEMENT_3D('',#55061,#32696,#32697);
#26813=AXIS2_PLACEMENT_3D('',#55065,#32700,#32701);
#26814=AXIS2_PLACEMENT_3D('',#55069,#32704,#32705);
#26815=AXIS2_PLACEMENT_3D('',#55073,#32708,#32709);
#26816=AXIS2_PLACEMENT_3D('',#55075,#32710,#32711);
#26817=AXIS2_PLACEMENT_3D('',#55077,#32713,#32714);
#26818=AXIS2_PLACEMENT_3D('',#55079,#32715,#32716);
#26819=AXIS2_PLACEMENT_3D('',#55081,#32718,#32719);
#26820=AXIS2_PLACEMENT_3D('',#55083,#32720,#32721);
#26821=AXIS2_PLACEMENT_3D('',#55085,#32723,#32724);
#26822=AXIS2_PLACEMENT_3D('',#55089,#32727,#32728);
#26823=AXIS2_PLACEMENT_3D('',#55091,#32729,#32730);
#26824=AXIS2_PLACEMENT_3D('',#55093,#32732,#32733);
#26825=AXIS2_PLACEMENT_3D('',#55097,#32736,#32737);
#26826=AXIS2_PLACEMENT_3D('',#55099,#32738,#32739);
#26827=AXIS2_PLACEMENT_3D('',#55101,#32741,#32742);
#26828=AXIS2_PLACEMENT_3D('',#55105,#32745,#32746);
#26829=AXIS2_PLACEMENT_3D('',#55107,#32747,#32748);
#26830=AXIS2_PLACEMENT_3D('',#55109,#32750,#32751);
#26831=AXIS2_PLACEMENT_3D('',#55111,#32752,#32753);
#26832=AXIS2_PLACEMENT_3D('',#55113,#32755,#32756);
#26833=AXIS2_PLACEMENT_3D('',#55115,#32757,#32758);
#26834=AXIS2_PLACEMENT_3D('',#55117,#32760,#32761);
#26835=AXIS2_PLACEMENT_3D('',#55121,#32764,#32765);
#26836=AXIS2_PLACEMENT_3D('',#55123,#32766,#32767);
#26837=AXIS2_PLACEMENT_3D('',#55125,#32769,#32770);
#26838=AXIS2_PLACEMENT_3D('',#55129,#32773,#32774);
#26839=AXIS2_PLACEMENT_3D('',#55131,#32775,#32776);
#26840=AXIS2_PLACEMENT_3D('',#55133,#32778,#32779);
#26841=AXIS2_PLACEMENT_3D('',#55135,#32781,#32782);
#26842=AXIS2_PLACEMENT_3D('',#55136,#32783,#32784);
#26843=AXIS2_PLACEMENT_3D('',#55145,#32789,#32790);
#26844=AXIS2_PLACEMENT_3D('',#55154,#32795,#32796);
#26845=AXIS2_PLACEMENT_3D('',#55158,#32799,#32800);
#26846=AXIS2_PLACEMENT_3D('',#55162,#32803,#32804);
#26847=AXIS2_PLACEMENT_3D('',#55163,#32805,#32806);
#26848=AXIS2_PLACEMENT_3D('',#55164,#32807,#32808);
#26849=AXIS2_PLACEMENT_3D('',#55166,#32809,#32810);
#26850=AXIS2_PLACEMENT_3D('',#55168,#32811,#32812);
#26851=AXIS2_PLACEMENT_3D('',#55170,#32814,#32815);
#26852=AXIS2_PLACEMENT_3D('',#55178,#32820,#32821);
#26853=AXIS2_PLACEMENT_3D('',#55184,#32825,#32826);
#26854=AXIS2_PLACEMENT_3D('',#55193,#32831,#32832);
#26855=AXIS2_PLACEMENT_3D('',#55196,#32834,#32835);
#26856=AXIS2_PLACEMENT_3D('',#55200,#32838,#32839);
#26857=AXIS2_PLACEMENT_3D('',#55203,#32841,#32842);
#26858=AXIS2_PLACEMENT_3D('',#55204,#32843,#32844);
#26859=AXIS2_PLACEMENT_3D('',#55227,#32855,#32856);
#26860=AXIS2_PLACEMENT_3D('',#55231,#32858,#32859);
#26861=AXIS2_PLACEMENT_3D('',#55235,#32861,#32862);
#26862=AXIS2_PLACEMENT_3D('',#55237,#32863,#32864);
#26863=AXIS2_PLACEMENT_3D('',#55239,#32865,#32866);
#26864=AXIS2_PLACEMENT_3D('',#55243,#32868,#32869);
#26865=AXIS2_PLACEMENT_3D('',#55247,#32871,#32872);
#26866=AXIS2_PLACEMENT_3D('',#55251,#32874,#32875);
#26867=AXIS2_PLACEMENT_3D('',#55253,#32876,#32877);
#26868=AXIS2_PLACEMENT_3D('',#55255,#32878,#32879);
#26869=AXIS2_PLACEMENT_3D('',#55263,#32883,#32884);
#26870=AXIS2_PLACEMENT_3D('',#55265,#32885,#32886);
#26871=AXIS2_PLACEMENT_3D('',#55267,#32887,#32888);
#26872=AXIS2_PLACEMENT_3D('',#55271,#32890,#32891);
#26873=AXIS2_PLACEMENT_3D('',#55275,#32893,#32894);
#26874=AXIS2_PLACEMENT_3D('',#55279,#32896,#32897);
#26875=AXIS2_PLACEMENT_3D('',#55281,#32898,#32899);
#26876=AXIS2_PLACEMENT_3D('',#55283,#32900,#32901);
#26877=AXIS2_PLACEMENT_3D('',#55287,#32903,#32904);
#26878=AXIS2_PLACEMENT_3D('',#55291,#32906,#32907);
#26879=AXIS2_PLACEMENT_3D('',#55293,#32909,#32910);
#26880=AXIS2_PLACEMENT_3D('',#55297,#32913,#32914);
#26881=AXIS2_PLACEMENT_3D('',#55301,#32917,#32918);
#26882=AXIS2_PLACEMENT_3D('',#55307,#32922,#32923);
#26883=AXIS2_PLACEMENT_3D('',#55313,#32927,#32928);
#26884=AXIS2_PLACEMENT_3D('',#55319,#32932,#32933);
#26885=AXIS2_PLACEMENT_3D('',#55325,#32937,#32938);
#26886=AXIS2_PLACEMENT_3D('',#55326,#32939,#32940);
#26887=AXIS2_PLACEMENT_3D('',#55327,#32941,#32942);
#26888=AXIS2_PLACEMENT_3D('',#55328,#32943,#32944);
#26889=AXIS2_PLACEMENT_3D('',#55329,#32945,#32946);
#26890=AXIS2_PLACEMENT_3D('',#55331,#32947,#32948);
#26891=AXIS2_PLACEMENT_3D('',#55337,#32952,#32953);
#26892=AXIS2_PLACEMENT_3D('',#55343,#32957,#32958);
#26893=AXIS2_PLACEMENT_3D('',#55345,#32959,#32960);
#26894=AXIS2_PLACEMENT_3D('',#55349,#32963,#32964);
#26895=AXIS2_PLACEMENT_3D('',#55355,#32968,#32969);
#26896=AXIS2_PLACEMENT_3D('',#55359,#32972,#32973);
#26897=AXIS2_PLACEMENT_3D('',#55360,#32974,#32975);
#26898=AXIS2_PLACEMENT_3D('',#55362,#32976,#32977);
#26899=AXIS2_PLACEMENT_3D('',#55366,#32980,#32981);
#26900=AXIS2_PLACEMENT_3D('',#55367,#32982,#32983);
#26901=AXIS2_PLACEMENT_3D('',#55368,#32984,#32985);
#26902=AXIS2_PLACEMENT_3D('',#55369,#32986,#32987);
#26903=AXIS2_PLACEMENT_3D('',#55375,#32991,#32992);
#26904=AXIS2_PLACEMENT_3D('',#55379,#32995,#32996);
#26905=AXIS2_PLACEMENT_3D('',#55383,#32999,#33000);
#26906=AXIS2_PLACEMENT_3D('',#55387,#33003,#33004);
#26907=AXIS2_PLACEMENT_3D('',#55391,#33007,#33008);
#26908=AXIS2_PLACEMENT_3D('',#55395,#33011,#33012);
#26909=AXIS2_PLACEMENT_3D('',#55399,#33015,#33016);
#26910=AXIS2_PLACEMENT_3D('',#55403,#33019,#33020);
#26911=AXIS2_PLACEMENT_3D('',#55407,#33023,#33024);
#26912=AXIS2_PLACEMENT_3D('',#55411,#33027,#33028);
#26913=AXIS2_PLACEMENT_3D('',#55413,#33029,#33030);
#26914=AXIS2_PLACEMENT_3D('',#55415,#33032,#33033);
#26915=AXIS2_PLACEMENT_3D('',#55419,#33036,#33037);
#26916=AXIS2_PLACEMENT_3D('',#55421,#33038,#33039);
#26917=AXIS2_PLACEMENT_3D('',#55423,#33041,#33042);
#26918=AXIS2_PLACEMENT_3D('',#55427,#33045,#33046);
#26919=AXIS2_PLACEMENT_3D('',#55429,#33047,#33048);
#26920=AXIS2_PLACEMENT_3D('',#55431,#33050,#33051);
#26921=AXIS2_PLACEMENT_3D('',#55433,#33052,#33053);
#26922=AXIS2_PLACEMENT_3D('',#55435,#33055,#33056);
#26923=AXIS2_PLACEMENT_3D('',#55437,#33057,#33058);
#26924=AXIS2_PLACEMENT_3D('',#55439,#33060,#33061);
#26925=AXIS2_PLACEMENT_3D('',#55443,#33064,#33065);
#26926=AXIS2_PLACEMENT_3D('',#55445,#33066,#33067);
#26927=AXIS2_PLACEMENT_3D('',#55447,#33069,#33070);
#26928=AXIS2_PLACEMENT_3D('',#55451,#33073,#33074);
#26929=AXIS2_PLACEMENT_3D('',#55453,#33075,#33076);
#26930=AXIS2_PLACEMENT_3D('',#55455,#33078,#33079);
#26931=AXIS2_PLACEMENT_3D('',#55459,#33082,#33083);
#26932=AXIS2_PLACEMENT_3D('',#55461,#33084,#33085);
#26933=AXIS2_PLACEMENT_3D('',#55463,#33087,#33088);
#26934=AXIS2_PLACEMENT_3D('',#55465,#33089,#33090);
#26935=AXIS2_PLACEMENT_3D('',#55467,#33092,#33093);
#26936=AXIS2_PLACEMENT_3D('',#55469,#33094,#33095);
#26937=AXIS2_PLACEMENT_3D('',#55471,#33097,#33098);
#26938=AXIS2_PLACEMENT_3D('',#55475,#33101,#33102);
#26939=AXIS2_PLACEMENT_3D('',#55479,#33105,#33106);
#26940=AXIS2_PLACEMENT_3D('',#55483,#33109,#33110);
#26941=AXIS2_PLACEMENT_3D('',#55485,#33111,#33112);
#26942=AXIS2_PLACEMENT_3D('',#55487,#33114,#33115);
#26943=AXIS2_PLACEMENT_3D('',#55489,#33116,#33117);
#26944=AXIS2_PLACEMENT_3D('',#55491,#33119,#33120);
#26945=AXIS2_PLACEMENT_3D('',#55493,#33121,#33122);
#26946=AXIS2_PLACEMENT_3D('',#55495,#33124,#33125);
#26947=AXIS2_PLACEMENT_3D('',#55499,#33128,#33129);
#26948=AXIS2_PLACEMENT_3D('',#55501,#33130,#33131);
#26949=AXIS2_PLACEMENT_3D('',#55503,#33133,#33134);
#26950=AXIS2_PLACEMENT_3D('',#55507,#33137,#33138);
#26951=AXIS2_PLACEMENT_3D('',#55509,#33139,#33140);
#26952=AXIS2_PLACEMENT_3D('',#55511,#33142,#33143);
#26953=AXIS2_PLACEMENT_3D('',#55515,#33146,#33147);
#26954=AXIS2_PLACEMENT_3D('',#55517,#33148,#33149);
#26955=AXIS2_PLACEMENT_3D('',#55519,#33151,#33152);
#26956=AXIS2_PLACEMENT_3D('',#55521,#33153,#33154);
#26957=AXIS2_PLACEMENT_3D('',#55523,#33156,#33157);
#26958=AXIS2_PLACEMENT_3D('',#55525,#33158,#33159);
#26959=AXIS2_PLACEMENT_3D('',#55527,#33161,#33162);
#26960=AXIS2_PLACEMENT_3D('',#55531,#33165,#33166);
#26961=AXIS2_PLACEMENT_3D('',#55533,#33167,#33168);
#26962=AXIS2_PLACEMENT_3D('',#55535,#33170,#33171);
#26963=AXIS2_PLACEMENT_3D('',#55539,#33174,#33175);
#26964=AXIS2_PLACEMENT_3D('',#55541,#33176,#33177);
#26965=AXIS2_PLACEMENT_3D('',#55543,#33179,#33180);
#26966=AXIS2_PLACEMENT_3D('',#55545,#33182,#33183);
#26967=AXIS2_PLACEMENT_3D('',#55554,#33188,#33189);
#26968=AXIS2_PLACEMENT_3D('',#55560,#33193,#33194);
#26969=AXIS2_PLACEMENT_3D('',#55566,#33198,#33199);
#26970=AXIS2_PLACEMENT_3D('',#55572,#33203,#33204);
#26971=AXIS2_PLACEMENT_3D('',#55578,#33208,#33209);
#26972=AXIS2_PLACEMENT_3D('',#55587,#33214,#33215);
#26973=AXIS2_PLACEMENT_3D('',#55593,#33219,#33220);
#26974=AXIS2_PLACEMENT_3D('',#55599,#33224,#33225);
#26975=AXIS2_PLACEMENT_3D('',#55602,#33228,#33229);
#26976=AXIS2_PLACEMENT_3D('',#55610,#33234,#33235);
#26977=AXIS2_PLACEMENT_3D('',#55616,#33239,#33240);
#26978=AXIS2_PLACEMENT_3D('',#55622,#33244,#33245);
#26979=AXIS2_PLACEMENT_3D('',#55628,#33249,#33250);
#26980=AXIS2_PLACEMENT_3D('',#55634,#33254,#33255);
#26981=AXIS2_PLACEMENT_3D('',#55640,#33259,#33260);
#26982=AXIS2_PLACEMENT_3D('',#55646,#33264,#33265);
#26983=AXIS2_PLACEMENT_3D('',#55652,#33269,#33270);
#26984=AXIS2_PLACEMENT_3D('',#55658,#33274,#33275);
#26985=AXIS2_PLACEMENT_3D('',#55664,#33279,#33280);
#26986=AXIS2_PLACEMENT_3D('',#55670,#33284,#33285);
#26987=AXIS2_PLACEMENT_3D('',#55676,#33289,#33290);
#26988=AXIS2_PLACEMENT_3D('',#55682,#33294,#33295);
#26989=AXIS2_PLACEMENT_3D('',#55688,#33299,#33300);
#26990=AXIS2_PLACEMENT_3D('',#55693,#33304,#33305);
#26991=AXIS2_PLACEMENT_3D('',#55695,#33306,#33307);
#26992=AXIS2_PLACEMENT_3D('',#55699,#33310,#33311);
#26993=AXIS2_PLACEMENT_3D('',#55705,#33315,#33316);
#26994=AXIS2_PLACEMENT_3D('',#55707,#33317,#33318);
#26995=AXIS2_PLACEMENT_3D('',#55711,#33321,#33322);
#26996=AXIS2_PLACEMENT_3D('',#55713,#33323,#33324);
#26997=AXIS2_PLACEMENT_3D('',#55717,#33327,#33328);
#26998=AXIS2_PLACEMENT_3D('',#55723,#33332,#33333);
#26999=AXIS2_PLACEMENT_3D('',#55725,#33335,#33336);
#27000=AXIS2_PLACEMENT_3D('',#55726,#33337,#33338);
#27001=AXIS2_PLACEMENT_3D('',#55727,#33339,#33340);
#27002=AXIS2_PLACEMENT_3D('',#55731,#33343,#33344);
#27003=AXIS2_PLACEMENT_3D('',#55737,#33348,#33349);
#27004=AXIS2_PLACEMENT_3D('',#55743,#33353,#33354);
#27005=AXIS2_PLACEMENT_3D('',#55748,#33358,#33359);
#27006=AXIS2_PLACEMENT_3D('',#55749,#33360,#33361);
#27007=AXIS2_PLACEMENT_3D('',#55751,#33363,#33364);
#27008=AXIS2_PLACEMENT_3D('',#55757,#33367,#33368);
#27009=AXIS2_PLACEMENT_3D('',#55761,#33370,#33371);
#27010=AXIS2_PLACEMENT_3D('',#55765,#33373,#33374);
#27011=AXIS2_PLACEMENT_3D('',#55767,#33375,#33376);
#27012=AXIS2_PLACEMENT_3D('',#55769,#33377,#33378);
#27013=AXIS2_PLACEMENT_3D('',#55773,#33380,#33381);
#27014=AXIS2_PLACEMENT_3D('',#55777,#33383,#33384);
#27015=AXIS2_PLACEMENT_3D('',#55781,#33386,#33387);
#27016=AXIS2_PLACEMENT_3D('',#55783,#33388,#33389);
#27017=AXIS2_PLACEMENT_3D('',#55785,#33390,#33391);
#27018=AXIS2_PLACEMENT_3D('',#55793,#33395,#33396);
#27019=AXIS2_PLACEMENT_3D('',#55795,#33397,#33398);
#27020=AXIS2_PLACEMENT_3D('',#55797,#33399,#33400);
#27021=AXIS2_PLACEMENT_3D('',#55801,#33402,#33403);
#27022=AXIS2_PLACEMENT_3D('',#55805,#33405,#33406);
#27023=AXIS2_PLACEMENT_3D('',#55809,#33408,#33409);
#27024=AXIS2_PLACEMENT_3D('',#55811,#33410,#33411);
#27025=AXIS2_PLACEMENT_3D('',#55813,#33412,#33413);
#27026=AXIS2_PLACEMENT_3D('',#55817,#33415,#33416);
#27027=AXIS2_PLACEMENT_3D('',#55821,#33418,#33419);
#27028=AXIS2_PLACEMENT_3D('',#55825,#33422,#33423);
#27029=AXIS2_PLACEMENT_3D('',#55851,#33437,#33438);
#27030=AXIS2_PLACEMENT_3D('',#55857,#33442,#33443);
#27031=AXIS2_PLACEMENT_3D('',#55863,#33447,#33448);
#27032=AXIS2_PLACEMENT_3D('',#55867,#33451,#33452);
#27033=AXIS2_PLACEMENT_3D('',#55871,#33455,#33456);
#27034=AXIS2_PLACEMENT_3D('',#55875,#33459,#33460);
#27035=AXIS2_PLACEMENT_3D('',#55879,#33462,#33463);
#27036=AXIS2_PLACEMENT_3D('',#55881,#33465,#33466);
#27037=AXIS2_PLACEMENT_3D('',#55885,#33468,#33469);
#27038=AXIS2_PLACEMENT_3D('',#55887,#33471,#33472);
#27039=AXIS2_PLACEMENT_3D('',#55889,#33474,#33475);
#27040=AXIS2_PLACEMENT_3D('',#55893,#33478,#33479);
#27041=AXIS2_PLACEMENT_3D('',#55895,#33481,#33482);
#27042=AXIS2_PLACEMENT_3D('',#55898,#33483,#33484);
#27043=AXIS2_PLACEMENT_3D('',#55901,#33487,#33488);
#27044=AXIS2_PLACEMENT_3D('',#55904,#33489,#33490);
#27045=AXIS2_PLACEMENT_3D('',#55907,#33493,#33494);
#27046=AXIS2_PLACEMENT_3D('',#55908,#33495,#33496);
#27047=AXIS2_PLACEMENT_3D('',#55909,#33497,#33498);
#27048=AXIS2_PLACEMENT_3D('',#55912,#33499,#33500);
#27049=AXIS2_PLACEMENT_3D('',#55915,#33503,#33504);
#27050=AXIS2_PLACEMENT_3D('',#55918,#33505,#33506);
#27051=AXIS2_PLACEMENT_3D('',#55921,#33509,#33510);
#27052=AXIS2_PLACEMENT_3D('',#55923,#33512,#33513);
#27053=AXIS2_PLACEMENT_3D('',#55925,#33515,#33516);
#27054=AXIS2_PLACEMENT_3D('',#55928,#33517,#33518);
#27055=AXIS2_PLACEMENT_3D('',#55931,#33521,#33522);
#27056=AXIS2_PLACEMENT_3D('',#55934,#33523,#33524);
#27057=AXIS2_PLACEMENT_3D('',#55937,#33527,#33528);
#27058=AXIS2_PLACEMENT_3D('',#55938,#33529,#33530);
#27059=AXIS2_PLACEMENT_3D('',#55939,#33531,#33532);
#27060=AXIS2_PLACEMENT_3D('',#55945,#33536,#33537);
#27061=AXIS2_PLACEMENT_3D('',#55947,#33539,#33540);
#27062=AXIS2_PLACEMENT_3D('',#55950,#33541,#33542);
#27063=AXIS2_PLACEMENT_3D('',#55953,#33545,#33546);
#27064=AXIS2_PLACEMENT_3D('',#55956,#33547,#33548);
#27065=AXIS2_PLACEMENT_3D('',#55959,#33551,#33552);
#27066=AXIS2_PLACEMENT_3D('',#55960,#33553,#33554);
#27067=AXIS2_PLACEMENT_3D('',#55961,#33555,#33556);
#27068=AXIS2_PLACEMENT_3D('',#55964,#33557,#33558);
#27069=AXIS2_PLACEMENT_3D('',#55967,#33561,#33562);
#27070=AXIS2_PLACEMENT_3D('',#55970,#33563,#33564);
#27071=AXIS2_PLACEMENT_3D('',#55973,#33567,#33568);
#27072=AXIS2_PLACEMENT_3D('',#55975,#33570,#33571);
#27073=AXIS2_PLACEMENT_3D('',#55977,#33573,#33574);
#27074=AXIS2_PLACEMENT_3D('',#55979,#33576,#33577);
#27075=AXIS2_PLACEMENT_3D('',#55982,#33578,#33579);
#27076=AXIS2_PLACEMENT_3D('',#55985,#33582,#33583);
#27077=AXIS2_PLACEMENT_3D('',#55988,#33584,#33585);
#27078=AXIS2_PLACEMENT_3D('',#55991,#33588,#33589);
#27079=AXIS2_PLACEMENT_3D('',#55992,#33590,#33591);
#27080=AXIS2_PLACEMENT_3D('',#55993,#33592,#33593);
#27081=AXIS2_PLACEMENT_3D('',#55997,#33595,#33596);
#27082=AXIS2_PLACEMENT_3D('',#55999,#33598,#33599);
#27083=AXIS2_PLACEMENT_3D('',#56003,#33601,#33602);
#27084=AXIS2_PLACEMENT_3D('',#56005,#33604,#33605);
#27085=AXIS2_PLACEMENT_3D('',#56011,#33609,#33610);
#27086=AXIS2_PLACEMENT_3D('',#56015,#33613,#33614);
#27087=AXIS2_PLACEMENT_3D('',#56019,#33617,#33618);
#27088=AXIS2_PLACEMENT_3D('',#56021,#33620,#33621);
#27089=AXIS2_PLACEMENT_3D('',#56025,#33624,#33625);
#27090=AXIS2_PLACEMENT_3D('',#56027,#33627,#33628);
#27091=AXIS2_PLACEMENT_3D('',#56029,#33630,#33631);
#27092=AXIS2_PLACEMENT_3D('',#56031,#33633,#33634);
#27093=AXIS2_PLACEMENT_3D('',#56033,#33636,#33637);
#27094=AXIS2_PLACEMENT_3D('',#56035,#33639,#33640);
#27095=AXIS2_PLACEMENT_3D('',#56037,#33642,#33643);
#27096=AXIS2_PLACEMENT_3D('',#56041,#33646,#33647);
#27097=AXIS2_PLACEMENT_3D('',#56043,#33649,#33650);
#27098=AXIS2_PLACEMENT_3D('',#56044,#33651,#33652);
#27099=AXIS2_PLACEMENT_3D('',#56048,#33655,#33656);
#27100=AXIS2_PLACEMENT_3D('',#56050,#33657,#33658);
#27101=AXIS2_PLACEMENT_3D('',#56052,#33660,#33661);
#27102=AXIS2_PLACEMENT_3D('',#56054,#33663,#33664);
#27103=AXIS2_PLACEMENT_3D('',#56055,#33665,#33666);
#27104=AXIS2_PLACEMENT_3D('',#56056,#33667,#33668);
#27105=AXIS2_PLACEMENT_3D('',#56057,#33669,#33670);
#27106=AXIS2_PLACEMENT_3D('',#56058,#33671,#33672);
#31779=DIRECTION('axis',(0.,0.,1.));
#31780=DIRECTION('refdir',(1.,0.,0.));
#31781=DIRECTION('center_axis',(1.,0.,0.));
#31782=DIRECTION('ref_axis',(0.,0.,-1.));
#31783=DIRECTION('center_axis',(1.,0.,0.));
#31784=DIRECTION('ref_axis',(0.,0.,-1.));
#31785=DIRECTION('',(1.,0.,0.));
#31786=DIRECTION('center_axis',(1.,0.,0.));
#31787=DIRECTION('ref_axis',(0.,0.,-1.));
#31788=DIRECTION('center_axis',(-1.,0.,0.));
#31789=DIRECTION('ref_axis',(0.,0.,1.));
#31790=DIRECTION('center_axis',(-1.,0.,0.));
#31791=DIRECTION('ref_axis',(0.,0.,1.));
#31792=DIRECTION('',(-1.,0.,0.));
#31793=DIRECTION('center_axis',(-1.,0.,0.));
#31794=DIRECTION('ref_axis',(0.,0.,1.));
#31795=DIRECTION('center_axis',(-1.30104260698261E-15,1.,-1.73611473352215E-31));
#31796=DIRECTION('ref_axis',(-1.,-1.30104260698261E-15,-2.16593351677506E-47));
#31797=DIRECTION('center_axis',(-1.30104260698261E-15,1.,-1.73611473352215E-31));
#31798=DIRECTION('ref_axis',(-1.,-1.30104260698261E-15,-2.16593351677507E-47));
#31799=DIRECTION('',(-1.30104260698261E-15,1.,-1.73611473352215E-31));
#31800=DIRECTION('center_axis',(-1.30104260698261E-15,1.,-1.73611473352215E-31));
#31801=DIRECTION('ref_axis',(-1.,-1.30104260698261E-15,-2.16593351677507E-47));
#31802=DIRECTION('center_axis',(1.,0.,0.));
#31803=DIRECTION('ref_axis',(0.,0.,-1.));
#31804=DIRECTION('',(0.515038074910055,-1.04972719113862E-16,0.857167300702112));
#31805=DIRECTION('center_axis',(-1.,0.,0.));
#31806=DIRECTION('ref_axis',(0.,0.,1.));
#31807=DIRECTION('',(-0.515038074910054,-1.04972719113862E-16,-0.857167300702112));
#31808=DIRECTION('center_axis',(0.,1.,0.));
#31809=DIRECTION('ref_axis',(0.,0.,1.));
#31810=DIRECTION('center_axis',(-1.2823896663807E-16,1.,0.));
#31811=DIRECTION('ref_axis',(-1.,-1.2823896663807E-16,0.));
#31812=DIRECTION('',(0.,1.,0.));
#31813=DIRECTION('center_axis',(0.,1.,0.));
#31814=DIRECTION('ref_axis',(0.,0.,1.));
#31815=DIRECTION('center_axis',(0.,1.,0.));
#31816=DIRECTION('ref_axis',(0.,0.,1.));
#31817=DIRECTION('center_axis',(-1.2823896663807E-16,1.,0.));
#31818=DIRECTION('ref_axis',(-1.,-1.2823896663807E-16,0.));
#31819=DIRECTION('',(0.,1.,0.));
#31820=DIRECTION('center_axis',(0.,1.,0.));
#31821=DIRECTION('ref_axis',(0.,0.,1.));
#31822=DIRECTION('center_axis',(0.,1.,0.));
#31823=DIRECTION('ref_axis',(0.,0.,1.));
#31824=DIRECTION('center_axis',(1.2823896663807E-16,1.,0.));
#31825=DIRECTION('ref_axis',(-1.,1.2823896663807E-16,0.));
#31826=DIRECTION('',(0.,1.,0.));
#31827=DIRECTION('center_axis',(0.,1.,0.));
#31828=DIRECTION('ref_axis',(0.,0.,1.));
#31829=DIRECTION('center_axis',(0.,1.,0.));
#31830=DIRECTION('ref_axis',(0.,0.,1.));
#31831=DIRECTION('center_axis',(1.2823896663807E-16,1.,0.));
#31832=DIRECTION('ref_axis',(-1.,1.2823896663807E-16,0.));
#31833=DIRECTION('',(0.,1.,0.));
#31834=DIRECTION('center_axis',(0.,1.,0.));
#31835=DIRECTION('ref_axis',(0.,0.,1.));
#31836=DIRECTION('center_axis',(-1.,0.,0.));
#31837=DIRECTION('ref_axis',(0.,0.,1.));
#31838=DIRECTION('center_axis',(-1.,0.,0.));
#31839=DIRECTION('ref_axis',(0.,0.,1.));
#31840=DIRECTION('',(-1.,0.,0.));
#31841=DIRECTION('center_axis',(-1.,0.,0.));
#31842=DIRECTION('ref_axis',(0.,0.,1.));
#31843=DIRECTION('center_axis',(1.,0.,0.));
#31844=DIRECTION('ref_axis',(0.,0.,-1.));
#31845=DIRECTION('center_axis',(1.,0.,0.));
#31846=DIRECTION('ref_axis',(0.,0.,-1.));
#31847=DIRECTION('',(1.,0.,0.));
#31848=DIRECTION('center_axis',(1.,0.,0.));
#31849=DIRECTION('ref_axis',(0.,0.,-1.));
#31850=DIRECTION('center_axis',(-1.30104260698261E-15,1.,-1.73611473352215E-31));
#31851=DIRECTION('ref_axis',(-1.,-1.30104260698261E-15,-2.16593351677506E-47));
#31852=DIRECTION('center_axis',(-1.30104260698261E-15,1.,-1.73611473352215E-31));
#31853=DIRECTION('ref_axis',(-1.,-1.30104260698261E-15,-2.16593351677507E-47));
#31854=DIRECTION('',(-1.30104260698261E-15,1.,-1.73611473352215E-31));
#31855=DIRECTION('center_axis',(-1.30104260698261E-15,1.,-1.73611473352215E-31));
#31856=DIRECTION('ref_axis',(-1.,-1.30104260698261E-15,-2.16593351677507E-47));
#31857=DIRECTION('center_axis',(-1.30104260698261E-15,1.,-1.73611473352215E-31));
#31858=DIRECTION('ref_axis',(-1.,-1.30104260698261E-15,2.25875923892257E-46));
#31859=DIRECTION('center_axis',(-1.30104260698261E-15,1.,-1.73611473352215E-31));
#31860=DIRECTION('ref_axis',(-1.,-1.30104260698261E-15,2.25875923892257E-46));
#31861=DIRECTION('',(-1.30104260698261E-15,1.,-1.73611473352215E-31));
#31862=DIRECTION('center_axis',(-1.30104260698261E-15,1.,-1.73611473352215E-31));
#31863=DIRECTION('ref_axis',(-1.,-1.30104260698261E-15,2.25875923892257E-46));
#31864=DIRECTION('',(-1.30104260698261E-15,1.,-1.73611473352215E-31));
#31865=DIRECTION('center_axis',(-1.30104260698261E-15,1.,-1.73611473352215E-31));
#31866=DIRECTION('ref_axis',(-1.,-1.30104260698261E-15,2.25875923892257E-46));
#31867=DIRECTION('',(-1.30104260698261E-15,1.,-1.73611473352215E-31));
#31868=DIRECTION('center_axis',(-1.,0.,0.));
#31869=DIRECTION('ref_axis',(0.,0.,1.));
#31870=DIRECTION('',(-0.515038074910054,-1.04972719113862E-16,-0.857167300702112));
#31871=DIRECTION('center_axis',(1.,0.,0.));
#31872=DIRECTION('ref_axis',(0.,0.,-1.));
#31873=DIRECTION('',(0.515038074910055,-1.04972719113862E-16,0.857167300702112));
#31874=DIRECTION('center_axis',(-1.30104260698261E-15,1.,-1.73611473352215E-31));
#31875=DIRECTION('ref_axis',(-1.,-1.30104260698261E-15,2.25875923892257E-46));
#31876=DIRECTION('center_axis',(-1.30104260698261E-15,1.,-1.73611473352215E-31));
#31877=DIRECTION('ref_axis',(-1.,-1.30104260698261E-15,2.25875923892257E-46));
#31878=DIRECTION('',(-1.30104260698261E-15,1.,-1.73611473352215E-31));
#31879=DIRECTION('',(-1.30104260698261E-15,1.,-1.73611473352215E-31));
#31880=DIRECTION('center_axis',(-1.30104260698261E-15,1.,-1.73611473352215E-31));
#31881=DIRECTION('ref_axis',(-1.,-1.30104260698261E-15,2.25875923892257E-46));
#31882=DIRECTION('',(-1.30104260698261E-15,1.,-1.73611473352215E-31));
#31883=DIRECTION('center_axis',(-1.30104260698261E-15,1.,-1.73611473352215E-31));
#31884=DIRECTION('ref_axis',(-1.,-1.30104260698261E-15,2.25875923892257E-46));
#31885=DIRECTION('center_axis',(0.,0.,1.));
#31886=DIRECTION('ref_axis',(-1.,0.,0.));
#31887=DIRECTION('center_axis',(0.,0.,1.));
#31888=DIRECTION('ref_axis',(-1.,0.,0.));
#31889=DIRECTION('center_axis',(0.,0.,1.));
#31890=DIRECTION('ref_axis',(1.,0.,0.));
#31891=DIRECTION('center_axis',(0.,0.,-1.));
#31892=DIRECTION('ref_axis',(-1.,0.,0.));
#31893=DIRECTION('',(0.,0.,-1.));
#31894=DIRECTION('center_axis',(0.,0.,-1.));
#31895=DIRECTION('ref_axis',(-1.,0.,0.));
#31896=DIRECTION('center_axis',(0.,0.,-1.));
#31897=DIRECTION('ref_axis',(-1.,0.,0.));
#31898=DIRECTION('',(0.,0.,-1.));
#31899=DIRECTION('center_axis',(0.,0.,-1.));
#31900=DIRECTION('ref_axis',(-1.,0.,0.));
#31901=DIRECTION('center_axis',(0.61566147532566,-0.788010753606721,0.));
#31902=DIRECTION('ref_axis',(0.78801075360672,0.61566147532566,0.));
#31903=DIRECTION('center_axis',(0.615661475325656,-0.788010753606724,-5.22755357805913E-15));
#31904=DIRECTION('ref_axis',(0.788010753606724,0.615661475325656,-5.17730530723809E-13));
#31905=DIRECTION('',(0.,0.,1.));
#31906=DIRECTION('',(0.78801075360672,0.61566147532566,0.));
#31907=DIRECTION('',(0.,0.,1.));
#31908=DIRECTION('center_axis',(0.61566147532566,-0.788010753606721,0.));
#31909=DIRECTION('ref_axis',(0.78801075360672,0.61566147532566,0.));
#31910=DIRECTION('center_axis',(0.615661475325656,-0.788010753606724,5.27148259972344E-15));
#31911=DIRECTION('ref_axis',(0.788010753606724,0.615661475325656,-9.16833363821094E-14));
#31912=DIRECTION('',(0.,0.,1.));
#31913=DIRECTION('center_axis',(0.615661475325662,-0.788010753606719,1.40572869325959E-15));
#31914=DIRECTION('ref_axis',(0.788010753606719,0.615661475325662,-7.1472163446861E-13));
#31915=DIRECTION('',(0.,0.,1.));
#31916=DIRECTION('center_axis',(-0.61566147532566,-0.788010753606721,0.));
#31917=DIRECTION('ref_axis',(0.78801075360672,-0.61566147532566,0.));
#31918=DIRECTION('center_axis',(-0.615661475325663,-0.788010753606718,-3.73396684147081E-15));
#31919=DIRECTION('ref_axis',(0.788010753606718,-0.615661475325663,1.05496270744081E-13));
#31920=DIRECTION('',(0.,0.,1.));
#31921=DIRECTION('center_axis',(-0.615661475325666,-0.788010753606716,6.32577911966821E-15));
#31922=DIRECTION('ref_axis',(0.788010753606716,-0.615661475325666,2.12834187078208E-13));
#31923=DIRECTION('',(0.,0.,1.));
#31924=DIRECTION('center_axis',(-0.61566147532566,-0.788010753606721,0.));
#31925=DIRECTION('ref_axis',(0.78801075360672,-0.61566147532566,0.));
#31926=DIRECTION('center_axis',(-0.615661475325663,-0.788010753606718,-3.64610879814206E-15));
#31927=DIRECTION('ref_axis',(0.788010753606718,-0.615661475325663,-2.42930938978673E-14));
#31928=DIRECTION('',(0.,0.,1.));
#31929=DIRECTION('',(0.78801075360672,-0.61566147532566,0.));
#31930=DIRECTION('',(0.,0.,1.));
#31931=DIRECTION('center_axis',(-0.707106781186546,0.707106781186549,0.));
#31932=DIRECTION('ref_axis',(-0.707106781186549,-0.707106781186546,0.));
#31933=DIRECTION('',(-0.707106781186549,-0.707106781186546,0.));
#31934=DIRECTION('',(0.,0.,-1.));
#31935=DIRECTION('',(-0.707106781186549,-0.707106781186546,0.));
#31936=DIRECTION('',(0.,0.,1.));
#31937=DIRECTION('center_axis',(-0.707106781186549,-0.707106781186546,0.));
#31938=DIRECTION('ref_axis',(0.707106781186546,-0.707106781186549,0.));
#31939=DIRECTION('',(0.707106781186545,-0.70710678118655,0.));
#31940=DIRECTION('',(0.,0.,-1.));
#31941=DIRECTION('',(0.707106781186546,-0.707106781186549,0.));
#31942=DIRECTION('',(0.,0.,1.));
#31943=DIRECTION('center_axis',(0.707106781186546,0.707106781186549,0.));
#31944=DIRECTION('ref_axis',(-0.707106781186549,0.707106781186546,0.));
#31945=DIRECTION('',(-0.707106781186548,0.707106781186547,0.));
#31946=DIRECTION('',(0.,0.,-1.));
#31947=DIRECTION('',(-0.707106781186549,0.707106781186546,0.));
#31948=DIRECTION('',(0.,0.,1.));
#31949=DIRECTION('center_axis',(0.707106781186549,-0.707106781186546,0.));
#31950=DIRECTION('ref_axis',(0.707106781186546,0.707106781186549,0.));
#31951=DIRECTION('',(0.707106781186546,0.707106781186549,0.));
#31952=DIRECTION('',(0.,0.,-1.));
#31953=DIRECTION('',(0.707106781186546,0.707106781186549,0.));
#31954=DIRECTION('',(0.,0.,1.));
#31955=DIRECTION('center_axis',(0.707106781186549,-0.707106781186546,0.));
#31956=DIRECTION('ref_axis',(0.707106781186546,0.707106781186549,0.));
#31957=DIRECTION('',(0.707106781186545,0.70710678118655,0.));
#31958=DIRECTION('',(0.,0.,-1.));
#31959=DIRECTION('',(0.707106781186546,0.707106781186549,0.));
#31960=DIRECTION('',(0.,0.,1.));
#31961=DIRECTION('center_axis',(1.,0.,0.));
#31962=DIRECTION('ref_axis',(0.,0.,-1.));
#31963=DIRECTION('',(0.,1.,0.));
#31964=DIRECTION('',(0.,0.,-1.));
#31965=DIRECTION('',(0.,1.,0.));
#31966=DIRECTION('',(0.,0.,1.));
#31967=DIRECTION('center_axis',(0.707106781186546,0.707106781186549,0.));
#31968=DIRECTION('ref_axis',(-0.707106781186549,0.707106781186546,0.));
#31969=DIRECTION('',(-0.707106781186549,0.707106781186546,0.));
#31970=DIRECTION('',(0.,0.,-1.));
#31971=DIRECTION('',(-0.707106781186549,0.707106781186546,0.));
#31972=DIRECTION('',(0.,0.,1.));
#31973=DIRECTION('center_axis',(1.,0.,0.));
#31974=DIRECTION('ref_axis',(0.,0.,-1.));
#31975=DIRECTION('',(0.,1.,0.));
#31976=DIRECTION('',(0.,0.,-1.));
#31977=DIRECTION('',(0.,1.,0.));
#31978=DIRECTION('',(0.,0.,1.));
#31979=DIRECTION('center_axis',(0.707106781186549,-0.707106781186546,0.));
#31980=DIRECTION('ref_axis',(0.707106781186546,0.707106781186549,0.));
#31981=DIRECTION('',(0.707106781186546,0.707106781186549,0.));
#31982=DIRECTION('',(0.,0.,1.));
#31983=DIRECTION('',(0.707106781186546,0.707106781186549,0.));
#31984=DIRECTION('',(0.,0.,1.));
#31985=DIRECTION('center_axis',(0.,-1.,0.));
#31986=DIRECTION('ref_axis',(0.,0.,-1.));
#31987=DIRECTION('',(1.,0.,0.));
#31988=DIRECTION('',(0.,0.,1.));
#31989=DIRECTION('',(1.,0.,0.));
#31990=DIRECTION('center_axis',(-6.49101394191508E-16,-1.,0.));
#31991=DIRECTION('ref_axis',(1.,-6.49101394191508E-16,0.));
#31992=DIRECTION('',(1.,-3.50803534070133E-16,0.));
#31993=DIRECTION('',(0.,0.,1.));
#31994=DIRECTION('',(1.,-6.49101394191508E-16,0.));
#31995=DIRECTION('',(0.,0.,1.));
#31996=DIRECTION('center_axis',(-0.707106781186549,-0.707106781186546,0.));
#31997=DIRECTION('ref_axis',(0.707106781186546,-0.707106781186549,0.));
#31998=DIRECTION('',(0.707106781186546,-0.707106781186549,0.));
#31999=DIRECTION('',(0.,0.,-1.));
#32000=DIRECTION('',(0.707106781186546,-0.707106781186549,0.));
#32001=DIRECTION('center_axis',(-1.,0.,0.));
#32002=DIRECTION('ref_axis',(0.,0.,1.));
#32003=DIRECTION('',(0.,-1.,0.));
#32004=DIRECTION('',(0.,0.,-1.));
#32005=DIRECTION('',(0.,-1.,0.));
#32006=DIRECTION('',(0.,0.,1.));
#32007=DIRECTION('center_axis',(-0.707106781186546,0.707106781186549,0.));
#32008=DIRECTION('ref_axis',(-0.707106781186549,-0.707106781186546,0.));
#32009=DIRECTION('',(-0.707106781186548,-0.707106781186547,0.));
#32010=DIRECTION('',(0.,0.,-1.));
#32011=DIRECTION('',(-0.707106781186549,-0.707106781186546,0.));
#32012=DIRECTION('',(0.,0.,1.));
#32013=DIRECTION('center_axis',(-1.,0.,0.));
#32014=DIRECTION('ref_axis',(0.,0.,1.));
#32015=DIRECTION('',(0.,-1.,0.));
#32016=DIRECTION('',(0.,0.,-1.));
#32017=DIRECTION('',(0.,-1.,0.));
#32018=DIRECTION('',(0.,0.,1.));
#32019=DIRECTION('center_axis',(-0.707106781186549,-0.707106781186546,0.));
#32020=DIRECTION('ref_axis',(0.707106781186546,-0.707106781186549,0.));
#32021=DIRECTION('',(0.707106781186546,-0.707106781186549,0.));
#32022=DIRECTION('',(0.,0.,1.));
#32023=DIRECTION('',(0.707106781186546,-0.707106781186549,0.));
#32024=DIRECTION('',(0.,0.,1.));
#32025=DIRECTION('center_axis',(1.22464679914735E-16,-1.,0.));
#32026=DIRECTION('ref_axis',(1.,1.22464679914735E-16,0.));
#32027=DIRECTION('',(1.,1.22464679914735E-16,0.));
#32028=DIRECTION('',(1.,1.22464679914735E-16,0.));
#32029=DIRECTION('center_axis',(0.,0.,1.));
#32030=DIRECTION('ref_axis',(1.,0.,0.));
#32031=DIRECTION('center_axis',(0.,0.,1.));
#32032=DIRECTION('ref_axis',(1.,0.,0.));
#32033=DIRECTION('',(0.,0.,-1.));
#32034=DIRECTION('center_axis',(0.,0.,1.));
#32035=DIRECTION('ref_axis',(1.,0.,0.));
#32036=DIRECTION('',(0.,0.,1.));
#32037=DIRECTION('center_axis',(0.,0.,1.));
#32038=DIRECTION('ref_axis',(1.,0.,0.));
#32039=DIRECTION('center_axis',(0.,0.,1.));
#32040=DIRECTION('ref_axis',(1.,0.,0.));
#32041=DIRECTION('',(0.,0.,-1.));
#32042=DIRECTION('center_axis',(0.,0.,1.));
#32043=DIRECTION('ref_axis',(1.,0.,0.));
#32044=DIRECTION('',(0.,0.,1.));
#32045=DIRECTION('center_axis',(0.,0.,1.));
#32046=DIRECTION('ref_axis',(1.,0.,0.));
#32047=DIRECTION('center_axis',(0.,0.,1.));
#32048=DIRECTION('ref_axis',(1.,0.,0.));
#32049=DIRECTION('',(0.,0.,-1.));
#32050=DIRECTION('center_axis',(0.,0.,1.));
#32051=DIRECTION('ref_axis',(1.,0.,0.));
#32052=DIRECTION('',(0.,0.,1.));
#32053=DIRECTION('center_axis',(0.,0.,1.));
#32054=DIRECTION('ref_axis',(1.,0.,0.));
#32055=DIRECTION('center_axis',(0.,0.,1.));
#32056=DIRECTION('ref_axis',(1.,0.,0.));
#32057=DIRECTION('',(0.,0.,-1.));
#32058=DIRECTION('center_axis',(0.,0.,1.));
#32059=DIRECTION('ref_axis',(1.,0.,0.));
#32060=DIRECTION('',(0.,0.,1.));
#32061=DIRECTION('center_axis',(0.,0.,1.));
#32062=DIRECTION('ref_axis',(1.,0.,0.));
#32063=DIRECTION('center_axis',(0.,0.,1.));
#32064=DIRECTION('ref_axis',(1.,0.,0.));
#32065=DIRECTION('center_axis',(0.,0.,-1.));
#32066=DIRECTION('ref_axis',(-1.,0.,0.));
#32067=DIRECTION('center_axis',(0.,0.,1.));
#32068=DIRECTION('ref_axis',(1.,0.,0.));
#32069=DIRECTION('center_axis',(0.,0.,1.));
#32070=DIRECTION('ref_axis',(1.,0.,0.));
#32071=DIRECTION('center_axis',(0.,0.,-1.));
#32072=DIRECTION('ref_axis',(-1.,0.,0.));
#32073=DIRECTION('center_axis',(0.,0.,-1.));
#32074=DIRECTION('ref_axis',(-1.,0.,0.));
#32075=DIRECTION('center_axis',(0.,0.,-1.));
#32076=DIRECTION('ref_axis',(1.,0.,0.));
#32077=DIRECTION('center_axis',(0.,0.,1.));
#32078=DIRECTION('ref_axis',(-1.,0.,0.));
#32079=DIRECTION('center_axis',(0.,0.,-1.));
#32080=DIRECTION('ref_axis',(-1.,0.,0.));
#32081=DIRECTION('center_axis',(0.,0.,-1.));
#32082=DIRECTION('ref_axis',(1.,0.,0.));
#32083=DIRECTION('center_axis',(0.,0.,1.));
#32084=DIRECTION('ref_axis',(-1.,-5.20417042793042E-15,0.));
#32085=DIRECTION('center_axis',(0.,0.,1.));
#32086=DIRECTION('ref_axis',(1.,0.,0.));
#32087=DIRECTION('center_axis',(0.,0.,-1.));
#32088=DIRECTION('ref_axis',(1.,0.,0.));
#32089=DIRECTION('center_axis',(0.,0.,1.));
#32090=DIRECTION('ref_axis',(-1.,-3.46944695195361E-15,0.));
#32091=DIRECTION('center_axis',(0.,0.,1.));
#32092=DIRECTION('ref_axis',(1.,0.,0.));
#32093=DIRECTION('center_axis',(0.,0.,-1.));
#32094=DIRECTION('ref_axis',(1.,0.,0.));
#32095=DIRECTION('center_axis',(0.,0.,1.));
#32096=DIRECTION('ref_axis',(-1.,5.42101086242752E-15,0.));
#32097=DIRECTION('center_axis',(0.,0.,1.));
#32098=DIRECTION('ref_axis',(1.,0.,0.));
#32099=DIRECTION('center_axis',(0.,0.,-1.));
#32100=DIRECTION('ref_axis',(1.,0.,0.));
#32101=DIRECTION('center_axis',(0.,0.,1.));
#32102=DIRECTION('ref_axis',(-1.,-1.73472347597681E-15,0.));
#32103=DIRECTION('center_axis',(0.,0.,1.));
#32104=DIRECTION('ref_axis',(1.,0.,0.));
#32105=DIRECTION('center_axis',(0.,0.,-1.));
#32106=DIRECTION('ref_axis',(1.,0.,0.));
#32107=DIRECTION('center_axis',(0.,0.,1.));
#32108=DIRECTION('ref_axis',(-1.,8.67361737988403E-15,0.));
#32109=DIRECTION('center_axis',(0.,0.,1.));
#32110=DIRECTION('ref_axis',(1.,0.,0.));
#32111=DIRECTION('center_axis',(0.,0.,1.));
#32112=DIRECTION('ref_axis',(1.,0.,0.));
#32113=DIRECTION('center_axis',(0.,0.,-1.));
#32114=DIRECTION('ref_axis',(-1.,0.,0.));
#32115=DIRECTION('center_axis',(0.,0.,1.));
#32116=DIRECTION('ref_axis',(1.,0.,0.));
#32117=DIRECTION('center_axis',(0.,0.,1.));
#32118=DIRECTION('ref_axis',(1.,0.,0.));
#32119=DIRECTION('center_axis',(0.,0.,-1.));
#32120=DIRECTION('ref_axis',(-1.,0.,0.));
#32121=DIRECTION('center_axis',(0.,0.,1.));
#32122=DIRECTION('ref_axis',(1.,0.,0.));
#32123=DIRECTION('center_axis',(0.,0.,-1.));
#32124=DIRECTION('ref_axis',(1.,0.,0.));
#32125=DIRECTION('center_axis',(0.,0.,1.));
#32126=DIRECTION('ref_axis',(-1.,1.73472347597681E-15,0.));
#32127=DIRECTION('center_axis',(0.,0.,1.));
#32128=DIRECTION('ref_axis',(1.,0.,0.));
#32129=DIRECTION('center_axis',(0.,0.,-1.));
#32130=DIRECTION('ref_axis',(1.,0.,0.));
#32131=DIRECTION('center_axis',(0.,0.,1.));
#32132=DIRECTION('ref_axis',(-1.,0.,0.));
#32133=DIRECTION('center_axis',(0.,0.,-1.));
#32134=DIRECTION('ref_axis',(-1.,0.,0.));
#32135=DIRECTION('center_axis',(0.,0.,-1.));
#32136=DIRECTION('ref_axis',(1.,0.,0.));
#32137=DIRECTION('center_axis',(0.,0.,1.));
#32138=DIRECTION('ref_axis',(-1.,0.,0.));
#32139=DIRECTION('center_axis',(0.,0.,-1.));
#32140=DIRECTION('ref_axis',(-1.,0.,0.));
#32141=DIRECTION('center_axis',(0.,0.,-1.));
#32142=DIRECTION('ref_axis',(1.,0.,0.));
#32143=DIRECTION('center_axis',(0.,0.,1.));
#32144=DIRECTION('ref_axis',(-1.,-1.64798730217797E-14,0.));
#32145=DIRECTION('center_axis',(0.,0.,1.));
#32146=DIRECTION('ref_axis',(1.,0.,0.));
#32147=DIRECTION('center_axis',(0.,0.,-1.));
#32148=DIRECTION('ref_axis',(1.,0.,0.));
#32149=DIRECTION('center_axis',(0.,0.,1.));
#32150=DIRECTION('ref_axis',(-1.,-1.73472347597681E-14,0.));
#32151=DIRECTION('center_axis',(0.,0.,1.));
#32152=DIRECTION('ref_axis',(1.,0.,0.));
#32153=DIRECTION('center_axis',(0.,0.,-1.));
#32154=DIRECTION('ref_axis',(1.,0.,0.));
#32155=DIRECTION('center_axis',(0.,0.,1.));
#32156=DIRECTION('ref_axis',(-1.,1.95156391047391E-14,0.));
#32157=DIRECTION('center_axis',(0.,0.,-1.));
#32158=DIRECTION('ref_axis',(-1.,0.,0.));
#32159=DIRECTION('center_axis',(0.,-1.,0.));
#32160=DIRECTION('ref_axis',(0.,0.,-1.));
#32161=DIRECTION('',(0.,0.,1.));
#32162=DIRECTION('',(-1.,0.,0.));
#32163=DIRECTION('',(0.,0.,1.));
#32164=DIRECTION('',(1.,0.,0.));
#32165=DIRECTION('center_axis',(0.,0.,-1.));
#32166=DIRECTION('ref_axis',(-1.,0.,0.));
#32167=DIRECTION('',(-0.707106781186547,0.707106781186548,0.));
#32168=DIRECTION('',(-1.26161707343768E-16,1.,0.));
#32169=DIRECTION('',(0.707106781186562,0.707106781186533,0.));
#32170=DIRECTION('',(0.707106781186562,-0.707106781186533,0.));
#32171=DIRECTION('',(-1.26161707343768E-16,-1.,0.));
#32172=DIRECTION('',(-0.707106781186547,-0.707106781186548,0.));
#32173=DIRECTION('center_axis',(0.707106781186533,-0.707106781186562,0.));
#32174=DIRECTION('ref_axis',(0.707106781186562,0.707106781186533,0.));
#32175=DIRECTION('',(0.,0.,1.));
#32176=DIRECTION('',(-0.707106781186562,-0.707106781186533,0.));
#32177=DIRECTION('center_axis',(1.,1.26161707343768E-16,0.));
#32178=DIRECTION('ref_axis',(-1.26161707343768E-16,1.,0.));
#32179=DIRECTION('',(0.,0.,1.));
#32180=DIRECTION('',(1.26161707343768E-16,-1.,0.));
#32181=DIRECTION('center_axis',(0.707106781186548,0.707106781186547,0.));
#32182=DIRECTION('ref_axis',(-0.707106781186547,0.707106781186548,0.));
#32183=DIRECTION('',(0.707106781186547,-0.707106781186548,0.));
#32184=DIRECTION('center_axis',(-0.707106781186548,0.707106781186547,0.));
#32185=DIRECTION('ref_axis',(-0.707106781186547,-0.707106781186548,0.));
#32186=DIRECTION('',(0.,0.,1.));
#32187=DIRECTION('',(0.707106781186547,0.707106781186548,0.));
#32188=DIRECTION('center_axis',(-1.,1.26161707343768E-16,0.));
#32189=DIRECTION('ref_axis',(-1.26161707343768E-16,-1.,0.));
#32190=DIRECTION('',(0.,0.,1.));
#32191=DIRECTION('',(1.26161707343768E-16,1.,0.));
#32192=DIRECTION('center_axis',(-0.707106781186533,-0.707106781186562,0.));
#32193=DIRECTION('ref_axis',(0.707106781186562,-0.707106781186533,0.));
#32194=DIRECTION('',(-0.707106781186562,0.707106781186533,0.));
#32195=DIRECTION('center_axis',(-0.866025403784439,0.5,0.));
#32196=DIRECTION('ref_axis',(-0.5,-0.866025403784439,0.));
#32197=DIRECTION('',(0.,0.,-1.));
#32198=DIRECTION('',(0.,0.,-1.));
#32199=DIRECTION('',(0.5,0.866025403784439,0.));
#32200=DIRECTION('center_axis',(-0.866025403784438,-0.5,0.));
#32201=DIRECTION('ref_axis',(0.5,-0.866025403784438,0.));
#32202=DIRECTION('',(-0.5,0.866025403784438,0.));
#32203=DIRECTION('',(0.,0.,-1.));
#32204=DIRECTION('center_axis',(7.51157299368579E-16,-1.,0.));
#32205=DIRECTION('ref_axis',(1.,7.5115729936858E-16,0.));
#32206=DIRECTION('',(0.,0.,-1.));
#32207=DIRECTION('',(-1.,-7.5115729936858E-16,0.));
#32208=DIRECTION('center_axis',(0.866025403784439,-0.5,0.));
#32209=DIRECTION('ref_axis',(0.5,0.866025403784439,0.));
#32210=DIRECTION('',(0.,0.,-1.));
#32211=DIRECTION('',(-0.5,-0.866025403784439,0.));
#32212=DIRECTION('center_axis',(0.866025403784439,0.5,0.));
#32213=DIRECTION('ref_axis',(-0.5,0.866025403784439,0.));
#32214=DIRECTION('',(0.,0.,-1.));
#32215=DIRECTION('',(0.5,-0.866025403784438,0.));
#32216=DIRECTION('center_axis',(0.,1.,0.));
#32217=DIRECTION('ref_axis',(0.,0.,1.));
#32218=DIRECTION('',(1.,0.,0.));
#32219=DIRECTION('center_axis',(0.,0.,-1.));
#32220=DIRECTION('ref_axis',(-1.,0.,0.));
#32221=DIRECTION('center_axis',(0.,0.,-1.));
#32222=DIRECTION('ref_axis',(1.,0.,0.));
#32223=DIRECTION('',(0.707106781186546,-0.707106781186549,0.));
#32224=DIRECTION('center_axis',(0.,0.,1.));
#32225=DIRECTION('ref_axis',(1.,0.,0.));
#32226=DIRECTION('',(0.,-1.,0.));
#32227=DIRECTION('center_axis',(0.,0.,1.));
#32228=DIRECTION('ref_axis',(1.,0.,0.));
#32229=DIRECTION('',(-0.707106781186552,-0.707106781186543,0.));
#32230=DIRECTION('center_axis',(0.,0.,-1.));
#32231=DIRECTION('ref_axis',(1.,0.,0.));
#32232=DIRECTION('center_axis',(0.,0.,1.));
#32233=DIRECTION('ref_axis',(1.,0.,0.));
#32234=DIRECTION('center_axis',(0.,0.,-1.));
#32235=DIRECTION('ref_axis',(1.,0.,0.));
#32236=DIRECTION('',(-0.707106781186552,-0.707106781186543,0.));
#32237=DIRECTION('center_axis',(0.,0.,-1.));
#32238=DIRECTION('ref_axis',(1.,0.,0.));
#32239=DIRECTION('',(0.,-1.,0.));
#32240=DIRECTION('center_axis',(0.,0.,-1.));
#32241=DIRECTION('ref_axis',(1.,0.,0.));
#32242=DIRECTION('',(0.707106781186547,-0.707106781186547,0.));
#32243=DIRECTION('center_axis',(0.,0.,-1.));
#32244=DIRECTION('ref_axis',(1.,0.,0.));
#32245=DIRECTION('center_axis',(0.,0.,1.));
#32246=DIRECTION('ref_axis',(1.,0.,0.));
#32247=DIRECTION('center_axis',(0.,0.,-1.));
#32248=DIRECTION('ref_axis',(1.,0.,0.));
#32249=DIRECTION('',(0.707106781186546,-0.707106781186549,0.));
#32250=DIRECTION('',(1.,4.61786466713945E-17,0.));
#32251=DIRECTION('',(0.707106781186547,0.707106781186548,0.));
#32252=DIRECTION('center_axis',(0.,0.,-1.));
#32253=DIRECTION('ref_axis',(1.,0.,0.));
#32254=DIRECTION('center_axis',(0.,0.,1.));
#32255=DIRECTION('ref_axis',(1.,0.,0.));
#32256=DIRECTION('center_axis',(0.,0.,-1.));
#32257=DIRECTION('ref_axis',(1.,0.,0.));
#32258=DIRECTION('',(0.707106781186546,0.707106781186549,0.));
#32259=DIRECTION('center_axis',(0.,0.,-1.));
#32260=DIRECTION('ref_axis',(1.,0.,0.));
#32261=DIRECTION('',(0.,1.,0.));
#32262=DIRECTION('center_axis',(0.,0.,-1.));
#32263=DIRECTION('ref_axis',(1.,0.,0.));
#32264=DIRECTION('',(-0.707106781186546,0.707106781186549,0.));
#32265=DIRECTION('center_axis',(0.,0.,-1.));
#32266=DIRECTION('ref_axis',(1.,0.,0.));
#32267=DIRECTION('center_axis',(0.,0.,1.));
#32268=DIRECTION('ref_axis',(1.,0.,0.));
#32269=DIRECTION('center_axis',(0.,0.,-1.));
#32270=DIRECTION('ref_axis',(1.,0.,0.));
#32271=DIRECTION('',(-0.707106781186552,0.707106781186543,0.));
#32272=DIRECTION('center_axis',(0.,0.,1.));
#32273=DIRECTION('ref_axis',(1.,0.,0.));
#32274=DIRECTION('',(0.,1.,0.));
#32275=DIRECTION('center_axis',(0.,0.,1.));
#32276=DIRECTION('ref_axis',(1.,0.,0.));
#32277=DIRECTION('',(0.707106781186546,0.707106781186549,0.));
#32278=DIRECTION('',(1.,0.,0.));
#32279=DIRECTION('',(0.707106781186547,-0.707106781186548,0.));
#32280=DIRECTION('',(1.26352022694434E-16,-1.,0.));
#32281=DIRECTION('',(-0.707106781186562,-0.707106781186533,0.));
#32282=DIRECTION('',(-1.,-1.95534159233113E-16,0.));
#32283=DIRECTION('',(-0.707106781186561,0.707106781186534,0.));
#32284=DIRECTION('',(0.,1.,0.));
#32285=DIRECTION('',(0.707106781186546,0.707106781186549,0.));
#32286=DIRECTION('',(1.,0.,0.));
#32287=DIRECTION('center_axis',(-0.707106781186549,-0.707106781186546,0.));
#32288=DIRECTION('ref_axis',(0.707106781186546,-0.707106781186549,0.));
#32289=DIRECTION('',(0.707106781186546,-0.707106781186549,0.));
#32290=DIRECTION('',(0.,0.,1.));
#32291=DIRECTION('',(0.,0.,1.));
#32292=DIRECTION('center_axis',(0.,0.,1.));
#32293=DIRECTION('ref_axis',(1.,0.,0.));
#32294=DIRECTION('center_axis',(0.,0.,1.));
#32295=DIRECTION('ref_axis',(1.,0.,0.));
#32296=DIRECTION('',(0.,0.,1.));
#32297=DIRECTION('center_axis',(-1.,0.,0.));
#32298=DIRECTION('ref_axis',(0.,0.,1.));
#32299=DIRECTION('',(0.,-1.,0.));
#32300=DIRECTION('',(0.,0.,1.));
#32301=DIRECTION('center_axis',(0.,0.,1.));
#32302=DIRECTION('ref_axis',(1.,0.,0.));
#32303=DIRECTION('center_axis',(0.,0.,1.));
#32304=DIRECTION('ref_axis',(1.,0.,0.));
#32305=DIRECTION('',(0.,0.,1.));
#32306=DIRECTION('center_axis',(-0.707106781186543,0.707106781186552,0.));
#32307=DIRECTION('ref_axis',(-0.707106781186552,-0.707106781186543,0.));
#32308=DIRECTION('',(-0.707106781186552,-0.707106781186543,0.));
#32309=DIRECTION('',(0.,0.,1.));
#32310=DIRECTION('center_axis',(0.,0.,1.));
#32311=DIRECTION('ref_axis',(1.,0.,0.));
#32312=DIRECTION('center_axis',(0.,0.,-1.));
#32313=DIRECTION('ref_axis',(1.,0.,0.));
#32314=DIRECTION('',(0.,0.,1.));
#32315=DIRECTION('center_axis',(0.,0.,1.));
#32316=DIRECTION('ref_axis',(1.,0.,0.));
#32317=DIRECTION('center_axis',(0.,0.,1.));
#32318=DIRECTION('ref_axis',(1.,0.,0.));
#32319=DIRECTION('',(0.,0.,1.));
#32320=DIRECTION('center_axis',(0.,0.,1.));
#32321=DIRECTION('ref_axis',(1.,0.,0.));
#32322=DIRECTION('center_axis',(0.,0.,-1.));
#32323=DIRECTION('ref_axis',(1.,0.,0.));
#32324=DIRECTION('',(0.,0.,1.));
#32325=DIRECTION('center_axis',(-0.707106781186543,0.707106781186552,0.));
#32326=DIRECTION('ref_axis',(-0.707106781186552,-0.707106781186543,0.));
#32327=DIRECTION('',(-0.707106781186552,-0.707106781186543,0.));
#32328=DIRECTION('',(0.,0.,1.));
#32329=DIRECTION('center_axis',(0.,0.,1.));
#32330=DIRECTION('ref_axis',(1.,0.,0.));
#32331=DIRECTION('center_axis',(0.,0.,-1.));
#32332=DIRECTION('ref_axis',(1.,0.,0.));
#32333=DIRECTION('',(0.,0.,1.));
#32334=DIRECTION('center_axis',(-1.,0.,0.));
#32335=DIRECTION('ref_axis',(0.,0.,1.));
#32336=DIRECTION('',(0.,-1.,0.));
#32337=DIRECTION('',(0.,0.,1.));
#32338=DIRECTION('center_axis',(0.,0.,1.));
#32339=DIRECTION('ref_axis',(1.,0.,0.));
#32340=DIRECTION('center_axis',(0.,0.,-1.));
#32341=DIRECTION('ref_axis',(1.,0.,0.));
#32342=DIRECTION('',(0.,0.,1.));
#32343=DIRECTION('center_axis',(-0.707106781186548,-0.707106781186548,0.));
#32344=DIRECTION('ref_axis',(0.707106781186548,-0.707106781186548,0.));
#32345=DIRECTION('',(0.707106781186547,-0.707106781186547,0.));
#32346=DIRECTION('',(0.,0.,1.));
#32347=DIRECTION('center_axis',(0.,0.,1.));
#32348=DIRECTION('ref_axis',(1.,0.,0.));
#32349=DIRECTION('center_axis',(0.,0.,-1.));
#32350=DIRECTION('ref_axis',(1.,0.,0.));
#32351=DIRECTION('',(0.,0.,1.));
#32352=DIRECTION('center_axis',(0.,0.,1.));
#32353=DIRECTION('ref_axis',(1.,0.,0.));
#32354=DIRECTION('center_axis',(0.,0.,1.));
#32355=DIRECTION('ref_axis',(1.,0.,0.));
#32356=DIRECTION('',(0.,0.,1.));
#32357=DIRECTION('center_axis',(0.,0.,1.));
#32358=DIRECTION('ref_axis',(1.,0.,0.));
#32359=DIRECTION('center_axis',(0.,0.,-1.));
#32360=DIRECTION('ref_axis',(1.,0.,0.));
#32361=DIRECTION('',(0.,0.,1.));
#32362=DIRECTION('center_axis',(-0.707106781186549,-0.707106781186546,0.));
#32363=DIRECTION('ref_axis',(0.707106781186546,-0.707106781186549,0.));
#32364=DIRECTION('',(0.707106781186546,-0.707106781186549,0.));
#32365=DIRECTION('',(0.,0.,1.));
#32366=DIRECTION('center_axis',(4.61786466713945E-17,-1.,0.));
#32367=DIRECTION('ref_axis',(1.,4.61786466713945E-17,0.));
#32368=DIRECTION('',(1.,4.61786466713945E-17,0.));
#32369=DIRECTION('',(0.,0.,1.));
#32370=DIRECTION('center_axis',(0.707106781186548,-0.707106781186547,0.));
#32371=DIRECTION('ref_axis',(0.707106781186547,0.707106781186548,0.));
#32372=DIRECTION('',(0.707106781186547,0.707106781186548,0.));
#32373=DIRECTION('',(0.,0.,1.));
#32374=DIRECTION('center_axis',(0.,0.,1.));
#32375=DIRECTION('ref_axis',(1.,0.,0.));
#32376=DIRECTION('center_axis',(0.,0.,-1.));
#32377=DIRECTION('ref_axis',(1.,0.,0.));
#32378=DIRECTION('',(0.,0.,1.));
#32379=DIRECTION('center_axis',(0.,0.,1.));
#32380=DIRECTION('ref_axis',(1.,0.,0.));
#32381=DIRECTION('center_axis',(0.,0.,1.));
#32382=DIRECTION('ref_axis',(1.,0.,0.));
#32383=DIRECTION('',(0.,0.,1.));
#32384=DIRECTION('center_axis',(0.,0.,1.));
#32385=DIRECTION('ref_axis',(1.,0.,0.));
#32386=DIRECTION('center_axis',(0.,0.,-1.));
#32387=DIRECTION('ref_axis',(1.,0.,0.));
#32388=DIRECTION('',(0.,0.,1.));
#32389=DIRECTION('center_axis',(0.70710678118655,-0.707106781186545,0.));
#32390=DIRECTION('ref_axis',(0.707106781186545,0.70710678118655,0.));
#32391=DIRECTION('',(0.707106781186546,0.707106781186549,0.));
#32392=DIRECTION('',(0.,0.,1.));
#32393=DIRECTION('center_axis',(0.,0.,1.));
#32394=DIRECTION('ref_axis',(1.,0.,0.));
#32395=DIRECTION('center_axis',(0.,0.,-1.));
#32396=DIRECTION('ref_axis',(1.,0.,0.));
#32397=DIRECTION('',(0.,0.,1.));
#32398=DIRECTION('center_axis',(1.,0.,0.));
#32399=DIRECTION('ref_axis',(0.,0.,-1.));
#32400=DIRECTION('',(0.,1.,0.));
#32401=DIRECTION('',(0.,0.,1.));
#32402=DIRECTION('center_axis',(0.,0.,1.));
#32403=DIRECTION('ref_axis',(1.,0.,0.));
#32404=DIRECTION('center_axis',(0.,0.,-1.));
#32405=DIRECTION('ref_axis',(1.,0.,0.));
#32406=DIRECTION('',(0.,0.,1.));
#32407=DIRECTION('center_axis',(0.707106781186549,0.707106781186546,0.));
#32408=DIRECTION('ref_axis',(-0.707106781186546,0.707106781186549,0.));
#32409=DIRECTION('',(-0.707106781186546,0.707106781186549,0.));
#32410=DIRECTION('',(0.,0.,1.));
#32411=DIRECTION('center_axis',(0.,0.,1.));
#32412=DIRECTION('ref_axis',(1.,0.,0.));
#32413=DIRECTION('center_axis',(0.,0.,-1.));
#32414=DIRECTION('ref_axis',(1.,0.,0.));
#32415=DIRECTION('',(0.,0.,1.));
#32416=DIRECTION('center_axis',(0.,0.,1.));
#32417=DIRECTION('ref_axis',(1.,0.,0.));
#32418=DIRECTION('center_axis',(0.,0.,1.));
#32419=DIRECTION('ref_axis',(1.,0.,0.));
#32420=DIRECTION('',(0.,0.,1.));
#32421=DIRECTION('center_axis',(0.,0.,1.));
#32422=DIRECTION('ref_axis',(1.,0.,0.));
#32423=DIRECTION('center_axis',(0.,0.,-1.));
#32424=DIRECTION('ref_axis',(1.,0.,0.));
#32425=DIRECTION('',(0.,0.,1.));
#32426=DIRECTION('center_axis',(0.707106781186543,0.707106781186552,0.));
#32427=DIRECTION('ref_axis',(-0.707106781186553,0.707106781186543,0.));
#32428=DIRECTION('',(-0.707106781186552,0.707106781186543,0.));
#32429=DIRECTION('',(0.,0.,1.));
#32430=DIRECTION('center_axis',(0.,0.,1.));
#32431=DIRECTION('ref_axis',(1.,0.,0.));
#32432=DIRECTION('center_axis',(0.,0.,1.));
#32433=DIRECTION('ref_axis',(1.,0.,0.));
#32434=DIRECTION('',(0.,0.,1.));
#32435=DIRECTION('center_axis',(1.,0.,0.));
#32436=DIRECTION('ref_axis',(0.,0.,-1.));
#32437=DIRECTION('',(0.,1.,0.));
#32438=DIRECTION('',(0.,0.,1.));
#32439=DIRECTION('center_axis',(0.,0.,1.));
#32440=DIRECTION('ref_axis',(1.,0.,0.));
#32441=DIRECTION('center_axis',(0.,0.,1.));
#32442=DIRECTION('ref_axis',(1.,0.,0.));
#32443=DIRECTION('',(0.,0.,1.));
#32444=DIRECTION('center_axis',(0.707106781186549,-0.707106781186546,0.));
#32445=DIRECTION('ref_axis',(0.707106781186546,0.707106781186549,0.));
#32446=DIRECTION('',(0.707106781186546,0.707106781186549,0.));
#32447=DIRECTION('',(0.,0.,1.));
#32448=DIRECTION('center_axis',(0.,-1.,0.));
#32449=DIRECTION('ref_axis',(0.,0.,-1.));
#32450=DIRECTION('',(1.,0.,0.));
#32451=DIRECTION('',(0.,0.,1.));
#32452=DIRECTION('center_axis',(-0.707106781186548,-0.707106781186547,0.));
#32453=DIRECTION('ref_axis',(0.707106781186547,-0.707106781186548,0.));
#32454=DIRECTION('',(0.707106781186547,-0.707106781186548,0.));
#32455=DIRECTION('',(0.,0.,1.));
#32456=DIRECTION('center_axis',(-1.,-1.26352022694434E-16,0.));
#32457=DIRECTION('ref_axis',(1.26352022694434E-16,-1.,0.));
#32458=DIRECTION('',(1.26352022694434E-16,-1.,0.));
#32459=DIRECTION('',(0.,0.,1.));
#32460=DIRECTION('center_axis',(-0.707106781186533,0.707106781186562,0.));
#32461=DIRECTION('ref_axis',(-0.707106781186562,-0.707106781186533,0.));
#32462=DIRECTION('',(-0.707106781186562,-0.707106781186533,0.));
#32463=DIRECTION('',(0.,0.,1.));
#32464=DIRECTION('center_axis',(-1.95534159233113E-16,1.,0.));
#32465=DIRECTION('ref_axis',(-1.,-1.95534159233113E-16,0.));
#32466=DIRECTION('',(-1.,-1.95534159233113E-16,0.));
#32467=DIRECTION('',(0.,0.,1.));
#32468=DIRECTION('center_axis',(0.707106781186534,0.707106781186561,0.));
#32469=DIRECTION('ref_axis',(-0.707106781186561,0.707106781186534,0.));
#32470=DIRECTION('',(-0.707106781186561,0.707106781186534,0.));
#32471=DIRECTION('',(0.,0.,1.));
#32472=DIRECTION('center_axis',(1.,0.,0.));
#32473=DIRECTION('ref_axis',(0.,0.,-1.));
#32474=DIRECTION('',(0.,1.,0.));
#32475=DIRECTION('',(0.,0.,1.));
#32476=DIRECTION('center_axis',(0.707106781186549,-0.707106781186546,0.));
#32477=DIRECTION('ref_axis',(0.707106781186546,0.707106781186549,0.));
#32478=DIRECTION('',(0.707106781186546,0.707106781186549,0.));
#32479=DIRECTION('',(0.,0.,1.));
#32480=DIRECTION('center_axis',(0.,-1.,0.));
#32481=DIRECTION('ref_axis',(0.,0.,-1.));
#32482=DIRECTION('',(1.,0.,0.));
#32483=DIRECTION('center_axis',(-1.30104260698261E-15,1.,-1.73611473352215E-31));
#32484=DIRECTION('ref_axis',(-1.,-1.30104260698261E-15,0.));
#32485=DIRECTION('center_axis',(-1.30104260698261E-15,1.,-1.73611473352215E-31));
#32486=DIRECTION('ref_axis',(-1.,-1.30104260698261E-15,0.));
#32487=DIRECTION('',(4.33680868994202E-17,0.,1.));
#32488=DIRECTION('center_axis',(-1.30104260698261E-15,1.,-1.73611473352215E-31));
#32489=DIRECTION('ref_axis',(-1.,-1.30104260698261E-15,2.25875923892257E-46));
#32490=DIRECTION('',(4.33680868994202E-17,0.,-1.));
#32491=DIRECTION('center_axis',(0.,0.,-1.));
#32492=DIRECTION('ref_axis',(-1.,0.,0.));
#32493=DIRECTION('',(1.,0.,0.));
#32494=DIRECTION('',(-1.73472347597681E-16,1.,0.));
#32495=DIRECTION('center_axis',(0.,0.,1.));
#32496=DIRECTION('ref_axis',(1.,0.,0.));
#32497=DIRECTION('',(-1.73472347597681E-16,-1.,0.));
#32498=DIRECTION('',(1.,0.,0.));
#32499=DIRECTION('',(0.707106781186562,0.707106781186533,0.));
#32500=DIRECTION('',(-1.26161707343768E-16,1.,0.));
#32501=DIRECTION('',(-0.707106781186547,0.707106781186548,0.));
#32502=DIRECTION('',(1.,0.,0.));
#32503=DIRECTION('',(0.707106781186546,0.707106781186549,0.));
#32504=DIRECTION('center_axis',(0.,0.,1.));
#32505=DIRECTION('ref_axis',(-1.,0.,0.));
#32506=DIRECTION('',(0.,1.,0.));
#32507=DIRECTION('center_axis',(0.,0.,1.));
#32508=DIRECTION('ref_axis',(-1.,0.,0.));
#32509=DIRECTION('',(-0.707106781186549,0.707106781186546,0.));
#32510=DIRECTION('center_axis',(0.,0.,-1.));
#32511=DIRECTION('ref_axis',(-1.,0.,0.));
#32512=DIRECTION('center_axis',(0.,0.,1.));
#32513=DIRECTION('ref_axis',(1.,0.,0.));
#32514=DIRECTION('center_axis',(0.,0.,-1.));
#32515=DIRECTION('ref_axis',(-1.,0.,0.));
#32516=DIRECTION('',(-0.707106781186549,0.707106781186546,0.));
#32517=DIRECTION('center_axis',(0.,0.,-1.));
#32518=DIRECTION('ref_axis',(-1.,0.,0.));
#32519=DIRECTION('',(0.,1.,0.));
#32520=DIRECTION('center_axis',(0.,0.,-1.));
#32521=DIRECTION('ref_axis',(-1.,0.,0.));
#32522=DIRECTION('',(0.707106781186546,0.707106781186549,0.));
#32523=DIRECTION('center_axis',(0.,0.,-1.));
#32524=DIRECTION('ref_axis',(-1.,0.,0.));
#32525=DIRECTION('center_axis',(0.,0.,1.));
#32526=DIRECTION('ref_axis',(1.,0.,0.));
#32527=DIRECTION('center_axis',(0.,0.,-1.));
#32528=DIRECTION('ref_axis',(-1.,0.,0.));
#32529=DIRECTION('',(0.707106781186546,0.707106781186549,0.));
#32530=DIRECTION('',(1.,1.22464679914735E-16,0.));
#32531=DIRECTION('',(0.707106781186546,-0.707106781186549,0.));
#32532=DIRECTION('center_axis',(0.,0.,-1.));
#32533=DIRECTION('ref_axis',(-1.,0.,0.));
#32534=DIRECTION('center_axis',(0.,0.,1.));
#32535=DIRECTION('ref_axis',(1.,0.,0.));
#32536=DIRECTION('center_axis',(0.,0.,-1.));
#32537=DIRECTION('ref_axis',(-1.,0.,0.));
#32538=DIRECTION('',(0.707106781186546,-0.707106781186549,0.));
#32539=DIRECTION('center_axis',(0.,0.,-1.));
#32540=DIRECTION('ref_axis',(-1.,0.,0.));
#32541=DIRECTION('',(0.,-1.,0.));
#32542=DIRECTION('center_axis',(0.,0.,-1.));
#32543=DIRECTION('ref_axis',(-1.,0.,0.));
#32544=DIRECTION('',(-0.707106781186549,-0.707106781186546,0.));
#32545=DIRECTION('center_axis',(0.,0.,-1.));
#32546=DIRECTION('ref_axis',(-1.,0.,0.));
#32547=DIRECTION('center_axis',(0.,0.,1.));
#32548=DIRECTION('ref_axis',(1.,0.,0.));
#32549=DIRECTION('center_axis',(0.,0.,-1.));
#32550=DIRECTION('ref_axis',(-1.,0.,0.));
#32551=DIRECTION('',(-0.707106781186549,-0.707106781186546,0.));
#32552=DIRECTION('center_axis',(0.,0.,1.));
#32553=DIRECTION('ref_axis',(-1.,-3.46944695195361E-15,0.));
#32554=DIRECTION('',(0.,-1.,0.));
#32555=DIRECTION('center_axis',(0.,0.,1.));
#32556=DIRECTION('ref_axis',(-1.,0.,0.));
#32557=DIRECTION('',(0.707106781186546,-0.707106781186549,0.));
#32558=DIRECTION('',(1.,-6.49101394191508E-16,0.));
#32559=DIRECTION('',(-0.707106781186547,-0.707106781186548,0.));
#32560=DIRECTION('',(-1.26161707343768E-16,-1.,0.));
#32561=DIRECTION('',(0.707106781186562,-0.707106781186533,0.));
#32562=DIRECTION('center_axis',(1.,1.30104260698261E-15,4.33680868994202E-17));
#32563=DIRECTION('ref_axis',(-1.30104260698261E-15,1.,5.08894400801554E-48));
#32564=DIRECTION('',(4.33680868994202E-17,0.,-1.));
#32565=DIRECTION('',(-1.30104260698261E-15,1.,-1.73611473352215E-31));
#32566=DIRECTION('center_axis',(-1.,-1.30104260698261E-15,4.33680868994202E-17));
#32567=DIRECTION('ref_axis',(1.30104260698261E-15,-1.,5.08894400801554E-48));
#32568=DIRECTION('',(4.33680868994202E-17,0.,1.));
#32569=DIRECTION('',(-1.30104260698261E-15,1.,-1.73611473352215E-31));
#32570=DIRECTION('center_axis',(-1.30104260698261E-15,1.,-1.73611473352215E-31));
#32571=DIRECTION('ref_axis',(-1.,-1.30104260698261E-15,2.25875923892257E-46));
#32572=DIRECTION('center_axis',(-1.30104260698261E-15,1.,-1.73611473352215E-31));
#32573=DIRECTION('ref_axis',(-1.,-1.30104260698261E-15,2.25875923892257E-46));
#32574=DIRECTION('center_axis',(-1.30104260698261E-15,1.,-1.73611473352215E-31));
#32575=DIRECTION('ref_axis',(-1.,-1.30104260698261E-15,0.));
#32576=DIRECTION('center_axis',(-1.30104260698261E-15,1.,-1.73611473352215E-31));
#32577=DIRECTION('ref_axis',(-1.,-1.30104260698261E-15,0.));
#32578=DIRECTION('',(-1.3010426069826E-16,0.,-1.));
#32579=DIRECTION('center_axis',(-1.30104260698261E-15,1.,-1.73611473352215E-31));
#32580=DIRECTION('ref_axis',(-1.,-1.30104260698261E-15,2.25875923892257E-46));
#32581=DIRECTION('',(1.3010426069826E-16,0.,1.));
#32582=DIRECTION('center_axis',(-6.49101394191508E-16,-1.,0.));
#32583=DIRECTION('ref_axis',(1.,-6.49101394191508E-16,0.));
#32584=DIRECTION('',(1.,-3.50803534070133E-16,0.));
#32585=DIRECTION('',(0.,0.,1.));
#32586=DIRECTION('',(0.,0.,1.));
#32587=DIRECTION('center_axis',(-0.707106781186548,0.707106781186547,0.));
#32588=DIRECTION('ref_axis',(-0.707106781186547,-0.707106781186548,0.));
#32589=DIRECTION('',(0.707106781186547,0.707106781186548,0.));
#32590=DIRECTION('',(0.,0.,1.));
#32591=DIRECTION('center_axis',(-1.,1.26161707343768E-16,0.));
#32592=DIRECTION('ref_axis',(-1.26161707343768E-16,-1.,0.));
#32593=DIRECTION('',(1.26161707343768E-16,1.,0.));
#32594=DIRECTION('',(0.,0.,1.));
#32595=DIRECTION('center_axis',(-0.707106781186533,-0.707106781186562,0.));
#32596=DIRECTION('ref_axis',(0.707106781186562,-0.707106781186533,0.));
#32597=DIRECTION('',(-0.707106781186562,0.707106781186533,0.));
#32598=DIRECTION('',(0.,0.,1.));
#32599=DIRECTION('center_axis',(0.,-1.,0.));
#32600=DIRECTION('ref_axis',(0.,0.,-1.));
#32601=DIRECTION('',(-1.,0.,0.));
#32602=DIRECTION('',(0.,0.,1.));
#32603=DIRECTION('',(-1.,0.,0.));
#32604=DIRECTION('',(0.,0.,1.));
#32605=DIRECTION('',(0.,0.,1.));
#32606=DIRECTION('center_axis',(0.707106781186533,-0.707106781186562,0.));
#32607=DIRECTION('ref_axis',(0.707106781186562,0.707106781186533,0.));
#32608=DIRECTION('',(-0.707106781186562,-0.707106781186533,0.));
#32609=DIRECTION('',(0.,0.,1.));
#32610=DIRECTION('center_axis',(1.,1.26161707343768E-16,0.));
#32611=DIRECTION('ref_axis',(-1.26161707343768E-16,1.,0.));
#32612=DIRECTION('',(1.26161707343768E-16,-1.,0.));
#32613=DIRECTION('',(0.,0.,1.));
#32614=DIRECTION('center_axis',(0.707106781186548,0.707106781186547,0.));
#32615=DIRECTION('ref_axis',(-0.707106781186547,0.707106781186548,0.));
#32616=DIRECTION('',(0.707106781186547,-0.707106781186548,0.));
#32617=DIRECTION('',(0.,0.,1.));
#32618=DIRECTION('center_axis',(0.,-1.,0.));
#32619=DIRECTION('ref_axis',(0.,0.,-1.));
#32620=DIRECTION('',(1.,0.,0.));
#32621=DIRECTION('',(0.,0.,1.));
#32622=DIRECTION('center_axis',(0.707106781186549,-0.707106781186546,0.));
#32623=DIRECTION('ref_axis',(0.707106781186546,0.707106781186549,0.));
#32624=DIRECTION('',(0.707106781186546,0.707106781186549,0.));
#32625=DIRECTION('',(0.,0.,1.));
#32626=DIRECTION('center_axis',(0.,0.,1.));
#32627=DIRECTION('ref_axis',(1.,0.,0.));
#32628=DIRECTION('center_axis',(0.,0.,1.));
#32629=DIRECTION('ref_axis',(1.,0.,0.));
#32630=DIRECTION('',(0.,0.,-1.));
#32631=DIRECTION('center_axis',(1.,0.,0.));
#32632=DIRECTION('ref_axis',(0.,0.,-1.));
#32633=DIRECTION('',(0.,1.,0.));
#32634=DIRECTION('',(0.,0.,1.));
#32635=DIRECTION('center_axis',(0.,0.,1.));
#32636=DIRECTION('ref_axis',(1.,0.,0.));
#32637=DIRECTION('center_axis',(0.,0.,1.));
#32638=DIRECTION('ref_axis',(1.,0.,0.));
#32639=DIRECTION('',(0.,0.,-1.));
#32640=DIRECTION('center_axis',(0.707106781186546,0.707106781186549,0.));
#32641=DIRECTION('ref_axis',(-0.707106781186549,0.707106781186546,0.));
#32642=DIRECTION('',(-0.707106781186549,0.707106781186546,0.));
#32643=DIRECTION('',(0.,0.,1.));
#32644=DIRECTION('center_axis',(0.,0.,1.));
#32645=DIRECTION('ref_axis',(1.,0.,0.));
#32646=DIRECTION('center_axis',(0.,0.,-1.));
#32647=DIRECTION('ref_axis',(1.,0.,0.));
#32648=DIRECTION('',(0.,0.,-1.));
#32649=DIRECTION('center_axis',(0.,0.,1.));
#32650=DIRECTION('ref_axis',(1.,0.,0.));
#32651=DIRECTION('center_axis',(0.,0.,1.));
#32652=DIRECTION('ref_axis',(1.,0.,0.));
#32653=DIRECTION('',(0.,0.,1.));
#32654=DIRECTION('center_axis',(0.,0.,1.));
#32655=DIRECTION('ref_axis',(1.,0.,0.));
#32656=DIRECTION('center_axis',(0.,0.,-1.));
#32657=DIRECTION('ref_axis',(1.,0.,0.));
#32658=DIRECTION('',(0.,0.,-1.));
#32659=DIRECTION('center_axis',(0.707106781186546,0.707106781186549,0.));
#32660=DIRECTION('ref_axis',(-0.707106781186549,0.707106781186546,0.));
#32661=DIRECTION('',(-0.707106781186548,0.707106781186547,0.));
#32662=DIRECTION('',(0.,0.,1.));
#32663=DIRECTION('center_axis',(0.,0.,-1.));
#32664=DIRECTION('ref_axis',(-1.,0.,0.));
#32665=DIRECTION('center_axis',(0.,0.,-1.));
#32666=DIRECTION('ref_axis',(1.,0.,0.));
#32667=DIRECTION('',(0.,0.,-1.));
#32668=DIRECTION('center_axis',(1.,0.,0.));
#32669=DIRECTION('ref_axis',(0.,0.,-1.));
#32670=DIRECTION('',(0.,1.,0.));
#32671=DIRECTION('',(0.,0.,1.));
#32672=DIRECTION('center_axis',(0.,0.,-1.));
#32673=DIRECTION('ref_axis',(-1.,0.,0.));
#32674=DIRECTION('center_axis',(0.,0.,-1.));
#32675=DIRECTION('ref_axis',(1.,0.,0.));
#32676=DIRECTION('',(0.,0.,-1.));
#32677=DIRECTION('center_axis',(0.707106781186549,-0.707106781186546,0.));
#32678=DIRECTION('ref_axis',(0.707106781186546,0.707106781186549,0.));
#32679=DIRECTION('',(0.707106781186545,0.70710678118655,0.));
#32680=DIRECTION('',(0.,0.,1.));
#32681=DIRECTION('center_axis',(0.,0.,1.));
#32682=DIRECTION('ref_axis',(1.,0.,0.));
#32683=DIRECTION('center_axis',(0.,0.,-1.));
#32684=DIRECTION('ref_axis',(1.,0.,0.));
#32685=DIRECTION('',(0.,0.,-1.));
#32686=DIRECTION('center_axis',(0.,0.,1.));
#32687=DIRECTION('ref_axis',(1.,0.,0.));
#32688=DIRECTION('center_axis',(0.,0.,1.));
#32689=DIRECTION('ref_axis',(1.,0.,0.));
#32690=DIRECTION('',(0.,0.,1.));
#32691=DIRECTION('center_axis',(0.,0.,1.));
#32692=DIRECTION('ref_axis',(1.,0.,0.));
#32693=DIRECTION('center_axis',(0.,0.,-1.));
#32694=DIRECTION('ref_axis',(1.,0.,0.));
#32695=DIRECTION('',(0.,0.,-1.));
#32696=DIRECTION('center_axis',(0.707106781186549,-0.707106781186546,0.));
#32697=DIRECTION('ref_axis',(0.707106781186546,0.707106781186549,0.));
#32698=DIRECTION('',(0.707106781186546,0.707106781186549,0.));
#32699=DIRECTION('',(0.,0.,1.));
#32700=DIRECTION('center_axis',(1.22464679914735E-16,-1.,0.));
#32701=DIRECTION('ref_axis',(1.,1.22464679914735E-16,0.));
#32702=DIRECTION('',(1.,1.22464679914735E-16,0.));
#32703=DIRECTION('',(0.,0.,1.));
#32704=DIRECTION('center_axis',(-0.707106781186549,-0.707106781186546,0.));
#32705=DIRECTION('ref_axis',(0.707106781186546,-0.707106781186549,0.));
#32706=DIRECTION('',(0.707106781186546,-0.707106781186549,0.));
#32707=DIRECTION('',(0.,0.,1.));
#32708=DIRECTION('center_axis',(0.,0.,1.));
#32709=DIRECTION('ref_axis',(1.,0.,0.));
#32710=DIRECTION('center_axis',(0.,0.,-1.));
#32711=DIRECTION('ref_axis',(1.,0.,0.));
#32712=DIRECTION('',(0.,0.,-1.));
#32713=DIRECTION('center_axis',(0.,0.,1.));
#32714=DIRECTION('ref_axis',(1.,0.,0.));
#32715=DIRECTION('center_axis',(0.,0.,1.));
#32716=DIRECTION('ref_axis',(1.,0.,0.));
#32717=DIRECTION('',(0.,0.,1.));
#32718=DIRECTION('center_axis',(0.,0.,1.));
#32719=DIRECTION('ref_axis',(1.,0.,0.));
#32720=DIRECTION('center_axis',(0.,0.,-1.));
#32721=DIRECTION('ref_axis',(1.,0.,0.));
#32722=DIRECTION('',(0.,0.,-1.));
#32723=DIRECTION('center_axis',(-0.707106781186549,-0.707106781186546,0.));
#32724=DIRECTION('ref_axis',(0.707106781186546,-0.707106781186549,0.));
#32725=DIRECTION('',(0.707106781186545,-0.70710678118655,0.));
#32726=DIRECTION('',(0.,0.,1.));
#32727=DIRECTION('center_axis',(0.,0.,-1.));
#32728=DIRECTION('ref_axis',(-1.,0.,0.));
#32729=DIRECTION('center_axis',(0.,0.,-1.));
#32730=DIRECTION('ref_axis',(1.,0.,0.));
#32731=DIRECTION('',(0.,0.,-1.));
#32732=DIRECTION('center_axis',(-1.,0.,0.));
#32733=DIRECTION('ref_axis',(0.,0.,1.));
#32734=DIRECTION('',(0.,-1.,0.));
#32735=DIRECTION('',(0.,0.,1.));
#32736=DIRECTION('center_axis',(0.,0.,-1.));
#32737=DIRECTION('ref_axis',(-1.,0.,0.));
#32738=DIRECTION('center_axis',(0.,0.,-1.));
#32739=DIRECTION('ref_axis',(1.,0.,0.));
#32740=DIRECTION('',(0.,0.,-1.));
#32741=DIRECTION('center_axis',(-0.707106781186546,0.707106781186549,0.));
#32742=DIRECTION('ref_axis',(-0.707106781186549,-0.707106781186546,0.));
#32743=DIRECTION('',(-0.707106781186548,-0.707106781186547,0.));
#32744=DIRECTION('',(0.,0.,1.));
#32745=DIRECTION('center_axis',(0.,0.,1.));
#32746=DIRECTION('ref_axis',(1.,0.,0.));
#32747=DIRECTION('center_axis',(0.,0.,-1.));
#32748=DIRECTION('ref_axis',(1.,0.,0.));
#32749=DIRECTION('',(0.,0.,-1.));
#32750=DIRECTION('center_axis',(0.,0.,1.));
#32751=DIRECTION('ref_axis',(1.,0.,0.));
#32752=DIRECTION('center_axis',(0.,0.,1.));
#32753=DIRECTION('ref_axis',(1.,0.,0.));
#32754=DIRECTION('',(0.,0.,1.));
#32755=DIRECTION('center_axis',(0.,0.,1.));
#32756=DIRECTION('ref_axis',(1.,0.,0.));
#32757=DIRECTION('center_axis',(0.,0.,-1.));
#32758=DIRECTION('ref_axis',(1.,0.,0.));
#32759=DIRECTION('',(0.,0.,-1.));
#32760=DIRECTION('center_axis',(-0.707106781186546,0.707106781186549,0.));
#32761=DIRECTION('ref_axis',(-0.707106781186549,-0.707106781186546,0.));
#32762=DIRECTION('',(-0.707106781186549,-0.707106781186546,0.));
#32763=DIRECTION('',(0.,0.,1.));
#32764=DIRECTION('center_axis',(0.,0.,1.));
#32765=DIRECTION('ref_axis',(1.,0.,0.));
#32766=DIRECTION('center_axis',(0.,0.,1.));
#32767=DIRECTION('ref_axis',(1.,0.,0.));
#32768=DIRECTION('',(0.,0.,-1.));
#32769=DIRECTION('center_axis',(-1.,0.,0.));
#32770=DIRECTION('ref_axis',(0.,0.,1.));
#32771=DIRECTION('',(0.,-1.,0.));
#32772=DIRECTION('',(0.,0.,1.));
#32773=DIRECTION('center_axis',(0.,0.,1.));
#32774=DIRECTION('ref_axis',(1.,0.,0.));
#32775=DIRECTION('center_axis',(0.,0.,1.));
#32776=DIRECTION('ref_axis',(1.,0.,0.));
#32777=DIRECTION('',(0.,0.,-1.));
#32778=DIRECTION('center_axis',(-0.707106781186549,-0.707106781186546,0.));
#32779=DIRECTION('ref_axis',(0.707106781186546,-0.707106781186549,0.));
#32780=DIRECTION('',(0.707106781186546,-0.707106781186549,0.));
#32781=DIRECTION('center_axis',(-1.30104260698261E-15,1.,-1.73611473352215E-31));
#32782=DIRECTION('ref_axis',(-1.,-1.30104260698261E-15,0.));
#32783=DIRECTION('center_axis',(-7.96355992932556E-18,-1.,0.));
#32784=DIRECTION('ref_axis',(1.,-7.96355992932556E-18,0.));
#32785=DIRECTION('',(0.,0.,1.));
#32786=DIRECTION('',(-1.,7.96355992932556E-18,0.));
#32787=DIRECTION('',(0.,0.,-1.));
#32788=DIRECTION('',(1.,-7.96355992932556E-18,0.));
#32789=DIRECTION('center_axis',(4.11015771401436E-16,-1.,0.));
#32790=DIRECTION('ref_axis',(1.,4.11015771401436E-16,0.));
#32791=DIRECTION('',(0.,0.,1.));
#32792=DIRECTION('',(-1.,-4.11015771401436E-16,0.));
#32793=DIRECTION('',(0.,0.,-1.));
#32794=DIRECTION('',(-1.,-4.11015771401436E-16,0.));
#32795=DIRECTION('center_axis',(-1.,-1.30104260698261E-15,1.3010426069826E-16));
#32796=DIRECTION('ref_axis',(1.30104260698261E-15,-1.,-3.07902494602621E-48));
#32797=DIRECTION('',(1.3010426069826E-16,0.,1.));
#32798=DIRECTION('',(-1.30104260698261E-15,1.,-1.73611473352215E-31));
#32799=DIRECTION('center_axis',(1.,1.30104260698261E-15,-1.3010426069826E-16));
#32800=DIRECTION('ref_axis',(-1.30104260698261E-15,1.,3.07902494602621E-48));
#32801=DIRECTION('',(-1.3010426069826E-16,0.,-1.));
#32802=DIRECTION('',(-1.30104260698261E-15,1.,-1.73611473352215E-31));
#32803=DIRECTION('center_axis',(-1.30104260698261E-15,1.,-1.73611473352215E-31));
#32804=DIRECTION('ref_axis',(-1.,-1.30104260698261E-15,2.25875923892257E-46));
#32805=DIRECTION('center_axis',(-1.30104260698261E-15,1.,-1.73611473352215E-31));
#32806=DIRECTION('ref_axis',(-1.,-1.30104260698261E-15,2.25875923892257E-46));
#32807=DIRECTION('center_axis',(0.,0.,-1.));
#32808=DIRECTION('ref_axis',(-1.,0.,0.));
#32809=DIRECTION('center_axis',(0.,0.,-1.));
#32810=DIRECTION('ref_axis',(1.,0.,0.));
#32811=DIRECTION('center_axis',(0.,0.,1.));
#32812=DIRECTION('ref_axis',(-1.,-1.73472347597681E-15,0.));
#32813=DIRECTION('',(0.,0.,-1.));
#32814=DIRECTION('center_axis',(0.,0.,1.));
#32815=DIRECTION('ref_axis',(1.,0.,0.));
#32816=DIRECTION('',(-0.258819045102518,0.965925826289069,0.));
#32817=DIRECTION('',(2.04085114820801E-16,1.,0.));
#32818=DIRECTION('',(-1.,1.2823896663807E-16,0.));
#32819=DIRECTION('',(-0.707106781186548,0.707106781186547,0.));
#32820=DIRECTION('center_axis',(1.,-2.04085114820801E-16,0.));
#32821=DIRECTION('ref_axis',(2.04085114820801E-16,1.,0.));
#32822=DIRECTION('',(0.,0.,1.));
#32823=DIRECTION('',(0.,1.,0.));
#32824=DIRECTION('',(0.,0.,1.));
#32825=DIRECTION('center_axis',(-1.,-2.04085114820801E-16,0.));
#32826=DIRECTION('ref_axis',(2.04085114820801E-16,-1.,0.));
#32827=DIRECTION('',(0.,0.,1.));
#32828=DIRECTION('',(0.,-1.,0.));
#32829=DIRECTION('',(0.,0.,-1.));
#32830=DIRECTION('',(2.04085114820801E-16,-1.,0.));
#32831=DIRECTION('center_axis',(0.,0.,1.));
#32832=DIRECTION('ref_axis',(1.,0.,0.));
#32833=DIRECTION('',(-0.258819045102518,-0.965925826289069,0.));
#32834=DIRECTION('center_axis',(0.,0.,-1.));
#32835=DIRECTION('ref_axis',(1.,-1.73472347597681E-15,0.));
#32836=DIRECTION('',(-0.707106781186557,-0.707106781186538,0.));
#32837=DIRECTION('',(-1.,-1.2823896663807E-16,0.));
#32838=DIRECTION('center_axis',(0.,0.,-1.));
#32839=DIRECTION('ref_axis',(-1.,0.,0.));
#32840=DIRECTION('',(0.,0.,1.));
#32841=DIRECTION('center_axis',(0.,0.,-1.));
#32842=DIRECTION('ref_axis',(1.,0.,0.));
#32843=DIRECTION('center_axis',(0.,0.,1.));
#32844=DIRECTION('ref_axis',(1.,0.,0.));
#32845=DIRECTION('',(1.,0.,0.));
#32846=DIRECTION('',(0.707106781186546,0.707106781186549,0.));
#32847=DIRECTION('',(0.,1.,0.));
#32848=DIRECTION('',(-0.707106781186561,0.707106781186534,0.));
#32849=DIRECTION('',(-1.,-1.95534159233113E-16,0.));
#32850=DIRECTION('',(-0.707106781186562,-0.707106781186533,0.));
#32851=DIRECTION('',(1.26352022694434E-16,-1.,0.));
#32852=DIRECTION('',(0.707106781186547,-0.707106781186548,0.));
#32853=DIRECTION('',(1.,0.,0.));
#32854=DIRECTION('',(0.707106781186546,0.707106781186549,0.));
#32855=DIRECTION('center_axis',(0.,0.,1.));
#32856=DIRECTION('ref_axis',(1.,0.,0.));
#32857=DIRECTION('',(0.,1.,0.));
#32858=DIRECTION('center_axis',(0.,0.,1.));
#32859=DIRECTION('ref_axis',(1.,0.,0.));
#32860=DIRECTION('',(-0.707106781186552,0.707106781186543,0.));
#32861=DIRECTION('center_axis',(0.,0.,-1.));
#32862=DIRECTION('ref_axis',(1.,0.,0.));
#32863=DIRECTION('center_axis',(0.,0.,1.));
#32864=DIRECTION('ref_axis',(1.,0.,0.));
#32865=DIRECTION('center_axis',(0.,0.,-1.));
#32866=DIRECTION('ref_axis',(1.,0.,0.));
#32867=DIRECTION('',(-0.707106781186546,0.707106781186549,0.));
#32868=DIRECTION('center_axis',(0.,0.,-1.));
#32869=DIRECTION('ref_axis',(1.,0.,0.));
#32870=DIRECTION('',(0.,1.,0.));
#32871=DIRECTION('center_axis',(0.,0.,-1.));
#32872=DIRECTION('ref_axis',(1.,0.,0.));
#32873=DIRECTION('',(0.707106781186546,0.707106781186549,0.));
#32874=DIRECTION('center_axis',(0.,0.,-1.));
#32875=DIRECTION('ref_axis',(1.,0.,0.));
#32876=DIRECTION('center_axis',(0.,0.,1.));
#32877=DIRECTION('ref_axis',(1.,0.,0.));
#32878=DIRECTION('center_axis',(0.,0.,-1.));
#32879=DIRECTION('ref_axis',(1.,0.,0.));
#32880=DIRECTION('',(0.707106781186547,0.707106781186548,0.));
#32881=DIRECTION('',(1.,4.61786466713945E-17,0.));
#32882=DIRECTION('',(0.707106781186546,-0.707106781186549,0.));
#32883=DIRECTION('center_axis',(0.,0.,-1.));
#32884=DIRECTION('ref_axis',(1.,0.,0.));
#32885=DIRECTION('center_axis',(0.,0.,1.));
#32886=DIRECTION('ref_axis',(1.,0.,0.));
#32887=DIRECTION('center_axis',(0.,0.,-1.));
#32888=DIRECTION('ref_axis',(1.,0.,0.));
#32889=DIRECTION('',(0.707106781186547,-0.707106781186547,0.));
#32890=DIRECTION('center_axis',(0.,0.,-1.));
#32891=DIRECTION('ref_axis',(1.,0.,0.));
#32892=DIRECTION('',(0.,-1.,0.));
#32893=DIRECTION('center_axis',(0.,0.,-1.));
#32894=DIRECTION('ref_axis',(1.,0.,0.));
#32895=DIRECTION('',(-0.707106781186552,-0.707106781186543,0.));
#32896=DIRECTION('center_axis',(0.,0.,-1.));
#32897=DIRECTION('ref_axis',(1.,0.,0.));
#32898=DIRECTION('center_axis',(0.,0.,1.));
#32899=DIRECTION('ref_axis',(1.,0.,0.));
#32900=DIRECTION('center_axis',(0.,0.,-1.));
#32901=DIRECTION('ref_axis',(1.,0.,0.));
#32902=DIRECTION('',(-0.707106781186552,-0.707106781186543,0.));
#32903=DIRECTION('center_axis',(0.,0.,1.));
#32904=DIRECTION('ref_axis',(1.,0.,0.));
#32905=DIRECTION('',(0.,-1.,0.));
#32906=DIRECTION('center_axis',(0.,0.,1.));
#32907=DIRECTION('ref_axis',(1.,0.,0.));
#32908=DIRECTION('',(0.707106781186546,-0.707106781186549,0.));
#32909=DIRECTION('center_axis',(-0.707106781186538,0.707106781186557,0.));
#32910=DIRECTION('ref_axis',(0.,0.,1.));
#32911=DIRECTION('',(0.,0.,-1.));
#32912=DIRECTION('',(-0.707106781186557,-0.707106781186538,0.));
#32913=DIRECTION('center_axis',(0.707106781186547,0.707106781186548,0.));
#32914=DIRECTION('ref_axis',(0.,0.,1.));
#32915=DIRECTION('',(0.,0.,1.));
#32916=DIRECTION('',(0.707106781186548,-0.707106781186547,0.));
#32917=DIRECTION('center_axis',(0.,0.,-1.));
#32918=DIRECTION('ref_axis',(-1.,0.,0.));
#32919=DIRECTION('',(-2.04085114820801E-16,-1.,0.));
#32920=DIRECTION('',(0.258819045102518,-0.965925826289069,0.));
#32921=DIRECTION('',(1.,-1.2823896663807E-16,0.));
#32922=DIRECTION('center_axis',(1.,-2.04085114820801E-16,0.));
#32923=DIRECTION('ref_axis',(2.04085114820801E-16,1.,0.));
#32924=DIRECTION('',(0.,0.,-1.));
#32925=DIRECTION('',(0.,-1.,0.));
#32926=DIRECTION('',(0.,0.,1.));
#32927=DIRECTION('center_axis',(0.,0.,1.));
#32928=DIRECTION('ref_axis',(1.,0.,0.));
#32929=DIRECTION('',(1.,1.2823896663807E-16,0.));
#32930=DIRECTION('',(-0.258819045102518,-0.965925826289069,0.));
#32931=DIRECTION('',(-2.04085114820801E-16,1.,0.));
#32932=DIRECTION('center_axis',(-1.,-2.04085114820801E-16,0.));
#32933=DIRECTION('ref_axis',(2.04085114820801E-16,-1.,0.));
#32934=DIRECTION('',(0.,0.,-1.));
#32935=DIRECTION('',(0.,1.,0.));
#32936=DIRECTION('',(0.,0.,-1.));
#32937=DIRECTION('center_axis',(-1.30104260698261E-15,1.,-1.73611473352215E-31));
#32938=DIRECTION('ref_axis',(-1.,-1.30104260698261E-15,0.));
#32939=DIRECTION('center_axis',(-0.965925826289069,-0.258819045102518,0.));
#32940=DIRECTION('ref_axis',(0.258819045102518,-0.965925826289069,0.));
#32941=DIRECTION('center_axis',(-0.965925826289069,-0.258819045102518,0.));
#32942=DIRECTION('ref_axis',(0.258819045102518,-0.965925826289069,0.));
#32943=DIRECTION('center_axis',(-0.965925826289069,-0.258819045102518,0.));
#32944=DIRECTION('ref_axis',(0.258819045102518,-0.965925826289069,0.));
#32945=DIRECTION('center_axis',(-1.2823896663807E-16,1.,0.));
#32946=DIRECTION('ref_axis',(-1.,-1.2823896663807E-16,0.));
#32947=DIRECTION('center_axis',(-1.2823896663807E-16,-1.,0.));
#32948=DIRECTION('ref_axis',(-1.,1.2823896663807E-16,0.));
#32949=DIRECTION('',(0.,0.,-1.));
#32950=DIRECTION('',(-1.,-1.2823896663807E-16,0.));
#32951=DIRECTION('',(0.,0.,1.));
#32952=DIRECTION('center_axis',(-1.,-2.04085114820801E-16,0.));
#32953=DIRECTION('ref_axis',(2.04085114820801E-16,-1.,0.));
#32954=DIRECTION('',(0.,0.,-1.));
#32955=DIRECTION('',(0.,1.,0.));
#32956=DIRECTION('',(2.04085114820801E-16,-1.,0.));
#32957=DIRECTION('center_axis',(-0.965925826289069,-0.258819045102518,0.));
#32958=DIRECTION('ref_axis',(0.258819045102518,-0.965925826289069,0.));
#32959=DIRECTION('center_axis',(-0.965925826289069,-0.258819045102518,0.));
#32960=DIRECTION('ref_axis',(0.258819045102518,-0.965925826289069,0.));
#32961=DIRECTION('',(0.258819045102518,-0.965925826289069,0.));
#32962=DIRECTION('',(0.,0.,1.));
#32963=DIRECTION('center_axis',(1.,-2.04085114820801E-16,0.));
#32964=DIRECTION('ref_axis',(2.04085114820801E-16,1.,0.));
#32965=DIRECTION('',(0.,0.,1.));
#32966=DIRECTION('',(0.,-1.,0.));
#32967=DIRECTION('',(2.04085114820801E-16,1.,0.));
#32968=DIRECTION('center_axis',(1.2823896663807E-16,1.,0.));
#32969=DIRECTION('ref_axis',(-1.,1.2823896663807E-16,0.));
#32970=DIRECTION('',(-1.,1.2823896663807E-16,0.));
#32971=DIRECTION('',(0.,0.,1.));
#32972=DIRECTION('center_axis',(-1.2823896663807E-16,-1.,0.));
#32973=DIRECTION('ref_axis',(-1.,1.2823896663807E-16,0.));
#32974=DIRECTION('center_axis',(0.965925826289069,-0.258819045102518,0.));
#32975=DIRECTION('ref_axis',(0.258819045102518,0.965925826289069,0.));
#32976=DIRECTION('center_axis',(0.965925826289069,-0.258819045102518,0.));
#32977=DIRECTION('ref_axis',(0.258819045102518,0.965925826289069,0.));
#32978=DIRECTION('',(0.258819045102518,0.965925826289069,0.));
#32979=DIRECTION('',(0.,0.,1.));
#32980=DIRECTION('center_axis',(0.965925826289069,-0.258819045102518,0.));
#32981=DIRECTION('ref_axis',(0.258819045102518,0.965925826289069,0.));
#32982=DIRECTION('center_axis',(0.965925826289069,-0.258819045102518,0.));
#32983=DIRECTION('ref_axis',(0.258819045102518,0.965925826289069,0.));
#32984=DIRECTION('center_axis',(0.965925826289069,-0.258819045102518,0.));
#32985=DIRECTION('ref_axis',(0.258819045102518,0.965925826289069,0.));
#32986=DIRECTION('center_axis',(0.,1.,0.));
#32987=DIRECTION('ref_axis',(0.,0.,1.));
#32988=DIRECTION('',(1.,0.,0.));
#32989=DIRECTION('',(0.,0.,-1.));
#32990=DIRECTION('',(0.,0.,-1.));
#32991=DIRECTION('center_axis',(-0.707106781186549,0.707106781186546,0.));
#32992=DIRECTION('ref_axis',(-0.707106781186546,-0.707106781186549,0.));
#32993=DIRECTION('',(0.707106781186546,0.707106781186549,0.));
#32994=DIRECTION('',(0.,0.,-1.));
#32995=DIRECTION('center_axis',(-1.,0.,0.));
#32996=DIRECTION('ref_axis',(0.,0.,1.));
#32997=DIRECTION('',(0.,1.,0.));
#32998=DIRECTION('',(0.,0.,-1.));
#32999=DIRECTION('center_axis',(-0.707106781186534,-0.707106781186561,0.));
#33000=DIRECTION('ref_axis',(0.707106781186561,-0.707106781186534,0.));
#33001=DIRECTION('',(-0.707106781186561,0.707106781186534,0.));
#33002=DIRECTION('',(0.,0.,-1.));
#33003=DIRECTION('center_axis',(1.95534159233113E-16,-1.,0.));
#33004=DIRECTION('ref_axis',(1.,1.95534159233113E-16,0.));
#33005=DIRECTION('',(-1.,-1.95534159233113E-16,0.));
#33006=DIRECTION('',(0.,0.,-1.));
#33007=DIRECTION('center_axis',(0.707106781186533,-0.707106781186562,0.));
#33008=DIRECTION('ref_axis',(0.707106781186562,0.707106781186533,0.));
#33009=DIRECTION('',(-0.707106781186562,-0.707106781186533,0.));
#33010=DIRECTION('',(0.,0.,-1.));
#33011=DIRECTION('center_axis',(1.,1.26352022694434E-16,0.));
#33012=DIRECTION('ref_axis',(-1.26352022694434E-16,1.,0.));
#33013=DIRECTION('',(1.26352022694434E-16,-1.,0.));
#33014=DIRECTION('',(0.,0.,-1.));
#33015=DIRECTION('center_axis',(0.707106781186548,0.707106781186547,0.));
#33016=DIRECTION('ref_axis',(-0.707106781186547,0.707106781186548,0.));
#33017=DIRECTION('',(0.707106781186547,-0.707106781186548,0.));
#33018=DIRECTION('',(0.,0.,-1.));
#33019=DIRECTION('center_axis',(0.,1.,0.));
#33020=DIRECTION('ref_axis',(0.,0.,1.));
#33021=DIRECTION('',(1.,0.,0.));
#33022=DIRECTION('',(0.,0.,-1.));
#33023=DIRECTION('center_axis',(-0.707106781186549,0.707106781186546,0.));
#33024=DIRECTION('ref_axis',(-0.707106781186546,-0.707106781186549,0.));
#33025=DIRECTION('',(0.707106781186546,0.707106781186549,0.));
#33026=DIRECTION('',(0.,0.,-1.));
#33027=DIRECTION('center_axis',(0.,0.,-1.));
#33028=DIRECTION('ref_axis',(-1.,0.,0.));
#33029=DIRECTION('center_axis',(0.,0.,1.));
#33030=DIRECTION('ref_axis',(1.,0.,0.));
#33031=DIRECTION('',(0.,0.,-1.));
#33032=DIRECTION('center_axis',(-1.,0.,0.));
#33033=DIRECTION('ref_axis',(0.,0.,1.));
#33034=DIRECTION('',(0.,1.,0.));
#33035=DIRECTION('',(0.,0.,-1.));
#33036=DIRECTION('center_axis',(0.,0.,-1.));
#33037=DIRECTION('ref_axis',(-1.,0.,0.));
#33038=DIRECTION('center_axis',(0.,0.,1.));
#33039=DIRECTION('ref_axis',(1.,0.,0.));
#33040=DIRECTION('',(0.,0.,-1.));
#33041=DIRECTION('center_axis',(-0.707106781186543,-0.707106781186552,0.));
#33042=DIRECTION('ref_axis',(0.707106781186553,-0.707106781186543,0.));
#33043=DIRECTION('',(-0.707106781186552,0.707106781186543,0.));
#33044=DIRECTION('',(0.,0.,-1.));
#33045=DIRECTION('center_axis',(0.,0.,-1.));
#33046=DIRECTION('ref_axis',(-1.,0.,0.));
#33047=DIRECTION('center_axis',(0.,0.,-1.));
#33048=DIRECTION('ref_axis',(1.,0.,0.));
#33049=DIRECTION('',(0.,0.,-1.));
#33050=DIRECTION('center_axis',(0.,0.,-1.));
#33051=DIRECTION('ref_axis',(-1.,0.,0.));
#33052=DIRECTION('center_axis',(0.,0.,1.));
#33053=DIRECTION('ref_axis',(1.,0.,0.));
#33054=DIRECTION('',(0.,0.,-1.));
#33055=DIRECTION('center_axis',(0.,0.,-1.));
#33056=DIRECTION('ref_axis',(-1.,0.,0.));
#33057=DIRECTION('center_axis',(0.,0.,-1.));
#33058=DIRECTION('ref_axis',(1.,0.,0.));
#33059=DIRECTION('',(0.,0.,-1.));
#33060=DIRECTION('center_axis',(-0.707106781186549,-0.707106781186546,0.));
#33061=DIRECTION('ref_axis',(0.707106781186546,-0.707106781186549,0.));
#33062=DIRECTION('',(-0.707106781186546,0.707106781186549,0.));
#33063=DIRECTION('',(0.,0.,-1.));
#33064=DIRECTION('center_axis',(0.,0.,-1.));
#33065=DIRECTION('ref_axis',(-1.,0.,0.));
#33066=DIRECTION('center_axis',(0.,0.,-1.));
#33067=DIRECTION('ref_axis',(1.,0.,0.));
#33068=DIRECTION('',(0.,0.,-1.));
#33069=DIRECTION('center_axis',(-1.,0.,0.));
#33070=DIRECTION('ref_axis',(0.,0.,1.));
#33071=DIRECTION('',(0.,1.,0.));
#33072=DIRECTION('',(0.,0.,-1.));
#33073=DIRECTION('center_axis',(0.,0.,-1.));
#33074=DIRECTION('ref_axis',(-1.,0.,0.));
#33075=DIRECTION('center_axis',(0.,0.,-1.));
#33076=DIRECTION('ref_axis',(1.,0.,0.));
#33077=DIRECTION('',(0.,0.,-1.));
#33078=DIRECTION('center_axis',(-0.70710678118655,0.707106781186545,0.));
#33079=DIRECTION('ref_axis',(-0.707106781186545,-0.70710678118655,0.));
#33080=DIRECTION('',(0.707106781186546,0.707106781186549,0.));
#33081=DIRECTION('',(0.,0.,-1.));
#33082=DIRECTION('center_axis',(0.,0.,-1.));
#33083=DIRECTION('ref_axis',(-1.,0.,0.));
#33084=DIRECTION('center_axis',(0.,0.,-1.));
#33085=DIRECTION('ref_axis',(1.,0.,0.));
#33086=DIRECTION('',(0.,0.,-1.));
#33087=DIRECTION('center_axis',(0.,0.,-1.));
#33088=DIRECTION('ref_axis',(-1.,0.,0.));
#33089=DIRECTION('center_axis',(0.,0.,1.));
#33090=DIRECTION('ref_axis',(1.,0.,0.));
#33091=DIRECTION('',(0.,0.,-1.));
#33092=DIRECTION('center_axis',(0.,0.,-1.));
#33093=DIRECTION('ref_axis',(-1.,0.,0.));
#33094=DIRECTION('center_axis',(0.,0.,-1.));
#33095=DIRECTION('ref_axis',(1.,0.,0.));
#33096=DIRECTION('',(0.,0.,-1.));
#33097=DIRECTION('center_axis',(-0.707106781186548,0.707106781186547,0.));
#33098=DIRECTION('ref_axis',(-0.707106781186547,-0.707106781186548,0.));
#33099=DIRECTION('',(0.707106781186547,0.707106781186548,0.));
#33100=DIRECTION('',(0.,0.,-1.));
#33101=DIRECTION('center_axis',(-4.61786466713945E-17,1.,0.));
#33102=DIRECTION('ref_axis',(-1.,-4.61786466713945E-17,0.));
#33103=DIRECTION('',(1.,4.61786466713945E-17,0.));
#33104=DIRECTION('',(0.,0.,-1.));
#33105=DIRECTION('center_axis',(0.707106781186549,0.707106781186546,0.));
#33106=DIRECTION('ref_axis',(-0.707106781186546,0.707106781186549,0.));
#33107=DIRECTION('',(0.707106781186546,-0.707106781186549,0.));
#33108=DIRECTION('',(0.,0.,-1.));
#33109=DIRECTION('center_axis',(0.,0.,-1.));
#33110=DIRECTION('ref_axis',(-1.,0.,0.));
#33111=DIRECTION('center_axis',(0.,0.,-1.));
#33112=DIRECTION('ref_axis',(1.,0.,0.));
#33113=DIRECTION('',(0.,0.,-1.));
#33114=DIRECTION('center_axis',(0.,0.,-1.));
#33115=DIRECTION('ref_axis',(-1.,0.,0.));
#33116=DIRECTION('center_axis',(0.,0.,1.));
#33117=DIRECTION('ref_axis',(1.,0.,0.));
#33118=DIRECTION('',(0.,0.,-1.));
#33119=DIRECTION('center_axis',(0.,0.,-1.));
#33120=DIRECTION('ref_axis',(-1.,0.,0.));
#33121=DIRECTION('center_axis',(0.,0.,-1.));
#33122=DIRECTION('ref_axis',(1.,0.,0.));
#33123=DIRECTION('',(0.,0.,-1.));
#33124=DIRECTION('center_axis',(0.707106781186548,0.707106781186548,0.));
#33125=DIRECTION('ref_axis',(-0.707106781186548,0.707106781186548,0.));
#33126=DIRECTION('',(0.707106781186547,-0.707106781186547,0.));
#33127=DIRECTION('',(0.,0.,-1.));
#33128=DIRECTION('center_axis',(0.,0.,-1.));
#33129=DIRECTION('ref_axis',(-1.,0.,0.));
#33130=DIRECTION('center_axis',(0.,0.,-1.));
#33131=DIRECTION('ref_axis',(1.,0.,0.));
#33132=DIRECTION('',(0.,0.,-1.));
#33133=DIRECTION('center_axis',(1.,0.,0.));
#33134=DIRECTION('ref_axis',(0.,0.,-1.));
#33135=DIRECTION('',(0.,-1.,0.));
#33136=DIRECTION('',(0.,0.,-1.));
#33137=DIRECTION('center_axis',(0.,0.,-1.));
#33138=DIRECTION('ref_axis',(-1.,0.,0.));
#33139=DIRECTION('center_axis',(0.,0.,-1.));
#33140=DIRECTION('ref_axis',(1.,0.,0.));
#33141=DIRECTION('',(0.,0.,-1.));
#33142=DIRECTION('center_axis',(0.707106781186543,-0.707106781186552,0.));
#33143=DIRECTION('ref_axis',(0.707106781186552,0.707106781186543,0.));
#33144=DIRECTION('',(-0.707106781186552,-0.707106781186543,0.));
#33145=DIRECTION('',(0.,0.,-1.));
#33146=DIRECTION('center_axis',(0.,0.,-1.));
#33147=DIRECTION('ref_axis',(-1.,0.,0.));
#33148=DIRECTION('center_axis',(0.,0.,-1.));
#33149=DIRECTION('ref_axis',(1.,0.,0.));
#33150=DIRECTION('',(0.,0.,-1.));
#33151=DIRECTION('center_axis',(0.,0.,-1.));
#33152=DIRECTION('ref_axis',(-1.,0.,0.));
#33153=DIRECTION('center_axis',(0.,0.,1.));
#33154=DIRECTION('ref_axis',(1.,0.,0.));
#33155=DIRECTION('',(0.,0.,-1.));
#33156=DIRECTION('center_axis',(0.,0.,-1.));
#33157=DIRECTION('ref_axis',(-1.,0.,0.));
#33158=DIRECTION('center_axis',(0.,0.,-1.));
#33159=DIRECTION('ref_axis',(1.,0.,0.));
#33160=DIRECTION('',(0.,0.,-1.));
#33161=DIRECTION('center_axis',(0.707106781186543,-0.707106781186552,0.));
#33162=DIRECTION('ref_axis',(0.707106781186552,0.707106781186543,0.));
#33163=DIRECTION('',(-0.707106781186552,-0.707106781186543,0.));
#33164=DIRECTION('',(0.,0.,-1.));
#33165=DIRECTION('center_axis',(0.,0.,-1.));
#33166=DIRECTION('ref_axis',(-1.,0.,0.));
#33167=DIRECTION('center_axis',(0.,0.,1.));
#33168=DIRECTION('ref_axis',(1.,0.,0.));
#33169=DIRECTION('',(0.,0.,-1.));
#33170=DIRECTION('center_axis',(1.,0.,0.));
#33171=DIRECTION('ref_axis',(0.,0.,-1.));
#33172=DIRECTION('',(0.,-1.,0.));
#33173=DIRECTION('',(0.,0.,-1.));
#33174=DIRECTION('center_axis',(0.,0.,-1.));
#33175=DIRECTION('ref_axis',(-1.,0.,0.));
#33176=DIRECTION('center_axis',(0.,0.,1.));
#33177=DIRECTION('ref_axis',(1.,0.,0.));
#33178=DIRECTION('',(0.,0.,-1.));
#33179=DIRECTION('center_axis',(0.707106781186549,0.707106781186546,0.));
#33180=DIRECTION('ref_axis',(-0.707106781186546,0.707106781186549,0.));
#33181=DIRECTION('',(0.707106781186546,-0.707106781186549,0.));
#33182=DIRECTION('center_axis',(-1.19636101791504E-15,1.,-1.04815936541451E-31));
#33183=DIRECTION('ref_axis',(-1.,-1.19636101791504E-15,0.));
#33184=DIRECTION('',(1.,1.19636101791504E-15,3.7386281809845E-17));
#33185=DIRECTION('',(-4.38061483832527E-16,-6.28895619248706E-31,-1.));
#33186=DIRECTION('',(-1.,-1.19636101791504E-15,0.));
#33187=DIRECTION('',(-8.76122967665054E-17,0.,1.));
#33188=DIRECTION('center_axis',(0.707106781186554,0.707106781186541,-3.09756245794624E-16));
#33189=DIRECTION('ref_axis',(4.38061483832527E-16,6.55212072256257E-31,
1.));
#33190=DIRECTION('',(-0.707106781186541,0.707106781186554,-2.64360933910924E-17));
#33191=DIRECTION('',(-4.38061483832527E-16,0.,-1.));
#33192=DIRECTION('',(0.707106781186541,-0.707106781186554,0.));
#33193=DIRECTION('center_axis',(0.,-1.,0.));
#33194=DIRECTION('ref_axis',(0.,0.,-1.));
#33195=DIRECTION('',(-1.,0.,0.));
#33196=DIRECTION('',(0.,0.,1.));
#33197=DIRECTION('',(1.,0.,0.));
#33198=DIRECTION('center_axis',(-0.707106781186533,-0.707106781186562,0.));
#33199=DIRECTION('ref_axis',(0.707106781186562,-0.707106781186533,0.));
#33200=DIRECTION('',(-0.707106781186562,0.707106781186533,0.));
#33201=DIRECTION('',(0.,0.,1.));
#33202=DIRECTION('',(0.707106781186562,-0.707106781186533,0.));
#33203=DIRECTION('center_axis',(-1.,1.26161707343768E-16,0.));
#33204=DIRECTION('ref_axis',(-1.26161707343768E-16,-1.,0.));
#33205=DIRECTION('',(1.26161707343768E-16,1.,0.));
#33206=DIRECTION('',(0.,0.,1.));
#33207=DIRECTION('',(-1.26161707343768E-16,-1.,0.));
#33208=DIRECTION('center_axis',(1.,1.26161707343768E-16,0.));
#33209=DIRECTION('ref_axis',(-1.26161707343768E-16,1.,0.));
#33210=DIRECTION('',(1.26161707343768E-16,-1.,0.));
#33211=DIRECTION('',(0.,0.,1.));
#33212=DIRECTION('',(-1.26161707343768E-16,1.,0.));
#33213=DIRECTION('',(0.,0.,1.));
#33214=DIRECTION('center_axis',(0.707106781186533,-0.707106781186562,0.));
#33215=DIRECTION('ref_axis',(0.707106781186562,0.707106781186533,0.));
#33216=DIRECTION('',(-0.707106781186562,-0.707106781186533,0.));
#33217=DIRECTION('',(0.,0.,1.));
#33218=DIRECTION('',(0.707106781186562,0.707106781186533,0.));
#33219=DIRECTION('center_axis',(0.,-1.,0.));
#33220=DIRECTION('ref_axis',(0.,0.,-1.));
#33221=DIRECTION('',(-1.,0.,0.));
#33222=DIRECTION('',(-8.76122967665054E-17,0.,1.));
#33223=DIRECTION('',(1.,0.,0.));
#33224=DIRECTION('center_axis',(-0.707106781186554,0.707106781186542,-6.19512491589247E-17));
#33225=DIRECTION('ref_axis',(8.76122967665054E-17,3.85000586821995E-33,
-1.));
#33226=DIRECTION('',(0.707106781186541,0.707106781186554,0.));
#33227=DIRECTION('',(-0.707106781186541,-0.707106781186554,-2.64360933910925E-17));
#33228=DIRECTION('center_axis',(1.,0.,0.));
#33229=DIRECTION('ref_axis',(0.,0.,-1.));
#33230=DIRECTION('',(0.,1.,0.));
#33231=DIRECTION('',(0.,0.,-1.));
#33232=DIRECTION('',(0.,1.,0.));
#33233=DIRECTION('',(0.,0.,1.));
#33234=DIRECTION('center_axis',(0.70710678118655,0.707106781186545,0.));
#33235=DIRECTION('ref_axis',(-0.707106781186545,0.70710678118655,0.));
#33236=DIRECTION('',(-0.707106781186545,0.70710678118655,0.));
#33237=DIRECTION('',(0.,0.,1.));
#33238=DIRECTION('',(-0.707106781186545,0.70710678118655,0.));
#33239=DIRECTION('center_axis',(0.,1.,0.));
#33240=DIRECTION('ref_axis',(0.,0.,1.));
#33241=DIRECTION('',(0.,0.,1.));
#33242=DIRECTION('',(-1.,0.,0.));
#33243=DIRECTION('',(-1.,0.,0.));
#33244=DIRECTION('center_axis',(0.707106781186549,-0.707106781186546,0.));
#33245=DIRECTION('ref_axis',(0.707106781186546,0.707106781186549,0.));
#33246=DIRECTION('',(0.,0.,1.));
#33247=DIRECTION('',(0.707106781186546,0.707106781186549,0.));
#33248=DIRECTION('',(0.707106781186546,0.707106781186549,0.));
#33249=DIRECTION('center_axis',(-1.62579519772897E-16,-1.,0.));
#33250=DIRECTION('ref_axis',(1.,-1.62579519772897E-16,0.));
#33251=DIRECTION('',(0.,0.,1.));
#33252=DIRECTION('',(1.,-1.62579519772897E-16,0.));
#33253=DIRECTION('',(1.,-1.62579519772897E-16,0.));
#33254=DIRECTION('center_axis',(-0.707106781186544,-0.707106781186551,0.));
#33255=DIRECTION('ref_axis',(0.707106781186551,-0.707106781186544,0.));
#33256=DIRECTION('',(0.,0.,1.));
#33257=DIRECTION('',(0.707106781186551,-0.707106781186544,0.));
#33258=DIRECTION('',(0.707106781186551,-0.707106781186544,0.));
#33259=DIRECTION('center_axis',(0.,1.,0.));
#33260=DIRECTION('ref_axis',(0.,0.,1.));
#33261=DIRECTION('',(-1.,0.,0.));
#33262=DIRECTION('',(0.,0.,1.));
#33263=DIRECTION('',(-1.,0.,0.));
#33264=DIRECTION('center_axis',(0.707106781186544,-0.707106781186551,0.));
#33265=DIRECTION('ref_axis',(0.707106781186551,0.707106781186544,0.));
#33266=DIRECTION('',(0.,0.,1.));
#33267=DIRECTION('',(0.707106781186551,0.707106781186544,0.));
#33268=DIRECTION('',(0.707106781186551,0.707106781186544,0.));
#33269=DIRECTION('center_axis',(1.62579519772897E-16,-1.,0.));
#33270=DIRECTION('ref_axis',(1.,1.62579519772897E-16,0.));
#33271=DIRECTION('',(0.,0.,1.));
#33272=DIRECTION('',(1.,1.62579519772897E-16,0.));
#33273=DIRECTION('',(1.,1.62579519772897E-16,0.));
#33274=DIRECTION('center_axis',(-0.707106781186549,-0.707106781186546,0.));
#33275=DIRECTION('ref_axis',(0.707106781186546,-0.707106781186549,0.));
#33276=DIRECTION('',(0.,0.,1.));
#33277=DIRECTION('',(0.707106781186546,-0.707106781186549,0.));
#33278=DIRECTION('',(0.707106781186546,-0.707106781186549,0.));
#33279=DIRECTION('center_axis',(0.,1.,0.));
#33280=DIRECTION('ref_axis',(0.,0.,1.));
#33281=DIRECTION('',(-1.,0.,0.));
#33282=DIRECTION('',(0.,0.,1.));
#33283=DIRECTION('',(-1.,0.,0.));
#33284=DIRECTION('center_axis',(-0.70710678118655,0.707106781186545,0.));
#33285=DIRECTION('ref_axis',(-0.707106781186545,-0.70710678118655,0.));
#33286=DIRECTION('',(-0.707106781186545,-0.70710678118655,0.));
#33287=DIRECTION('',(0.,0.,1.));
#33288=DIRECTION('',(-0.707106781186545,-0.70710678118655,0.));
#33289=DIRECTION('center_axis',(-1.,0.,0.));
#33290=DIRECTION('ref_axis',(0.,0.,1.));
#33291=DIRECTION('',(0.,-1.,0.));
#33292=DIRECTION('',(0.,0.,1.));
#33293=DIRECTION('',(0.,-1.,0.));
#33294=DIRECTION('center_axis',(-0.707106781186546,-0.707106781186549,0.));
#33295=DIRECTION('ref_axis',(0.707106781186549,-0.707106781186546,0.));
#33296=DIRECTION('',(0.707106781186549,-0.707106781186546,0.));
#33297=DIRECTION('',(0.,0.,1.));
#33298=DIRECTION('',(0.707106781186549,-0.707106781186546,0.));
#33299=DIRECTION('center_axis',(-1.,0.,0.));
#33300=DIRECTION('ref_axis',(0.,0.,1.));
#33301=DIRECTION('',(0.,-1.,0.));
#33302=DIRECTION('',(0.,0.,1.));
#33303=DIRECTION('',(0.,-1.,0.));
#33304=DIRECTION('center_axis',(1.2823896663807E-16,1.,0.));
#33305=DIRECTION('ref_axis',(-1.,1.2823896663807E-16,0.));
#33306=DIRECTION('center_axis',(-1.2823896663807E-16,-1.,0.));
#33307=DIRECTION('ref_axis',(-1.,1.2823896663807E-16,2.52323414687535E-15));
#33308=DIRECTION('',(1.,-1.2823896663807E-16,0.));
#33309=DIRECTION('',(0.,0.,-1.));
#33310=DIRECTION('center_axis',(1.,-2.04085114820801E-16,0.));
#33311=DIRECTION('ref_axis',(2.04085114820801E-16,1.,0.));
#33312=DIRECTION('',(0.,0.,1.));
#33313=DIRECTION('',(0.,1.,0.));
#33314=DIRECTION('',(-2.04085114820801E-16,-1.,0.));
#33315=DIRECTION('center_axis',(-0.965925826289069,-0.258819045102518,0.));
#33316=DIRECTION('ref_axis',(0.258819045102518,-0.965925826289069,0.));
#33317=DIRECTION('center_axis',(-0.965925826289069,-0.258819045102518,0.));
#33318=DIRECTION('ref_axis',(0.258819045102518,-0.965925826289069,0.));
#33319=DIRECTION('',(0.258819045102518,-0.965925826289069,0.));
#33320=DIRECTION('',(0.,0.,1.));
#33321=DIRECTION('center_axis',(0.965925826289069,-0.258819045102518,0.));
#33322=DIRECTION('ref_axis',(0.258819045102518,0.965925826289069,0.));
#33323=DIRECTION('center_axis',(0.965925826289069,-0.258819045102518,0.));
#33324=DIRECTION('ref_axis',(0.258819045102518,0.965925826289069,0.));
#33325=DIRECTION('',(0.258819045102518,0.965925826289069,0.));
#33326=DIRECTION('',(0.,0.,-1.));
#33327=DIRECTION('center_axis',(-1.,-2.04085114820801E-16,0.));
#33328=DIRECTION('ref_axis',(2.04085114820801E-16,-1.,0.));
#33329=DIRECTION('',(0.,0.,-1.));
#33330=DIRECTION('',(0.,-1.,0.));
#33331=DIRECTION('',(-2.04085114820801E-16,1.,0.));
#33332=DIRECTION('center_axis',(-1.2823896663807E-16,1.,0.));
#33333=DIRECTION('ref_axis',(-1.,-1.2823896663807E-16,0.));
#33334=DIRECTION('',(1.,1.2823896663807E-16,0.));
#33335=DIRECTION('center_axis',(-1.2823896663807E-16,-1.,0.));
#33336=DIRECTION('ref_axis',(-1.,1.2823896663807E-16,-2.52323414687536E-15));
#33337=DIRECTION('center_axis',(-0.61566147532566,-0.788010753606721,0.));
#33338=DIRECTION('ref_axis',(0.78801075360672,-0.61566147532566,0.));
#33339=DIRECTION('center_axis',(-0.615661475325663,-0.788010753606718,3.86575390646386E-15));
#33340=DIRECTION('ref_axis',(0.788010753606718,-0.615661475325663,-6.5758767605984E-13));
#33341=DIRECTION('',(0.78801075360672,-0.61566147532566,0.));
#33342=DIRECTION('',(0.,0.,1.));
#33343=DIRECTION('center_axis',(0.707106781186548,0.707106781186547,0.));
#33344=DIRECTION('ref_axis',(-0.707106781186547,0.707106781186548,0.));
#33345=DIRECTION('',(0.707106781186547,-0.707106781186548,0.));
#33346=DIRECTION('',(-0.707106781186547,0.707106781186548,0.));
#33347=DIRECTION('',(0.,0.,1.));
#33348=DIRECTION('center_axis',(-0.707106781186548,0.707106781186547,0.));
#33349=DIRECTION('ref_axis',(-0.707106781186547,-0.707106781186548,0.));
#33350=DIRECTION('',(0.707106781186547,0.707106781186548,0.));
#33351=DIRECTION('',(0.,0.,1.));
#33352=DIRECTION('',(-0.707106781186547,-0.707106781186548,0.));
#33353=DIRECTION('center_axis',(0.,0.,1.));
#33354=DIRECTION('ref_axis',(1.,0.,0.));
#33355=DIRECTION('',(1.,0.,0.));
#33356=DIRECTION('',(1.,-4.33680868994201E-15,0.));
#33357=DIRECTION('',(0.78801075360672,0.61566147532566,0.));
#33358=DIRECTION('center_axis',(0.61566147532566,-0.788010753606721,0.));
#33359=DIRECTION('ref_axis',(0.78801075360672,0.61566147532566,0.));
#33360=DIRECTION('center_axis',(0.615661475325666,-0.788010753606716,-4.56861825309369E-15));
#33361=DIRECTION('ref_axis',(0.788010753606716,0.615661475325665,-3.955354877202E-13));
#33362=DIRECTION('',(0.,0.,1.));
#33363=DIRECTION('center_axis',(3.7386281809845E-17,4.26676715361993E-32,
-1.));
#33364=DIRECTION('ref_axis',(-1.,4.36567830323557E-65,-3.7386281809845E-17));
#33365=DIRECTION('',(1.,0.,0.));
#33366=DIRECTION('',(0.707106781186546,0.707106781186549,0.));
#33367=DIRECTION('center_axis',(0.,0.,1.));
#33368=DIRECTION('ref_axis',(1.,0.,0.));
#33369=DIRECTION('',(0.,1.,0.));
#33370=DIRECTION('center_axis',(0.,0.,1.));
#33371=DIRECTION('ref_axis',(1.,0.,0.));
#33372=DIRECTION('',(-0.707106781186549,0.707106781186546,0.));
#33373=DIRECTION('center_axis',(0.,0.,-1.));
#33374=DIRECTION('ref_axis',(1.,0.,0.));
#33375=DIRECTION('center_axis',(0.,0.,1.));
#33376=DIRECTION('ref_axis',(1.,0.,0.));
#33377=DIRECTION('center_axis',(0.,0.,-1.));
#33378=DIRECTION('ref_axis',(1.,0.,0.));
#33379=DIRECTION('',(-0.707106781186548,0.707106781186547,0.));
#33380=DIRECTION('center_axis',(0.,0.,-1.));
#33381=DIRECTION('ref_axis',(1.,0.,0.));
#33382=DIRECTION('',(0.,1.,0.));
#33383=DIRECTION('center_axis',(0.,0.,-1.));
#33384=DIRECTION('ref_axis',(1.,0.,0.));
#33385=DIRECTION('',(0.707106781186545,0.70710678118655,0.));
#33386=DIRECTION('center_axis',(0.,0.,-1.));
#33387=DIRECTION('ref_axis',(1.,0.,0.));
#33388=DIRECTION('center_axis',(0.,0.,1.));
#33389=DIRECTION('ref_axis',(1.,0.,0.));
#33390=DIRECTION('center_axis',(0.,0.,-1.));
#33391=DIRECTION('ref_axis',(1.,0.,0.));
#33392=DIRECTION('',(0.707106781186546,0.707106781186549,0.));
#33393=DIRECTION('',(1.,1.22464679914735E-16,0.));
#33394=DIRECTION('',(0.707106781186546,-0.707106781186549,0.));
#33395=DIRECTION('center_axis',(0.,0.,-1.));
#33396=DIRECTION('ref_axis',(1.,0.,0.));
#33397=DIRECTION('center_axis',(0.,0.,1.));
#33398=DIRECTION('ref_axis',(1.,0.,0.));
#33399=DIRECTION('center_axis',(0.,0.,-1.));
#33400=DIRECTION('ref_axis',(1.,0.,0.));
#33401=DIRECTION('',(0.707106781186545,-0.70710678118655,0.));
#33402=DIRECTION('center_axis',(0.,0.,-1.));
#33403=DIRECTION('ref_axis',(1.,0.,0.));
#33404=DIRECTION('',(0.,-1.,0.));
#33405=DIRECTION('center_axis',(0.,0.,-1.));
#33406=DIRECTION('ref_axis',(1.,0.,0.));
#33407=DIRECTION('',(-0.707106781186548,-0.707106781186547,0.));
#33408=DIRECTION('center_axis',(0.,0.,-1.));
#33409=DIRECTION('ref_axis',(1.,0.,0.));
#33410=DIRECTION('center_axis',(0.,0.,1.));
#33411=DIRECTION('ref_axis',(1.,0.,0.));
#33412=DIRECTION('center_axis',(0.,0.,-1.));
#33413=DIRECTION('ref_axis',(1.,0.,0.));
#33414=DIRECTION('',(-0.707106781186549,-0.707106781186546,0.));
#33415=DIRECTION('center_axis',(0.,0.,1.));
#33416=DIRECTION('ref_axis',(1.,0.,0.));
#33417=DIRECTION('',(0.,-1.,0.));
#33418=DIRECTION('center_axis',(0.,0.,1.));
#33419=DIRECTION('ref_axis',(1.,0.,0.));
#33420=DIRECTION('',(0.707106781186546,-0.707106781186549,0.));
#33421=DIRECTION('',(1.,-3.50803534070133E-16,0.));
#33422=DIRECTION('center_axis',(0.,0.,-1.));
#33423=DIRECTION('ref_axis',(-1.,0.,0.));
#33424=DIRECTION('',(1.,-4.33680868994201E-15,0.));
#33425=DIRECTION('',(-0.707106781186547,-0.707106781186548,0.));
#33426=DIRECTION('',(-1.26161707343768E-16,-1.,0.));
#33427=DIRECTION('',(0.707106781186562,-0.707106781186533,0.));
#33428=DIRECTION('',(1.,0.,0.));
#33429=DIRECTION('',(-0.707106781186548,0.707106781186547,0.));
#33430=DIRECTION('',(1.,1.19636101791504E-15,0.));
#33431=DIRECTION('',(-0.707106781186541,-0.707106781186554,0.));
#33432=DIRECTION('',(1.,0.,0.));
#33433=DIRECTION('',(0.707106781186562,0.707106781186533,0.));
#33434=DIRECTION('',(-1.26161707343768E-16,1.,0.));
#33435=DIRECTION('',(-0.707106781186547,0.707106781186548,0.));
#33436=DIRECTION('',(1.,0.,0.));
#33437=DIRECTION('center_axis',(-0.707106781186554,0.707106781186542,1.85853747476774E-16));
#33438=DIRECTION('ref_axis',(-2.62836890299516E-16,1.6519124519235E-33,
-1.));
#33439=DIRECTION('',(0.707106781186541,0.707106781186554,0.));
#33440=DIRECTION('',(2.62836890299516E-16,0.,1.));
#33441=DIRECTION('',(2.62836890299516E-16,0.,1.));
#33442=DIRECTION('center_axis',(-0.707106781186533,-0.707106781186562,0.));
#33443=DIRECTION('ref_axis',(0.707106781186562,-0.707106781186533,0.));
#33444=DIRECTION('',(-0.707106781186562,0.707106781186533,0.));
#33445=DIRECTION('',(0.,0.,1.));
#33446=DIRECTION('',(0.,0.,1.));
#33447=DIRECTION('center_axis',(-1.,1.26161707343768E-16,0.));
#33448=DIRECTION('ref_axis',(-1.26161707343768E-16,-1.,0.));
#33449=DIRECTION('',(1.26161707343768E-16,1.,0.));
#33450=DIRECTION('',(0.,0.,1.));
#33451=DIRECTION('center_axis',(-0.707106781186548,0.707106781186547,0.));
#33452=DIRECTION('ref_axis',(-0.707106781186547,-0.707106781186548,0.));
#33453=DIRECTION('',(0.707106781186547,0.707106781186548,0.));
#33454=DIRECTION('',(0.,0.,1.));
#33455=DIRECTION('center_axis',(0.,-1.,0.));
#33456=DIRECTION('ref_axis',(0.,0.,-1.));
#33457=DIRECTION('',(-1.,0.,0.));
#33458=DIRECTION('',(2.62836890299516E-16,0.,-1.));
#33459=DIRECTION('center_axis',(0.,0.,1.));
#33460=DIRECTION('ref_axis',(1.,0.,0.));
#33461=DIRECTION('',(0.,0.,1.));
#33462=DIRECTION('center_axis',(0.,0.,1.));
#33463=DIRECTION('ref_axis',(1.,0.,0.));
#33464=DIRECTION('',(0.,0.,-1.));
#33465=DIRECTION('center_axis',(0.,0.,1.));
#33466=DIRECTION('ref_axis',(1.,0.,0.));
#33467=DIRECTION('',(0.,0.,1.));
#33468=DIRECTION('center_axis',(0.,0.,1.));
#33469=DIRECTION('ref_axis',(1.,0.,0.));
#33470=DIRECTION('',(0.,0.,-1.));
#33471=DIRECTION('center_axis',(-1.,0.,0.));
#33472=DIRECTION('ref_axis',(0.,0.,1.));
#33473=DIRECTION('',(0.,-1.,0.));
#33474=DIRECTION('center_axis',(-0.707106781186549,-0.707106781186546,0.));
#33475=DIRECTION('ref_axis',(0.707106781186546,-0.707106781186549,0.));
#33476=DIRECTION('',(0.707106781186546,-0.707106781186549,0.));
#33477=DIRECTION('',(0.,0.,1.));
#33478=DIRECTION('center_axis',(-6.49101394191508E-16,-1.,0.));
#33479=DIRECTION('ref_axis',(1.,-6.49101394191508E-16,0.));
#33480=DIRECTION('',(1.,-3.50803534070133E-16,0.));
#33481=DIRECTION('center_axis',(0.,0.,1.));
#33482=DIRECTION('ref_axis',(1.,0.,0.));
#33483=DIRECTION('center_axis',(0.,0.,-1.));
#33484=DIRECTION('ref_axis',(1.,0.,0.));
#33485=DIRECTION('',(0.,0.,-1.));
#33486=DIRECTION('',(0.,0.,1.));
#33487=DIRECTION('center_axis',(0.,0.,1.));
#33488=DIRECTION('ref_axis',(1.,0.,0.));
#33489=DIRECTION('center_axis',(0.,0.,-1.));
#33490=DIRECTION('ref_axis',(1.,0.,0.));
#33491=DIRECTION('',(0.,0.,-1.));
#33492=DIRECTION('',(0.,0.,1.));
#33493=DIRECTION('center_axis',(0.,0.,1.));
#33494=DIRECTION('ref_axis',(1.,0.,0.));
#33495=DIRECTION('center_axis',(0.,0.,1.));
#33496=DIRECTION('ref_axis',(1.,0.,0.));
#33497=DIRECTION('center_axis',(0.,0.,-1.));
#33498=DIRECTION('ref_axis',(-1.,0.,0.));
#33499=DIRECTION('center_axis',(0.,0.,-1.));
#33500=DIRECTION('ref_axis',(1.,0.,0.));
#33501=DIRECTION('',(0.,0.,-1.));
#33502=DIRECTION('',(0.,0.,1.));
#33503=DIRECTION('center_axis',(0.,0.,-1.));
#33504=DIRECTION('ref_axis',(-1.,0.,0.));
#33505=DIRECTION('center_axis',(0.,0.,-1.));
#33506=DIRECTION('ref_axis',(1.,0.,0.));
#33507=DIRECTION('',(0.,0.,-1.));
#33508=DIRECTION('',(0.,0.,1.));
#33509=DIRECTION('center_axis',(-1.,0.,0.));
#33510=DIRECTION('ref_axis',(0.,0.,1.));
#33511=DIRECTION('',(0.,-1.,0.));
#33512=DIRECTION('center_axis',(-0.707106781186546,0.707106781186549,0.));
#33513=DIRECTION('ref_axis',(-0.707106781186549,-0.707106781186546,0.));
#33514=DIRECTION('',(-0.707106781186548,-0.707106781186547,0.));
#33515=DIRECTION('center_axis',(0.,0.,1.));
#33516=DIRECTION('ref_axis',(1.,0.,0.));
#33517=DIRECTION('center_axis',(0.,0.,-1.));
#33518=DIRECTION('ref_axis',(1.,0.,0.));
#33519=DIRECTION('',(0.,0.,-1.));
#33520=DIRECTION('',(0.,0.,1.));
#33521=DIRECTION('center_axis',(0.,0.,1.));
#33522=DIRECTION('ref_axis',(1.,0.,0.));
#33523=DIRECTION('center_axis',(0.,0.,-1.));
#33524=DIRECTION('ref_axis',(1.,0.,0.));
#33525=DIRECTION('',(0.,0.,-1.));
#33526=DIRECTION('',(0.,0.,1.));
#33527=DIRECTION('center_axis',(0.,0.,1.));
#33528=DIRECTION('ref_axis',(1.,0.,0.));
#33529=DIRECTION('center_axis',(0.,0.,1.));
#33530=DIRECTION('ref_axis',(1.,0.,0.));
#33531=DIRECTION('center_axis',(1.22464679914735E-16,-1.,0.));
#33532=DIRECTION('ref_axis',(1.,1.22464679914735E-16,0.));
#33533=DIRECTION('',(0.,0.,1.));
#33534=DIRECTION('',(1.,1.22464679914735E-16,0.));
#33535=DIRECTION('',(0.,0.,1.));
#33536=DIRECTION('center_axis',(-0.707106781186549,-0.707106781186546,0.));
#33537=DIRECTION('ref_axis',(0.707106781186546,-0.707106781186549,0.));
#33538=DIRECTION('',(0.707106781186546,-0.707106781186549,0.));
#33539=DIRECTION('center_axis',(0.,0.,1.));
#33540=DIRECTION('ref_axis',(1.,0.,0.));
#33541=DIRECTION('center_axis',(0.,0.,-1.));
#33542=DIRECTION('ref_axis',(1.,0.,0.));
#33543=DIRECTION('',(0.,0.,-1.));
#33544=DIRECTION('',(0.,0.,1.));
#33545=DIRECTION('center_axis',(0.,0.,1.));
#33546=DIRECTION('ref_axis',(1.,0.,0.));
#33547=DIRECTION('center_axis',(0.,0.,-1.));
#33548=DIRECTION('ref_axis',(1.,0.,0.));
#33549=DIRECTION('',(0.,0.,-1.));
#33550=DIRECTION('',(0.,0.,1.));
#33551=DIRECTION('center_axis',(0.,0.,1.));
#33552=DIRECTION('ref_axis',(1.,0.,0.));
#33553=DIRECTION('center_axis',(0.,0.,1.));
#33554=DIRECTION('ref_axis',(1.,0.,0.));
#33555=DIRECTION('center_axis',(0.,0.,-1.));
#33556=DIRECTION('ref_axis',(-1.,0.,0.));
#33557=DIRECTION('center_axis',(0.,0.,-1.));
#33558=DIRECTION('ref_axis',(1.,0.,0.));
#33559=DIRECTION('',(0.,0.,-1.));
#33560=DIRECTION('',(0.,0.,1.));
#33561=DIRECTION('center_axis',(0.,0.,-1.));
#33562=DIRECTION('ref_axis',(-1.,0.,0.));
#33563=DIRECTION('center_axis',(0.,0.,-1.));
#33564=DIRECTION('ref_axis',(1.,0.,0.));
#33565=DIRECTION('',(0.,0.,-1.));
#33566=DIRECTION('',(0.,0.,1.));
#33567=DIRECTION('center_axis',(1.,0.,0.));
#33568=DIRECTION('ref_axis',(0.,0.,-1.));
#33569=DIRECTION('',(0.,1.,0.));
#33570=DIRECTION('center_axis',(0.707106781186549,-0.707106781186546,0.));
#33571=DIRECTION('ref_axis',(0.707106781186546,0.707106781186549,0.));
#33572=DIRECTION('',(0.707106781186545,0.70710678118655,0.));
#33573=DIRECTION('center_axis',(0.707106781186549,-0.707106781186546,0.));
#33574=DIRECTION('ref_axis',(0.707106781186546,0.707106781186549,0.));
#33575=DIRECTION('',(0.707106781186546,0.707106781186549,0.));
#33576=DIRECTION('center_axis',(0.,0.,1.));
#33577=DIRECTION('ref_axis',(1.,0.,0.));
#33578=DIRECTION('center_axis',(0.,0.,-1.));
#33579=DIRECTION('ref_axis',(1.,0.,0.));
#33580=DIRECTION('',(0.,0.,-1.));
#33581=DIRECTION('',(0.,0.,1.));
#33582=DIRECTION('center_axis',(0.,0.,1.));
#33583=DIRECTION('ref_axis',(1.,0.,0.));
#33584=DIRECTION('center_axis',(0.,0.,-1.));
#33585=DIRECTION('ref_axis',(1.,0.,0.));
#33586=DIRECTION('',(0.,0.,-1.));
#33587=DIRECTION('',(0.,0.,1.));
#33588=DIRECTION('center_axis',(0.,0.,1.));
#33589=DIRECTION('ref_axis',(1.,0.,0.));
#33590=DIRECTION('center_axis',(0.,0.,1.));
#33591=DIRECTION('ref_axis',(1.,0.,0.));
#33592=DIRECTION('center_axis',(0.,0.,1.));
#33593=DIRECTION('ref_axis',(1.,0.,0.));
#33594=DIRECTION('',(0.,0.,1.));
#33595=DIRECTION('center_axis',(0.,0.,1.));
#33596=DIRECTION('ref_axis',(1.,0.,0.));
#33597=DIRECTION('',(0.,0.,-1.));
#33598=DIRECTION('center_axis',(0.,0.,1.));
#33599=DIRECTION('ref_axis',(1.,0.,0.));
#33600=DIRECTION('',(0.,0.,1.));
#33601=DIRECTION('center_axis',(0.,0.,1.));
#33602=DIRECTION('ref_axis',(1.,0.,0.));
#33603=DIRECTION('',(0.,0.,-1.));
#33604=DIRECTION('center_axis',(0.707106781186548,0.707106781186547,0.));
#33605=DIRECTION('ref_axis',(-0.707106781186547,0.707106781186548,0.));
#33606=DIRECTION('',(0.707106781186547,-0.707106781186548,0.));
#33607=DIRECTION('',(0.,0.,1.));
#33608=DIRECTION('',(0.,0.,1.));
#33609=DIRECTION('center_axis',(1.,1.26161707343768E-16,0.));
#33610=DIRECTION('ref_axis',(-1.26161707343768E-16,1.,0.));
#33611=DIRECTION('',(1.26161707343768E-16,-1.,0.));
#33612=DIRECTION('',(0.,0.,1.));
#33613=DIRECTION('center_axis',(0.707106781186533,-0.707106781186562,0.));
#33614=DIRECTION('ref_axis',(0.707106781186562,0.707106781186533,0.));
#33615=DIRECTION('',(-0.707106781186562,-0.707106781186533,0.));
#33616=DIRECTION('',(0.,0.,1.));
#33617=DIRECTION('center_axis',(0.,-1.,0.));
#33618=DIRECTION('ref_axis',(0.,0.,-1.));
#33619=DIRECTION('',(-1.,0.,0.));
#33620=DIRECTION('center_axis',(0.,-1.,0.));
#33621=DIRECTION('ref_axis',(0.,0.,-1.));
#33622=DIRECTION('',(1.,0.,0.));
#33623=DIRECTION('',(0.,0.,1.));
#33624=DIRECTION('center_axis',(0.707106781186549,-0.707106781186546,0.));
#33625=DIRECTION('ref_axis',(0.707106781186546,0.707106781186549,0.));
#33626=DIRECTION('',(0.707106781186546,0.707106781186549,0.));
#33627=DIRECTION('center_axis',(1.,0.,0.));
#33628=DIRECTION('ref_axis',(0.,0.,-1.));
#33629=DIRECTION('',(0.,1.,0.));
#33630=DIRECTION('center_axis',(0.707106781186546,0.707106781186549,0.));
#33631=DIRECTION('ref_axis',(-0.707106781186549,0.707106781186546,0.));
#33632=DIRECTION('',(-0.707106781186549,0.707106781186546,0.));
#33633=DIRECTION('center_axis',(0.707106781186546,0.707106781186549,0.));
#33634=DIRECTION('ref_axis',(-0.707106781186549,0.707106781186546,0.));
#33635=DIRECTION('',(-0.707106781186548,0.707106781186547,0.));
#33636=DIRECTION('center_axis',(-0.707106781186549,-0.707106781186546,0.));
#33637=DIRECTION('ref_axis',(0.707106781186546,-0.707106781186549,0.));
#33638=DIRECTION('',(0.707106781186545,-0.70710678118655,0.));
#33639=DIRECTION('center_axis',(-0.707106781186546,0.707106781186549,0.));
#33640=DIRECTION('ref_axis',(-0.707106781186549,-0.707106781186546,0.));
#33641=DIRECTION('',(-0.707106781186549,-0.707106781186546,0.));
#33642=DIRECTION('center_axis',(0.707106781186547,0.707106781186548,1.85853747476773E-16));
#33643=DIRECTION('ref_axis',(-2.62836890299516E-16,-6.09040047468605E-31,
1.));
#33644=DIRECTION('',(0.707106781186548,-0.707106781186547,0.));
#33645=DIRECTION('',(2.62836890299516E-16,6.28895619248706E-31,-1.));
#33646=DIRECTION('center_axis',(-1.19636101791504E-15,1.,3.14447809624353E-31));
#33647=DIRECTION('ref_axis',(-1.,-1.19636101791504E-15,0.));
#33648=DIRECTION('',(-1.,-1.19636101791504E-15,0.));
#33649=DIRECTION('center_axis',(0.,0.,1.));
#33650=DIRECTION('ref_axis',(1.,0.,0.));
#33651=DIRECTION('center_axis',(1.,1.73472347597681E-16,0.));
#33652=DIRECTION('ref_axis',(-1.73472347597681E-16,1.,0.));
#33653=DIRECTION('',(-1.73472347597681E-16,1.,0.));
#33654=DIRECTION('',(0.,0.,1.));
#33655=DIRECTION('center_axis',(0.,0.,1.));
#33656=DIRECTION('ref_axis',(1.,0.,0.));
#33657=DIRECTION('center_axis',(0.,0.,1.));
#33658=DIRECTION('ref_axis',(1.,0.,0.));
#33659=DIRECTION('',(0.,0.,1.));
#33660=DIRECTION('center_axis',(-1.,1.73472347597681E-16,0.));
#33661=DIRECTION('ref_axis',(-1.73472347597681E-16,-1.,0.));
#33662=DIRECTION('',(-1.73472347597681E-16,-1.,0.));
#33663=DIRECTION('center_axis',(0.,0.,1.));
#33664=DIRECTION('ref_axis',(1.,0.,0.));
#33665=DIRECTION('center_axis',(0.,-1.,0.));
#33666=DIRECTION('ref_axis',(0.,0.,-1.));
#33667=DIRECTION('center_axis',(0.,-1.,0.));
#33668=DIRECTION('ref_axis',(0.,0.,-1.));
#33669=DIRECTION('center_axis',(0.,-1.,0.));
#33670=DIRECTION('ref_axis',(0.,0.,-1.));
#33671=DIRECTION('center_axis',(0.,-1.,0.));
#33672=DIRECTION('ref_axis',(0.,0.,-1.));
#54036=CARTESIAN_POINT('',(0.,0.,0.));
#54037=CARTESIAN_POINT('Origin',(23.2,9.00000000000001,-77.4));
#54038=CARTESIAN_POINT('',(17.28,9.00000000000001,-74.9));
#54039=CARTESIAN_POINT('Origin',(17.28,9.00000000000001,-77.4));
#54040=CARTESIAN_POINT('',(23.2,9.00000000000001,-74.9));
#54041=CARTESIAN_POINT('',(23.2,9.00000000000001,-74.9));
#54042=CARTESIAN_POINT('Origin',(23.2,9.00000000000001,-77.4));
#54043=CARTESIAN_POINT('Origin',(-23.2,9.00000000000001,-77.4));
#54044=CARTESIAN_POINT('',(-17.28,9.00000000000001,-79.9));
#54045=CARTESIAN_POINT('Origin',(-17.28,9.00000000000001,-77.4));
#54046=CARTESIAN_POINT('',(-23.2,9.00000000000001,-79.9));
#54047=CARTESIAN_POINT('',(-23.2,9.00000000000001,-79.9));
#54048=CARTESIAN_POINT('Origin',(-23.2,9.00000000000001,-77.4));
#54049=CARTESIAN_POINT('Origin',(-1.54689479616415E-14,13.,-76.7));
#54050=CARTESIAN_POINT('',(3.64999999999998,13.,-76.7));
#54051=CARTESIAN_POINT('Origin',(-1.54689479616415E-14,13.,-76.7));
#54052=CARTESIAN_POINT('',(3.64999999999998,13.8,-76.7));
#54053=CARTESIAN_POINT('',(3.64999999999998,13.,-76.7));
#54054=CARTESIAN_POINT('Origin',(-1.65097820472275E-14,13.8,-76.7));
#54055=CARTESIAN_POINT('Origin',(17.28,9.00000000000001,-77.4));
#54056=CARTESIAN_POINT('',(15.7778484524311,9.,-77.4));
#54057=CARTESIAN_POINT('',(17.28,9.00000000000001,-74.9));
#54058=CARTESIAN_POINT('Origin',(-17.28,9.00000000000001,-77.4));
#54059=CARTESIAN_POINT('',(-15.7778484524311,9.,-77.4));
#54060=CARTESIAN_POINT('',(-17.28,9.00000000000001,-79.9));
#54061=CARTESIAN_POINT('Origin',(28.5,14.,-64.9));
#54062=CARTESIAN_POINT('',(28.5,0.500000000000005,-68.2235));
#54063=CARTESIAN_POINT('Origin',(28.5,0.500000000000006,-64.9));
#54064=CARTESIAN_POINT('',(28.5,14.,-68.2235));
#54065=CARTESIAN_POINT('',(28.5,14.,-68.2235));
#54066=CARTESIAN_POINT('Origin',(28.5,14.,-64.9));
#54067=CARTESIAN_POINT('Origin',(28.5,14.,-19.9));
#54068=CARTESIAN_POINT('',(28.5,0.500000000000005,-23.2235));
#54069=CARTESIAN_POINT('Origin',(28.5,0.500000000000006,-19.9));
#54070=CARTESIAN_POINT('',(28.5,14.,-23.2235));
#54071=CARTESIAN_POINT('',(28.5,14.,-23.2235));
#54072=CARTESIAN_POINT('Origin',(28.5,14.,-19.9));
#54073=CARTESIAN_POINT('Origin',(-28.5,14.,-64.9));
#54074=CARTESIAN_POINT('',(-28.5,0.500000000000005,-68.2235));
#54075=CARTESIAN_POINT('Origin',(-28.5,0.500000000000006,-64.9));
#54076=CARTESIAN_POINT('',(-28.5,14.,-68.2235));
#54077=CARTESIAN_POINT('',(-28.5,14.,-68.2235));
#54078=CARTESIAN_POINT('Origin',(-28.5,14.,-64.9));
#54079=CARTESIAN_POINT('Origin',(-28.5,14.,-19.9));
#54080=CARTESIAN_POINT('',(-28.5,0.500000000000003,-23.2235));
#54081=CARTESIAN_POINT('Origin',(-28.5,0.500000000000004,-19.9));
#54082=CARTESIAN_POINT('',(-28.5,14.,-23.2235));
#54083=CARTESIAN_POINT('',(-28.5,14.,-23.2235));
#54084=CARTESIAN_POINT('Origin',(-28.5,14.,-19.9));
#54085=CARTESIAN_POINT('Origin',(-23.2,9.00000000000001,-7.4));
#54086=CARTESIAN_POINT('',(-17.28,9.00000000000001,-9.9));
#54087=CARTESIAN_POINT('Origin',(-17.28,9.00000000000001,-7.4));
#54088=CARTESIAN_POINT('',(-23.2,9.00000000000001,-9.9));
#54089=CARTESIAN_POINT('',(-23.2,9.00000000000001,-9.9));
#54090=CARTESIAN_POINT('Origin',(-23.2,9.00000000000001,-7.4));
#54091=CARTESIAN_POINT('Origin',(23.2,9.00000000000001,-7.4));
#54092=CARTESIAN_POINT('',(17.28,9.00000000000001,-4.90000000000001));
#54093=CARTESIAN_POINT('Origin',(17.28,9.00000000000001,-7.4));
#54094=CARTESIAN_POINT('',(23.2,9.00000000000001,-4.90000000000001));
#54095=CARTESIAN_POINT('',(23.2,9.00000000000001,-4.90000000000001));
#54096=CARTESIAN_POINT('Origin',(23.2,9.00000000000001,-7.4));
#54097=CARTESIAN_POINT('Origin',(-1.54689479616415E-14,13.,-8.1));
#54098=CARTESIAN_POINT('',(3.64999999999998,13.,-8.1));
#54099=CARTESIAN_POINT('Origin',(-1.54689479616415E-14,13.,-8.1));
#54100=CARTESIAN_POINT('',(3.64999999999998,13.8,-8.1));
#54101=CARTESIAN_POINT('',(3.64999999999998,13.,-8.1));
#54102=CARTESIAN_POINT('Origin',(-1.65097820472275E-14,13.8,-8.1));
#54103=CARTESIAN_POINT('Origin',(-1.90276438129354E-14,12.7,-74.2));
#54104=CARTESIAN_POINT('',(0.499999999999987,12.5,-74.2));
#54105=CARTESIAN_POINT('Origin',(-1.87674352915389E-14,12.5,-74.2));
#54106=CARTESIAN_POINT('',(0.499999999999987,12.7,-74.2));
#54107=CARTESIAN_POINT('',(0.499999999999987,12.7,-74.2));
#54108=CARTESIAN_POINT('',(-0.500000000000023,12.7,-74.2));
#54109=CARTESIAN_POINT('Origin',(-1.90276438129354E-14,12.7,-74.2));
#54110=CARTESIAN_POINT('',(-0.500000000000025,13.,-74.2));
#54111=CARTESIAN_POINT('',(-0.500000000000025,12.7,-74.2));
#54112=CARTESIAN_POINT('',(0.499999999999986,13.,-74.2));
#54113=CARTESIAN_POINT('Origin',(-1.94179565950302E-14,13.,-74.2));
#54114=CARTESIAN_POINT('',(0.499999999999987,12.7,-74.2));
#54115=CARTESIAN_POINT('Origin',(-17.28,9.00000000000001,-7.4));
#54116=CARTESIAN_POINT('',(-15.7778484524311,9.,-7.4));
#54117=CARTESIAN_POINT('',(-17.28,9.00000000000001,-9.9));
#54118=CARTESIAN_POINT('Origin',(17.28,9.00000000000001,-7.4));
#54119=CARTESIAN_POINT('',(15.7778484524311,9.,-7.4));
#54120=CARTESIAN_POINT('',(17.28,9.00000000000001,-4.90000000000001));
#54121=CARTESIAN_POINT('Origin',(-1.65232411086791E-14,12.7,-10.6));
#54122=CARTESIAN_POINT('',(0.499999999999984,12.5,-10.6));
#54123=CARTESIAN_POINT('Origin',(-1.62630325872826E-14,12.5,-10.6));
#54124=CARTESIAN_POINT('',(0.499999999999984,12.7,-10.6));
#54125=CARTESIAN_POINT('',(0.499999999999984,12.7,-10.6));
#54126=CARTESIAN_POINT('',(0.499999999999983,13.,-10.6));
#54127=CARTESIAN_POINT('',(0.499999999999984,12.7,-10.6));
#54128=CARTESIAN_POINT('',(-0.500000000000017,13.,-10.6));
#54129=CARTESIAN_POINT('Origin',(-1.69135538907739E-14,13.,-10.6));
#54130=CARTESIAN_POINT('',(-0.500000000000017,12.7,-10.6));
#54131=CARTESIAN_POINT('',(-0.500000000000017,12.7,-10.6));
#54132=CARTESIAN_POINT('Origin',(-1.65232411086791E-14,12.7,-10.6));
#54133=CARTESIAN_POINT('Ctrl Pts',(4.,8.,-84.5));
#54134=CARTESIAN_POINT('Ctrl Pts',(4.,4.,-84.5));
#54135=CARTESIAN_POINT('Ctrl Pts',(0.,4.,-84.5));
#54136=CARTESIAN_POINT('Ctrl Pts',(-4.,4.,-84.5));
#54137=CARTESIAN_POINT('Ctrl Pts',(-4.,8.,-84.5));
#54138=CARTESIAN_POINT('Ctrl Pts',(-4.,12.,-84.5));
#54139=CARTESIAN_POINT('Ctrl Pts',(0.,12.,-84.5));
#54140=CARTESIAN_POINT('Ctrl Pts',(4.,12.,-84.5));
#54141=CARTESIAN_POINT('Ctrl Pts',(4.,8.,-84.5));
#54142=CARTESIAN_POINT('Ctrl Pts',(4.,8.,-86.5172334444062));
#54143=CARTESIAN_POINT('Ctrl Pts',(4.,4.,-86.5172334444062));
#54144=CARTESIAN_POINT('Ctrl Pts',(0.,4.,-86.5172334444062));
#54145=CARTESIAN_POINT('Ctrl Pts',(-4.,4.,-86.5172334444062));
#54146=CARTESIAN_POINT('Ctrl Pts',(-4.,8.,-86.5172334444062));
#54147=CARTESIAN_POINT('Ctrl Pts',(-4.,12.,-86.5172334444062));
#54148=CARTESIAN_POINT('Ctrl Pts',(0.,12.,-86.5172334444062));
#54149=CARTESIAN_POINT('Ctrl Pts',(4.,12.,-86.5172334444062));
#54150=CARTESIAN_POINT('Ctrl Pts',(4.,8.,-86.5172334444062));
#54151=CARTESIAN_POINT('Ctrl Pts',(2.,8.,-86.7803508501983));
#54152=CARTESIAN_POINT('Ctrl Pts',(2.,6.,-86.7803508501983));
#54153=CARTESIAN_POINT('Ctrl Pts',(0.,6.,-86.7803508501983));
#54154=CARTESIAN_POINT('Ctrl Pts',(-2.,6.,-86.7803508501983));
#54155=CARTESIAN_POINT('Ctrl Pts',(-2.,8.,-86.7803508501983));
#54156=CARTESIAN_POINT('Ctrl Pts',(-2.,10.,-86.7803508501983));
#54157=CARTESIAN_POINT('Ctrl Pts',(0.,10.,-86.7803508501983));
#54158=CARTESIAN_POINT('Ctrl Pts',(2.,10.,-86.7803508501983));
#54159=CARTESIAN_POINT('Ctrl Pts',(2.,8.,-86.7803508501983));
#54160=CARTESIAN_POINT('',(-1.15470053837925,6.,-86.7177985317981));
#54161=CARTESIAN_POINT('',(-2.3094010767585,8.,-86.7177985317981));
#54162=CARTESIAN_POINT('Ctrl Pts',(-1.15470053837925,6.,-86.7177985317981));
#54163=CARTESIAN_POINT('Ctrl Pts',(-1.16052376017366,6.01008611601166,-86.7193986219689));
#54164=CARTESIAN_POINT('Ctrl Pts',(-1.16635206467311,6.02018103552669,-86.7209572835343));
#54165=CARTESIAN_POINT('Ctrl Pts',(-1.36167110655042,6.35848353974387,-86.7717992509189));
#54166=CARTESIAN_POINT('Ctrl Pts',(-1.5557141858025,6.69457601186558,-86.7803508501983));
#54167=CARTESIAN_POINT('Ctrl Pts',(-1.90838742933526,7.30542398813443,-86.7803508501983));
#54168=CARTESIAN_POINT('Ctrl Pts',(-2.10243050858733,7.64151646025614,-86.7717992509189));
#54169=CARTESIAN_POINT('Ctrl Pts',(-2.29774955046464,7.97981896447331,-86.7209572835343));
#54170=CARTESIAN_POINT('Ctrl Pts',(-2.3035778549641,7.98991388398835,-86.7193986219689));
#54171=CARTESIAN_POINT('Ctrl Pts',(-2.30940107675851,8.00000000000001,-86.7177985317981));
#54172=CARTESIAN_POINT('',(1.15470053837925,6.,-86.7177985317981));
#54173=CARTESIAN_POINT('Ctrl Pts',(1.15470053837925,6.,-86.7177985317981));
#54174=CARTESIAN_POINT('Ctrl Pts',(1.14305409479044,6.,-86.7193986219689));
#54175=CARTESIAN_POINT('Ctrl Pts',(1.13139748579153,6.,-86.7209572835343));
#54176=CARTESIAN_POINT('Ctrl Pts',(0.740759402036912,6.,-86.7717992509189));
#54177=CARTESIAN_POINT('Ctrl Pts',(0.352673243532761,6.,-86.7803508501983));
#54178=CARTESIAN_POINT('Ctrl Pts',(-0.352673243532758,6.,-86.7803508501983));
#54179=CARTESIAN_POINT('Ctrl Pts',(-0.740759402036907,6.,-86.7717992509189));
#54180=CARTESIAN_POINT('Ctrl Pts',(-1.13139748579153,6.,-86.7209572835343));
#54181=CARTESIAN_POINT('Ctrl Pts',(-1.14305409479043,6.,-86.7193986219689));
#54182=CARTESIAN_POINT('Ctrl Pts',(-1.15470053837925,6.,-86.7177985317981));
#54183=CARTESIAN_POINT('',(2.3094010767585,8.,-86.7177985317981));
#54184=CARTESIAN_POINT('Ctrl Pts',(2.3094010767585,8.,-86.7177985317981));
#54185=CARTESIAN_POINT('Ctrl Pts',(2.30357785496409,7.98991388398834,-86.7193986219689));
#54186=CARTESIAN_POINT('Ctrl Pts',(2.29774955046465,7.97981896447331,-86.7209572835343));
#54187=CARTESIAN_POINT('Ctrl Pts',(2.10243050858733,7.64151646025614,-86.7717992509189));
#54188=CARTESIAN_POINT('Ctrl Pts',(1.90838742933526,7.30542398813443,-86.7803508501983));
#54189=CARTESIAN_POINT('Ctrl Pts',(1.5557141858025,6.69457601186558,-86.7803508501983));
#54190=CARTESIAN_POINT('Ctrl Pts',(1.36167110655042,6.35848353974387,-86.7717992509189));
#54191=CARTESIAN_POINT('Ctrl Pts',(1.16635206467311,6.02018103552669,-86.7209572835344));
#54192=CARTESIAN_POINT('Ctrl Pts',(1.16052376017366,6.01008611601166,-86.7193986219689));
#54193=CARTESIAN_POINT('Ctrl Pts',(1.15470053837925,6.00000000000001,-86.7177985317981));
#54194=CARTESIAN_POINT('',(4.,8.,-84.5));
#54195=CARTESIAN_POINT('Ctrl Pts',(2.3094010767585,8.,-86.7177985317981));
#54196=CARTESIAN_POINT('Ctrl Pts',(4.,8.,-86.2532600313803));
#54197=CARTESIAN_POINT('Ctrl Pts',(4.,8.,-84.5));
#54198=CARTESIAN_POINT('',(-4.,8.,-84.5));
#54199=CARTESIAN_POINT('Origin',(0.,8.,-84.5));
#54200=CARTESIAN_POINT('Origin',(0.,8.,-84.5));
#54201=CARTESIAN_POINT('',(1.15470053837925,10.,-86.7177985317981));
#54202=CARTESIAN_POINT('Ctrl Pts',(1.15470053837925,10.,-86.7177985317981));
#54203=CARTESIAN_POINT('Ctrl Pts',(1.16052376017366,9.98991388398835,-86.7193986219689));
#54204=CARTESIAN_POINT('Ctrl Pts',(1.16635206467311,9.97981896447332,-86.7209572835343));
#54205=CARTESIAN_POINT('Ctrl Pts',(1.36167110655042,9.64151646025614,-86.7717992509189));
#54206=CARTESIAN_POINT('Ctrl Pts',(1.5557141858025,9.30542398813443,-86.7803508501983));
#54207=CARTESIAN_POINT('Ctrl Pts',(1.90838742933526,8.69457601186558,-86.7803508501983));
#54208=CARTESIAN_POINT('Ctrl Pts',(2.10243050858733,8.35848353974387,-86.7717992509189));
#54209=CARTESIAN_POINT('Ctrl Pts',(2.29774955046465,8.02018103552669,-86.7209572835343));
#54210=CARTESIAN_POINT('Ctrl Pts',(2.3035778549641,8.01008611601166,-86.7193986219689));
#54211=CARTESIAN_POINT('Ctrl Pts',(2.30940107675851,8.,-86.7177985317981));
#54212=CARTESIAN_POINT('',(-1.15470053837925,10.,-86.7177985317981));
#54213=CARTESIAN_POINT('Ctrl Pts',(-1.15470053837925,10.,-86.7177985317981));
#54214=CARTESIAN_POINT('Ctrl Pts',(-1.14305409479043,10.,-86.7193986219689));
#54215=CARTESIAN_POINT('Ctrl Pts',(-1.13139748579153,10.,-86.7209572835343));
#54216=CARTESIAN_POINT('Ctrl Pts',(-0.740759402036911,10.,-86.7717992509189));
#54217=CARTESIAN_POINT('Ctrl Pts',(-0.352673243532759,10.,-86.7803508501983));
#54218=CARTESIAN_POINT('Ctrl Pts',(0.352673243532759,10.,-86.7803508501983));
#54219=CARTESIAN_POINT('Ctrl Pts',(0.740759402036911,10.,-86.7717992509189));
#54220=CARTESIAN_POINT('Ctrl Pts',(1.13139748579153,10.,-86.7209572835343));
#54221=CARTESIAN_POINT('Ctrl Pts',(1.14305409479044,10.,-86.7193986219689));
#54222=CARTESIAN_POINT('Ctrl Pts',(1.15470053837925,10.,-86.7177985317981));
#54223=CARTESIAN_POINT('Ctrl Pts',(-2.3094010767585,8.,-86.7177985317981));
#54224=CARTESIAN_POINT('Ctrl Pts',(-2.3035778549641,8.01008611601166,-86.7193986219689));
#54225=CARTESIAN_POINT('Ctrl Pts',(-2.29774955046464,8.02018103552669,-86.7209572835343));
#54226=CARTESIAN_POINT('Ctrl Pts',(-2.10243050858733,8.35848353974387,-86.7717992509189));
#54227=CARTESIAN_POINT('Ctrl Pts',(-1.90838742933526,8.69457601186558,-86.7803508501983));
#54228=CARTESIAN_POINT('Ctrl Pts',(-1.5557141858025,9.30542398813443,-86.7803508501983));
#54229=CARTESIAN_POINT('Ctrl Pts',(-1.36167110655042,9.64151646025614,-86.7717992509189));
#54230=CARTESIAN_POINT('Ctrl Pts',(-1.16635206467311,9.97981896447332,-86.7209572835343));
#54231=CARTESIAN_POINT('Ctrl Pts',(-1.16052376017366,9.98991388398835,-86.7193986219689));
#54232=CARTESIAN_POINT('Ctrl Pts',(-1.15470053837925,10.,-86.7177985317981));
#54233=CARTESIAN_POINT('Origin',(0.,8.,-86.8));
#54234=CARTESIAN_POINT('',(-4.,8.,-83.8));
#54235=CARTESIAN_POINT('Origin',(0.,8.,-83.8));
#54236=CARTESIAN_POINT('',(-4.,8.,-86.8));
#54237=CARTESIAN_POINT('Origin',(0.,8.,-83.8));
#54238=CARTESIAN_POINT('',(4.99995,8.,-83.8));
#54239=CARTESIAN_POINT('Origin',(0.,8.,-83.8));
#54240=CARTESIAN_POINT('',(4.99995,8.,-84.8));
#54241=CARTESIAN_POINT('',(4.99995,8.,-83.8));
#54242=CARTESIAN_POINT('Origin',(0.,8.,-84.8));
#54243=CARTESIAN_POINT('Origin',(25.4958861827765,-14.55,-104.175753233145));
#54244=CARTESIAN_POINT('',(23.,-16.5,-64.9));
#54245=CARTESIAN_POINT('',(25.4958861827765,-14.55,-69.5070923773207));
#54246=CARTESIAN_POINT('Origin',(28.4999999999971,-12.2029290542153,-64.9000000000014));
#54247=CARTESIAN_POINT('',(23.,-16.5,-71.4));
#54248=CARTESIAN_POINT('',(23.,-16.5,-84.8));
#54249=CARTESIAN_POINT('',(25.4958861827765,-14.55,-71.4));
#54250=CARTESIAN_POINT('',(25.4958861827765,-14.55,-71.4));
#54251=CARTESIAN_POINT('',(25.4958861827765,-14.55,-104.175753233145));
#54252=CARTESIAN_POINT('Origin',(25.4958861827765,-14.55,-104.175753233145));
#54253=CARTESIAN_POINT('',(25.4958861827765,-14.55,-60.2929076226793));
#54254=CARTESIAN_POINT('Origin',(28.5000000000002,-12.2029290542129,-64.9000000000003));
#54255=CARTESIAN_POINT('',(25.4958861827765,-14.55,-24.5070923773207));
#54256=CARTESIAN_POINT('',(25.4958861827765,-14.55,-104.175753233145));
#54257=CARTESIAN_POINT('',(23.,-16.5,-19.9));
#54258=CARTESIAN_POINT('Origin',(28.4999999999964,-12.2029290542158,-19.900000000002));
#54259=CARTESIAN_POINT('',(23.,-16.5,-84.8));
#54260=CARTESIAN_POINT('Origin',(-25.4958861827765,-14.55,-104.175753233145));
#54261=CARTESIAN_POINT('',(-23.,-16.5,-64.9));
#54262=CARTESIAN_POINT('',(-25.4958861827765,-14.55,-60.2929076226793));
#54263=CARTESIAN_POINT('Origin',(-28.5000000000003,-12.2029290542127,-64.9000000000003));
#54264=CARTESIAN_POINT('',(-23.,-16.5,-19.9));
#54265=CARTESIAN_POINT('',(-23.,-16.5,-84.8));
#54266=CARTESIAN_POINT('',(-25.4958861827765,-14.55,-24.5070923773207));
#54267=CARTESIAN_POINT('Origin',(-28.4999999999988,-12.2029290542139,-19.9000000000006));
#54268=CARTESIAN_POINT('',(-25.4958861827765,-14.55,-104.175753233145));
#54269=CARTESIAN_POINT('Origin',(-25.4958861827765,-14.55,-104.175753233145));
#54270=CARTESIAN_POINT('',(-25.4958861827765,-14.55,-15.2929076226793));
#54271=CARTESIAN_POINT('Origin',(-28.4999999999998,-12.2029290542132,-19.8999999999999));
#54272=CARTESIAN_POINT('',(-23.,-16.5,-13.4));
#54273=CARTESIAN_POINT('',(-23.,-16.5,-84.8));
#54274=CARTESIAN_POINT('',(-25.4958861827765,-14.55,-13.4));
#54275=CARTESIAN_POINT('',(-25.4958861827765,-14.55,-13.4));
#54276=CARTESIAN_POINT('',(-25.4958861827765,-14.55,-104.175753233145));
#54277=CARTESIAN_POINT('Origin',(8.05,-8.2,-84.8));
#54278=CARTESIAN_POINT('',(8.57259699813413,-7.67740300186587,-81.35));
#54279=CARTESIAN_POINT('',(8.19644660940673,-8.05355339059327,-81.35));
#54280=CARTESIAN_POINT('',(8.57259699813413,-7.67740300186587,-81.35));
#54281=CARTESIAN_POINT('',(8.57259699813413,-7.67740300186587,-84.8));
#54282=CARTESIAN_POINT('',(8.57259699813413,-7.67740300186587,-84.8));
#54283=CARTESIAN_POINT('',(8.19644660940673,-8.05355339059327,-84.8));
#54284=CARTESIAN_POINT('',(8.05,-8.2,-84.8));
#54285=CARTESIAN_POINT('',(8.19644660940673,-8.05355339059327,-84.8));
#54286=CARTESIAN_POINT('Origin',(8.05,3.67394039744206E-16,-84.8));
#54287=CARTESIAN_POINT('',(10.9824030018659,-2.93240300186586,-81.35));
#54288=CARTESIAN_POINT('',(11.3535533905933,-3.30355339059329,-81.35));
#54289=CARTESIAN_POINT('',(10.9824030018659,-2.93240300186586,-81.35));
#54290=CARTESIAN_POINT('',(10.9824030018659,-2.93240300186586,-84.8));
#54291=CARTESIAN_POINT('',(10.9824030018659,-2.93240300186586,-84.8));
#54292=CARTESIAN_POINT('',(11.3535533905933,-3.30355339059329,-84.8));
#54293=CARTESIAN_POINT('',(8.05,3.67394039744206E-16,-84.8));
#54294=CARTESIAN_POINT('',(11.3535533905933,-3.30355339059329,0.));
#54295=CARTESIAN_POINT('Origin',(-8.05,-8.2,-84.8));
#54296=CARTESIAN_POINT('',(-10.9824030018659,-5.26759699813413,-81.35));
#54297=CARTESIAN_POINT('',(-11.3535533905933,-4.89644660940674,-81.35));
#54298=CARTESIAN_POINT('',(-10.9824030018659,-5.26759699813413,-81.35));
#54299=CARTESIAN_POINT('',(-10.9824030018659,-5.26759699813413,-84.8));
#54300=CARTESIAN_POINT('',(-10.9824030018659,-5.26759699813413,-84.8));
#54301=CARTESIAN_POINT('',(-11.3535533905933,-4.89644660940674,-84.8));
#54302=CARTESIAN_POINT('',(-8.05,-8.2,-84.8));
#54303=CARTESIAN_POINT('',(-11.3535533905933,-4.89644660940674,0.));
#54304=CARTESIAN_POINT('Origin',(-8.05,-1.60428730688303E-15,-84.8));
#54305=CARTESIAN_POINT('',(-8.57259699813413,-0.522596998134137,-81.35));
#54306=CARTESIAN_POINT('',(-8.05,-1.60428730688303E-15,-81.35));
#54307=CARTESIAN_POINT('',(-8.57259699813413,-0.522596998134137,-81.35));
#54308=CARTESIAN_POINT('',(-8.57259699813413,-0.522596998134137,-84.8));
#54309=CARTESIAN_POINT('',(-8.57259699813413,-0.522596998134137,-84.8));
#54310=CARTESIAN_POINT('',(-8.05,-1.60428730688303E-15,-84.8));
#54311=CARTESIAN_POINT('',(-8.05,-1.60428730688303E-15,-84.8));
#54312=CARTESIAN_POINT('',(-8.05,-1.60428730688303E-15,-84.8));
#54313=CARTESIAN_POINT('Origin',(-8.05,-1.60428730688303E-15,-84.8));
#54314=CARTESIAN_POINT('',(-11.3535533905933,-3.30355339059329,-81.35));
#54315=CARTESIAN_POINT('',(-10.9824030018659,-2.93240300186587,-81.35));
#54316=CARTESIAN_POINT('',(-11.3535533905933,-3.30355339059329,-81.35));
#54317=CARTESIAN_POINT('',(-11.3535533905933,-3.30355339059329,-84.8));
#54318=CARTESIAN_POINT('',(-11.3535533905933,-3.30355339059329,-84.8));
#54319=CARTESIAN_POINT('',(-10.9824030018659,-2.93240300186587,-84.8));
#54320=CARTESIAN_POINT('',(-8.05,-1.60428730688303E-15,-84.8));
#54321=CARTESIAN_POINT('',(-10.9824030018659,-2.93240300186587,0.));
#54322=CARTESIAN_POINT('Origin',(-11.5,-4.75000000000001,-84.8));
#54323=CARTESIAN_POINT('',(-11.5,-4.54289321881346,-81.35));
#54324=CARTESIAN_POINT('',(-11.5,-3.65710678118656,-81.35));
#54325=CARTESIAN_POINT('',(-11.5,-4.54289321881346,-81.35));
#54326=CARTESIAN_POINT('',(-11.5,-4.54289321881346,-84.8));
#54327=CARTESIAN_POINT('',(-11.5,-4.54289321881346,-84.8));
#54328=CARTESIAN_POINT('',(-11.5,-3.65710678118656,-84.8));
#54329=CARTESIAN_POINT('',(-11.5,-4.75000000000001,-84.8));
#54330=CARTESIAN_POINT('',(-11.5,-3.65710678118656,0.));
#54331=CARTESIAN_POINT('Origin',(-8.05,-8.2,-84.8));
#54332=CARTESIAN_POINT('',(-8.19644660940673,-8.05355339059327,-81.35));
#54333=CARTESIAN_POINT('',(-8.57259699813413,-7.67740300186587,-81.35));
#54334=CARTESIAN_POINT('',(-8.19644660940673,-8.05355339059327,-81.35));
#54335=CARTESIAN_POINT('',(-8.19644660940673,-8.05355339059327,-84.8));
#54336=CARTESIAN_POINT('',(-8.19644660940673,-8.05355339059327,-84.8));
#54337=CARTESIAN_POINT('',(-8.57259699813413,-7.67740300186587,-84.8));
#54338=CARTESIAN_POINT('',(-8.05,-8.2,-84.8));
#54339=CARTESIAN_POINT('',(-8.57259699813413,-7.67740300186587,0.));
#54340=CARTESIAN_POINT('Origin',(-8.05,-12.24,-84.8));
#54341=CARTESIAN_POINT('',(-8.05,-12.0328932188134,-81.35));
#54342=CARTESIAN_POINT('',(-8.05,-8.40710678118654,-81.35));
#54343=CARTESIAN_POINT('',(-8.05,-12.0328932188134,-81.35));
#54344=CARTESIAN_POINT('',(-8.05,-12.0328932188134,-84.8));
#54345=CARTESIAN_POINT('',(-8.05,-12.0328932188134,-84.8));
#54346=CARTESIAN_POINT('',(-8.05,-8.40710678118654,-84.8));
#54347=CARTESIAN_POINT('',(-8.05,-12.24,-84.8));
#54348=CARTESIAN_POINT('',(-8.05,-8.40710678118654,-84.8));
#54349=CARTESIAN_POINT('Origin',(-12.31,-16.5,-84.8));
#54350=CARTESIAN_POINT('',(-12.31,-16.5,-81.35));
#54351=CARTESIAN_POINT('',(-8.19644660940672,-12.3864466094067,-81.35));
#54352=CARTESIAN_POINT('',(-12.31,-16.5,-81.35));
#54353=CARTESIAN_POINT('',(-12.31,-16.5,-84.8));
#54354=CARTESIAN_POINT('',(-12.31,-16.5,-84.8));
#54355=CARTESIAN_POINT('',(-8.19644660940672,-12.3864466094067,-84.8));
#54356=CARTESIAN_POINT('',(-12.31,-16.5,-84.8));
#54357=CARTESIAN_POINT('',(-8.19644660940672,-12.3864466094067,-84.8));
#54358=CARTESIAN_POINT('Origin',(-23.,-16.5,-84.8));
#54359=CARTESIAN_POINT('',(-22.2,-16.5,-81.35));
#54360=CARTESIAN_POINT('',(-22.2,-16.5,-81.35));
#54361=CARTESIAN_POINT('',(-22.2,-16.5,-84.8));
#54362=CARTESIAN_POINT('',(-22.2,-16.5,-84.8));
#54363=CARTESIAN_POINT('',(-23.,-16.5,-84.8));
#54364=CARTESIAN_POINT('Origin',(12.31,-16.5,-84.8));
#54365=CARTESIAN_POINT('',(12.31,-16.5,-81.35));
#54366=CARTESIAN_POINT('',(22.2,-16.5,-81.35));
#54367=CARTESIAN_POINT('',(12.31,-16.5,-81.35));
#54368=CARTESIAN_POINT('',(12.31,-16.5,-84.8));
#54369=CARTESIAN_POINT('',(12.31,-16.5,-84.8));
#54370=CARTESIAN_POINT('',(22.2,-16.5,-84.8));
#54371=CARTESIAN_POINT('',(12.31,-16.5,-84.8));
#54372=CARTESIAN_POINT('',(22.2,-16.5,-84.8));
#54373=CARTESIAN_POINT('Origin',(12.31,-16.5,-84.8));
#54374=CARTESIAN_POINT('',(8.19644660940673,-12.3864466094067,-81.35));
#54375=CARTESIAN_POINT('',(8.19644660940673,-12.3864466094067,-81.35));
#54376=CARTESIAN_POINT('',(8.19644660940673,-12.3864466094067,-84.8));
#54377=CARTESIAN_POINT('',(8.19644660940673,-12.3864466094067,-84.8));
#54378=CARTESIAN_POINT('',(12.31,-16.5,-84.8));
#54379=CARTESIAN_POINT('Origin',(8.05,-12.24,-84.8));
#54380=CARTESIAN_POINT('',(8.05,-8.40710678118654,-81.35));
#54381=CARTESIAN_POINT('',(8.05,-12.0328932188134,-81.35));
#54382=CARTESIAN_POINT('',(8.05,-8.40710678118654,-81.35));
#54383=CARTESIAN_POINT('',(8.05,-8.40710678118654,-84.8));
#54384=CARTESIAN_POINT('',(8.05,-8.40710678118654,-84.8));
#54385=CARTESIAN_POINT('',(8.05,-12.0328932188134,-84.8));
#54386=CARTESIAN_POINT('',(8.05,-12.24,-84.8));
#54387=CARTESIAN_POINT('',(8.05,-12.0328932188134,-84.8));
#54388=CARTESIAN_POINT('Origin',(8.05,-8.2,-84.8));
#54389=CARTESIAN_POINT('',(11.3535533905933,-4.89644660940673,-81.35));
#54390=CARTESIAN_POINT('',(10.9824030018659,-5.26759699813413,-81.35));
#54391=CARTESIAN_POINT('',(11.3535533905933,-4.89644660940673,-81.35));
#54392=CARTESIAN_POINT('',(11.3535533905933,-4.89644660940673,-84.8));
#54393=CARTESIAN_POINT('',(11.3535533905933,-4.89644660940673,-84.8));
#54394=CARTESIAN_POINT('',(10.9824030018659,-5.26759699813413,-84.8));
#54395=CARTESIAN_POINT('',(8.05,-8.2,-84.8));
#54396=CARTESIAN_POINT('',(10.9824030018659,-5.26759699813413,0.));
#54397=CARTESIAN_POINT('Origin',(11.5,-4.75000000000001,-84.8));
#54398=CARTESIAN_POINT('',(11.5,-3.65710678118656,-81.35));
#54399=CARTESIAN_POINT('',(11.5,-4.54289321881346,-81.35));
#54400=CARTESIAN_POINT('',(11.5,-3.65710678118656,-81.35));
#54401=CARTESIAN_POINT('',(11.5,-3.65710678118656,-84.8));
#54402=CARTESIAN_POINT('',(11.5,-3.65710678118656,-84.8));
#54403=CARTESIAN_POINT('',(11.5,-4.54289321881346,-84.8));
#54404=CARTESIAN_POINT('',(11.5,-4.75000000000001,-84.8));
#54405=CARTESIAN_POINT('',(11.5,-4.54289321881346,0.));
#54406=CARTESIAN_POINT('Origin',(8.05,3.67394039744206E-16,-84.8));
#54407=CARTESIAN_POINT('',(8.05,3.67394039744206E-16,-81.35));
#54408=CARTESIAN_POINT('',(8.57259699813413,-0.522596998134133,-81.35));
#54409=CARTESIAN_POINT('',(8.05,3.67394039744206E-16,-81.35));
#54410=CARTESIAN_POINT('',(8.05,3.67394039744206E-16,-84.8));
#54411=CARTESIAN_POINT('',(8.05,3.67394039744206E-16,-84.8));
#54412=CARTESIAN_POINT('',(8.57259699813413,-0.522596998134133,-84.8));
#54413=CARTESIAN_POINT('',(8.05,3.67394039744206E-16,-84.8));
#54414=CARTESIAN_POINT('',(8.57259699813413,-0.522596998134133,0.));
#54415=CARTESIAN_POINT('Origin',(8.05,3.67394039744206E-16,-84.8));
#54416=CARTESIAN_POINT('',(-8.05,-1.60428730688303E-15,-81.35));
#54417=CARTESIAN_POINT('',(8.05,3.67394039744206E-16,-84.8));
#54418=CARTESIAN_POINT('Origin',(-10.995,-0.510000000000002,-84.8));
#54419=CARTESIAN_POINT('',(-10.6942336092596,-2.79024989380572,-81.35));
#54420=CARTESIAN_POINT('',(-8.71475010619428,-0.810766390740372,-81.35));
#54421=CARTESIAN_POINT('Origin',(-10.995,-0.510000000000002,-81.35));
#54422=CARTESIAN_POINT('',(-10.6942336092596,-2.79024989380572,-84.8));
#54423=CARTESIAN_POINT('',(-10.6942336092596,-2.79024989380572,-84.8));
#54424=CARTESIAN_POINT('',(-8.71475010619428,-0.810766390740372,-84.8));
#54425=CARTESIAN_POINT('Origin',(-10.995,-0.510000000000002,-84.8));
#54426=CARTESIAN_POINT('',(-8.71475010619428,-0.810766390740372,-84.8));
#54427=CARTESIAN_POINT('Origin',(-10.995,-7.69,-84.8));
#54428=CARTESIAN_POINT('',(-8.71475010619428,-7.38923360925963,-81.35));
#54429=CARTESIAN_POINT('',(-10.6942336092596,-5.40975010619428,-81.35));
#54430=CARTESIAN_POINT('Origin',(-10.995,-7.69,-81.35));
#54431=CARTESIAN_POINT('',(-8.71475010619428,-7.38923360925963,-84.8));
#54432=CARTESIAN_POINT('',(-8.71475010619428,-7.38923360925963,-84.8));
#54433=CARTESIAN_POINT('',(-10.6942336092596,-5.40975010619428,-84.8));
#54434=CARTESIAN_POINT('Origin',(-10.995,-7.69,-84.8));
#54435=CARTESIAN_POINT('',(-10.6942336092596,-5.40975010619428,-84.8));
#54436=CARTESIAN_POINT('Origin',(10.995,-0.509999999999999,-84.8));
#54437=CARTESIAN_POINT('',(8.71475010619428,-0.81076639074037,-81.35));
#54438=CARTESIAN_POINT('',(10.6942336092596,-2.79024989380572,-81.35));
#54439=CARTESIAN_POINT('Origin',(10.995,-0.509999999999999,-81.35));
#54440=CARTESIAN_POINT('',(8.71475010619428,-0.81076639074037,-84.8));
#54441=CARTESIAN_POINT('',(8.71475010619428,-0.81076639074037,-84.8));
#54442=CARTESIAN_POINT('',(10.6942336092596,-2.79024989380572,-84.8));
#54443=CARTESIAN_POINT('Origin',(10.995,-0.509999999999999,-84.8));
#54444=CARTESIAN_POINT('',(10.6942336092596,-2.79024989380572,-84.8));
#54445=CARTESIAN_POINT('Origin',(10.995,-7.69,-84.8));
#54446=CARTESIAN_POINT('',(10.6942336092596,-5.40975010619428,-81.35));
#54447=CARTESIAN_POINT('',(8.71475010619428,-7.38923360925963,-81.35));
#54448=CARTESIAN_POINT('Origin',(10.995,-7.69,-81.35));
#54449=CARTESIAN_POINT('',(10.6942336092596,-5.40975010619428,-84.8));
#54450=CARTESIAN_POINT('',(10.6942336092596,-5.40975010619428,-84.8));
#54451=CARTESIAN_POINT('',(8.71475010619428,-7.38923360925963,-84.8));
#54452=CARTESIAN_POINT('Origin',(10.995,-7.69,-84.8));
#54453=CARTESIAN_POINT('',(8.71475010619428,-7.38923360925963,-84.8));
#54454=CARTESIAN_POINT('Origin',(8.55,-12.0328932188134,-84.8));
#54455=CARTESIAN_POINT('Origin',(8.55,-12.0328932188134,-81.35));
#54456=CARTESIAN_POINT('Origin',(8.55,-12.0328932188134,-84.8));
#54457=CARTESIAN_POINT('Origin',(-8.55,-12.0328932188134,-84.8));
#54458=CARTESIAN_POINT('Origin',(-8.55,-12.0328932188134,-81.35));
#54459=CARTESIAN_POINT('Origin',(-8.55,-12.0328932188134,-84.8));
#54460=CARTESIAN_POINT('Origin',(11.,-4.54289321881346,-84.8));
#54461=CARTESIAN_POINT('Origin',(11.,-4.54289321881346,-81.35));
#54462=CARTESIAN_POINT('Origin',(11.,-4.54289321881346,-84.8));
#54463=CARTESIAN_POINT('Origin',(11.,-3.65710678118656,-84.8));
#54464=CARTESIAN_POINT('Origin',(11.,-3.65710678118656,-81.35));
#54465=CARTESIAN_POINT('Origin',(11.,-3.65710678118656,-84.8));
#54466=CARTESIAN_POINT('Origin',(10.6288496112726,-3.28595639245914,-84.8));
#54467=CARTESIAN_POINT('Origin',(10.6288496112726,-3.28595639245914,-81.35));
#54468=CARTESIAN_POINT('Origin',(10.6288496112726,-3.28595639245914,-84.8));
#54469=CARTESIAN_POINT('Origin',(8.21904360754086,-0.876150388727407,-84.8));
#54470=CARTESIAN_POINT('Origin',(8.21904360754086,-0.876150388727407,-81.35));
#54471=CARTESIAN_POINT('Origin',(8.21904360754086,-0.876150388727407,-84.8));
#54472=CARTESIAN_POINT('Origin',(10.6288496112726,-4.91404360754086,-84.8));
#54473=CARTESIAN_POINT('Origin',(10.6288496112726,-4.91404360754086,-81.35));
#54474=CARTESIAN_POINT('Origin',(10.6288496112726,-4.91404360754086,-84.8));
#54475=CARTESIAN_POINT('Origin',(8.21904360754086,-7.32384961127259,-84.8));
#54476=CARTESIAN_POINT('Origin',(8.21904360754086,-7.32384961127259,-81.35));
#54477=CARTESIAN_POINT('Origin',(8.21904360754086,-7.32384961127259,-84.8));
#54478=CARTESIAN_POINT('Origin',(8.55,-8.40710678118654,-84.8));
#54479=CARTESIAN_POINT('Origin',(8.55,-8.40710678118654,-81.35));
#54480=CARTESIAN_POINT('Origin',(8.55,-8.40710678118654,-84.8));
#54481=CARTESIAN_POINT('Origin',(-8.55,-8.40710678118654,-84.8));
#54482=CARTESIAN_POINT('Origin',(-8.55,-8.40710678118654,-81.35));
#54483=CARTESIAN_POINT('Origin',(-8.55,-8.40710678118654,-84.8));
#54484=CARTESIAN_POINT('Origin',(-8.21904360754086,-7.32384961127259,-84.8));
#54485=CARTESIAN_POINT('Origin',(-8.21904360754086,-7.32384961127259,-81.35));
#54486=CARTESIAN_POINT('Origin',(-8.21904360754086,-7.32384961127259,-84.8));
#54487=CARTESIAN_POINT('Origin',(-10.6288496112726,-4.91404360754086,-84.8));
#54488=CARTESIAN_POINT('Origin',(-10.6288496112726,-4.91404360754086,-81.35));
#54489=CARTESIAN_POINT('Origin',(-10.6288496112726,-4.91404360754086,-84.8));
#54490=CARTESIAN_POINT('Origin',(-11.,-4.54289321881346,-84.8));
#54491=CARTESIAN_POINT('Origin',(-11.,-4.54289321881346,-81.35));
#54492=CARTESIAN_POINT('Origin',(-11.,-4.54289321881346,-84.8));
#54493=CARTESIAN_POINT('Origin',(-11.,-3.65710678118656,-84.8));
#54494=CARTESIAN_POINT('Origin',(-11.,-3.65710678118656,-81.35));
#54495=CARTESIAN_POINT('Origin',(-11.,-3.65710678118656,-84.8));
#54496=CARTESIAN_POINT('Origin',(-10.6288496112726,-3.28595639245914,-84.8));
#54497=CARTESIAN_POINT('Origin',(-10.6288496112726,-3.28595639245914,-81.35));
#54498=CARTESIAN_POINT('Origin',(-10.6288496112726,-3.28595639245914,-84.8));
#54499=CARTESIAN_POINT('Origin',(-8.21904360754086,-0.87615038872741,-84.8));
#54500=CARTESIAN_POINT('Origin',(-8.21904360754086,-0.87615038872741,-81.35));
#54501=CARTESIAN_POINT('Origin',(-8.21904360754086,-0.87615038872741,-84.8));
#54502=CARTESIAN_POINT('Origin',(0.,8.,-83.8));
#54503=CARTESIAN_POINT('Origin',(-22.2,13.,-84.8));
#54504=CARTESIAN_POINT('',(-22.2,13.,-84.8));
#54505=CARTESIAN_POINT('',(-22.2,13.,-81.35));
#54506=CARTESIAN_POINT('',(-22.2,13.,-84.8));
#54507=CARTESIAN_POINT('',(22.2,13.,-81.35));
#54508=CARTESIAN_POINT('',(22.2,13.,-81.35));
#54509=CARTESIAN_POINT('',(22.2,13.,-84.8));
#54510=CARTESIAN_POINT('',(22.2,13.,-84.8));
#54511=CARTESIAN_POINT('',(-22.2,13.,-84.8));
#54512=CARTESIAN_POINT('Origin',(0.,0.,-84.8));
#54513=CARTESIAN_POINT('',(-23.2,-15.5,-84.8));
#54514=CARTESIAN_POINT('',(-22.2,-16.5,-84.8));
#54515=CARTESIAN_POINT('',(-23.2,12.,-84.8));
#54516=CARTESIAN_POINT('',(-23.2,-15.5,-84.8));
#54517=CARTESIAN_POINT('',(-23.2,12.,-84.8));
#54518=CARTESIAN_POINT('',(23.2,12.,-84.8));
#54519=CARTESIAN_POINT('',(22.2,13.,-84.8));
#54520=CARTESIAN_POINT('',(23.2,-15.5,-84.8));
#54521=CARTESIAN_POINT('',(23.2,12.,-84.8));
#54522=CARTESIAN_POINT('',(23.2,-15.5,-84.8));
#54523=CARTESIAN_POINT('Origin',(-23.2,12.,-84.8));
#54524=CARTESIAN_POINT('',(-23.2,12.,-81.35));
#54525=CARTESIAN_POINT('',(-23.2,12.,-84.8));
#54526=CARTESIAN_POINT('',(-22.2,13.,-81.35));
#54527=CARTESIAN_POINT('Origin',(-23.2,-15.5,-84.8));
#54528=CARTESIAN_POINT('',(-23.2,-15.5,-81.35));
#54529=CARTESIAN_POINT('',(-23.2,-15.5,-84.8));
#54530=CARTESIAN_POINT('',(-23.2,12.,-81.35));
#54531=CARTESIAN_POINT('Origin',(-22.2,-16.5,-84.8));
#54532=CARTESIAN_POINT('',(-23.2,-15.5,-81.35));
#54533=CARTESIAN_POINT('Origin',(23.2,-15.5,-84.8));
#54534=CARTESIAN_POINT('',(23.2,-15.5,-81.35));
#54535=CARTESIAN_POINT('',(23.2,-15.5,-84.8));
#54536=CARTESIAN_POINT('',(22.2,-16.5,-81.35));
#54537=CARTESIAN_POINT('Origin',(23.2,12.,-84.8));
#54538=CARTESIAN_POINT('',(23.2,12.,-81.35));
#54539=CARTESIAN_POINT('',(23.2,12.,-84.8));
#54540=CARTESIAN_POINT('',(23.2,-15.5,-81.35));
#54541=CARTESIAN_POINT('Origin',(22.2,13.,-84.8));
#54542=CARTESIAN_POINT('',(23.2,12.,-81.35));
#54543=CARTESIAN_POINT('Origin',(-2.3094010767585,8.,-84.4));
#54544=CARTESIAN_POINT('',(-2.3094010767585,8.,-84.4));
#54545=CARTESIAN_POINT('',(-2.3094010767585,8.,-84.4));
#54546=CARTESIAN_POINT('',(-1.15470053837925,10.,-84.4));
#54547=CARTESIAN_POINT('',(-1.15470053837925,10.,-84.4));
#54548=CARTESIAN_POINT('',(-2.3094010767585,8.,-84.4));
#54549=CARTESIAN_POINT('Origin',(-1.15470053837925,6.,-84.4));
#54550=CARTESIAN_POINT('',(-1.15470053837925,6.,-84.4));
#54551=CARTESIAN_POINT('',(-1.15470053837925,6.,-84.4));
#54552=CARTESIAN_POINT('',(-1.15470053837925,6.,-84.4));
#54553=CARTESIAN_POINT('Origin',(1.15470053837925,6.,-84.4));
#54554=CARTESIAN_POINT('',(1.15470053837925,6.,-84.4));
#54555=CARTESIAN_POINT('',(1.15470053837925,6.,-84.4));
#54556=CARTESIAN_POINT('',(1.15470053837925,6.,-84.4));
#54557=CARTESIAN_POINT('Origin',(2.3094010767585,8.,-84.4));
#54558=CARTESIAN_POINT('',(2.3094010767585,8.,-84.4));
#54559=CARTESIAN_POINT('',(2.3094010767585,8.,-84.4));
#54560=CARTESIAN_POINT('',(2.3094010767585,8.,-84.4));
#54561=CARTESIAN_POINT('Origin',(1.15470053837925,10.,-84.4));
#54562=CARTESIAN_POINT('',(1.15470053837925,10.,-84.4));
#54563=CARTESIAN_POINT('',(1.15470053837925,10.,-84.4));
#54564=CARTESIAN_POINT('',(1.15470053837925,10.,-84.4));
#54565=CARTESIAN_POINT('Origin',(-1.15470053837925,10.,-84.4));
#54566=CARTESIAN_POINT('',(-1.15470053837925,10.,-84.4));
#54567=CARTESIAN_POINT('Origin',(0.,0.,-84.4));
#54568=CARTESIAN_POINT('Origin',(-8.55,-12.0328932188134,-81.35));
#54569=CARTESIAN_POINT('',(8.23180194846605,-12.3510912703474,-81.35));
#54570=CARTESIAN_POINT('',(12.3307106781187,-16.45,-81.35));
#54571=CARTESIAN_POINT('',(8.23180194846605,-12.3510912703474,-81.35));
#54572=CARTESIAN_POINT('',(8.1,-12.0328932188134,-81.35));
#54573=CARTESIAN_POINT('Origin',(8.55,-12.0328932188134,-81.35));
#54574=CARTESIAN_POINT('',(8.1,-8.40710678118654,-81.35));
#54575=CARTESIAN_POINT('',(8.1,-8.40710678118654,-81.35));
#54576=CARTESIAN_POINT('',(8.23180194846606,-8.08890872965259,-81.35));
#54577=CARTESIAN_POINT('Origin',(8.55,-8.40710678118654,-81.35));
#54578=CARTESIAN_POINT('',(8.60795233719346,-7.71275834092519,-81.35));
#54579=CARTESIAN_POINT('',(8.60795233719346,-7.71275834092519,-81.35));
#54580=CARTESIAN_POINT('',(8.76432075605962,-7.39577200905833,-81.35));
#54581=CARTESIAN_POINT('Origin',(8.21904360754086,-7.32384961127259,-81.35));
#54582=CARTESIAN_POINT('',(10.7007720090583,-5.45932075605962,-81.35));
#54583=CARTESIAN_POINT('Origin',(10.995,-7.69,-81.35));
#54584=CARTESIAN_POINT('',(11.0177583409252,-5.30295233719346,-81.35));
#54585=CARTESIAN_POINT('Origin',(10.6288496112726,-4.91404360754086,-81.35));
#54586=CARTESIAN_POINT('',(11.3889087296526,-4.93180194846606,-81.35));
#54587=CARTESIAN_POINT('',(11.3889087296526,-4.93180194846606,-81.35));
#54588=CARTESIAN_POINT('',(11.55,-4.54289321881346,-81.35));
#54589=CARTESIAN_POINT('Origin',(11.,-4.54289321881346,-81.35));
#54590=CARTESIAN_POINT('',(11.55,-3.65710678118656,-81.35));
#54591=CARTESIAN_POINT('',(11.55,-3.65710678118656,-81.35));
#54592=CARTESIAN_POINT('',(11.3889087296526,-3.26819805153396,-81.35));
#54593=CARTESIAN_POINT('Origin',(11.,-3.65710678118656,-81.35));
#54594=CARTESIAN_POINT('',(11.0177583409252,-2.89704766280654,-81.35));
#54595=CARTESIAN_POINT('',(11.0177583409252,-2.89704766280654,-81.35));
#54596=CARTESIAN_POINT('',(10.7007720090583,-2.74067924394038,-81.35));
#54597=CARTESIAN_POINT('Origin',(10.6288496112726,-3.28595639245914,-81.35));
#54598=CARTESIAN_POINT('',(8.76432075605962,-0.804227990941667,-81.35));
#54599=CARTESIAN_POINT('Origin',(10.995,-0.509999999999999,-81.35));
#54600=CARTESIAN_POINT('',(8.60795233719346,-0.487241659074806,-81.35));
#54601=CARTESIAN_POINT('Origin',(8.21904360754086,-0.876150388727407,-81.35));
#54602=CARTESIAN_POINT('',(8.07071067811865,0.0500000000000006,-81.35));
#54603=CARTESIAN_POINT('',(8.07071067811865,0.0500000000000006,-81.35));
#54604=CARTESIAN_POINT('',(-8.07071067811865,0.0499999999999998,-81.35));
#54605=CARTESIAN_POINT('',(-8.07071067811865,0.0499999999999998,-81.35));
#54606=CARTESIAN_POINT('',(-8.60795233719346,-0.48724165907481,-81.35));
#54607=CARTESIAN_POINT('',(-8.60795233719346,-0.487241659074809,-81.35));
#54608=CARTESIAN_POINT('',(-8.76432075605962,-0.804227990941668,-81.35));
#54609=CARTESIAN_POINT('Origin',(-8.21904360754086,-0.87615038872741,-81.35));
#54610=CARTESIAN_POINT('',(-10.7007720090583,-2.74067924394038,-81.35));
#54611=CARTESIAN_POINT('Origin',(-10.995,-0.510000000000002,-81.35));
#54612=CARTESIAN_POINT('',(-11.0177583409252,-2.89704766280654,-81.35));
#54613=CARTESIAN_POINT('Origin',(-10.6288496112726,-3.28595639245914,-81.35));
#54614=CARTESIAN_POINT('',(-11.3889087296526,-3.26819805153396,-81.35));
#54615=CARTESIAN_POINT('',(-11.3889087296526,-3.26819805153396,-81.35));
#54616=CARTESIAN_POINT('',(-11.55,-3.65710678118656,-81.35));
#54617=CARTESIAN_POINT('Origin',(-11.,-3.65710678118656,-81.35));
#54618=CARTESIAN_POINT('',(-11.55,-4.54289321881346,-81.35));
#54619=CARTESIAN_POINT('',(-11.55,-4.54289321881346,-81.35));
#54620=CARTESIAN_POINT('',(-11.3889087296526,-4.93180194846607,-81.35));
#54621=CARTESIAN_POINT('Origin',(-11.,-4.54289321881346,-81.35));
#54622=CARTESIAN_POINT('',(-11.0177583409252,-5.30295233719346,-81.35));
#54623=CARTESIAN_POINT('',(-11.0177583409252,-5.30295233719346,-81.35));
#54624=CARTESIAN_POINT('',(-10.7007720090583,-5.45932075605962,-81.35));
#54625=CARTESIAN_POINT('Origin',(-10.6288496112726,-4.91404360754086,-81.35));
#54626=CARTESIAN_POINT('',(-8.76432075605962,-7.39577200905833,-81.35));
#54627=CARTESIAN_POINT('Origin',(-10.995,-7.69,-81.35));
#54628=CARTESIAN_POINT('',(-8.60795233719346,-7.7127583409252,-81.35));
#54629=CARTESIAN_POINT('Origin',(-8.21904360754086,-7.32384961127259,-81.35));
#54630=CARTESIAN_POINT('',(-8.23180194846605,-8.0889087296526,-81.35));
#54631=CARTESIAN_POINT('',(-8.23180194846605,-8.0889087296526,-81.35));
#54632=CARTESIAN_POINT('',(-8.1,-8.40710678118654,-81.35));
#54633=CARTESIAN_POINT('Origin',(-8.55,-8.40710678118654,-81.35));
#54634=CARTESIAN_POINT('',(-8.1,-12.0328932188134,-81.35));
#54635=CARTESIAN_POINT('',(-8.1,-12.0328932188134,-81.35));
#54636=CARTESIAN_POINT('',(-8.23180194846605,-12.3510912703474,-81.35));
#54637=CARTESIAN_POINT('Origin',(-8.55,-12.0328932188134,-81.35));
#54638=CARTESIAN_POINT('',(-12.3307106781186,-16.45,-81.35));
#54639=CARTESIAN_POINT('',(-12.3307106781186,-16.45,-81.35));
#54640=CARTESIAN_POINT('',(-22.1792893218814,-16.45,-81.35));
#54641=CARTESIAN_POINT('',(-22.1792893218814,-16.45,-81.35));
#54642=CARTESIAN_POINT('',(-23.15,-15.4792893218813,-81.35));
#54643=CARTESIAN_POINT('',(-23.15,-15.4792893218813,-81.35));
#54644=CARTESIAN_POINT('',(-23.15,11.9792893218814,-81.35));
#54645=CARTESIAN_POINT('',(-23.15,11.9792893218814,-81.35));
#54646=CARTESIAN_POINT('',(-22.1792893218813,12.95,-81.35));
#54647=CARTESIAN_POINT('',(-22.1792893218813,12.95,-81.35));
#54648=CARTESIAN_POINT('',(22.1792893218813,12.95,-81.35));
#54649=CARTESIAN_POINT('',(22.1792893218813,12.95,-81.35));
#54650=CARTESIAN_POINT('',(23.15,11.9792893218814,-81.35));
#54651=CARTESIAN_POINT('',(23.15,11.9792893218814,-81.35));
#54652=CARTESIAN_POINT('',(23.15,-15.4792893218813,-81.35));
#54653=CARTESIAN_POINT('',(23.15,-15.4792893218813,-81.35));
#54654=CARTESIAN_POINT('',(22.1792893218814,-16.45,-81.35));
#54655=CARTESIAN_POINT('',(22.1792893218814,-16.45,-81.35));
#54656=CARTESIAN_POINT('',(12.3307106781187,-16.45,-81.35));
#54657=CARTESIAN_POINT('Origin',(8.23180194846605,-12.3510912703474,-81.35));
#54658=CARTESIAN_POINT('',(8.23180194846605,-12.3510912703474,-81.3));
#54659=CARTESIAN_POINT('',(12.3307106781187,-16.45,-81.3));
#54660=CARTESIAN_POINT('',(8.23180194846605,-12.3510912703474,-81.3));
#54661=CARTESIAN_POINT('',(8.23180194846605,-12.3510912703474,-81.35));
#54662=CARTESIAN_POINT('',(12.3307106781187,-16.45,-81.35));
#54663=CARTESIAN_POINT('Origin',(8.55,-12.0328932188134,-81.35));
#54664=CARTESIAN_POINT('',(8.1,-12.0328932188134,-81.3));
#54665=CARTESIAN_POINT('Origin',(8.55,-12.0328932188134,-81.3));
#54666=CARTESIAN_POINT('',(8.1,-12.0328932188134,-81.35));
#54667=CARTESIAN_POINT('Origin',(8.1,-8.40710678118654,-81.35));
#54668=CARTESIAN_POINT('',(8.1,-8.40710678118654,-81.3));
#54669=CARTESIAN_POINT('',(8.1,-8.40710678118654,-81.3));
#54670=CARTESIAN_POINT('',(8.1,-8.40710678118654,-81.35));
#54671=CARTESIAN_POINT('Origin',(8.55,-8.40710678118654,-81.35));
#54672=CARTESIAN_POINT('',(8.23180194846606,-8.08890872965259,-81.3));
#54673=CARTESIAN_POINT('Origin',(8.55,-8.40710678118654,-81.3));
#54674=CARTESIAN_POINT('',(8.23180194846606,-8.08890872965259,-81.35));
#54675=CARTESIAN_POINT('Origin',(8.60795233719346,-7.71275834092519,-81.35));
#54676=CARTESIAN_POINT('',(8.60795233719346,-7.71275834092519,-81.3));
#54677=CARTESIAN_POINT('',(8.60795233719346,-7.71275834092519,-81.3));
#54678=CARTESIAN_POINT('',(8.60795233719346,-7.71275834092519,-81.35));
#54679=CARTESIAN_POINT('Origin',(8.21904360754086,-7.32384961127259,-81.35));
#54680=CARTESIAN_POINT('',(8.76432075605962,-7.39577200905833,-81.3));
#54681=CARTESIAN_POINT('Origin',(8.21904360754086,-7.32384961127259,-81.3));
#54682=CARTESIAN_POINT('',(8.76432075605962,-7.39577200905833,-81.35));
#54683=CARTESIAN_POINT('Origin',(10.995,-7.69,-81.35));
#54684=CARTESIAN_POINT('',(10.7007720090583,-5.45932075605962,-81.3));
#54685=CARTESIAN_POINT('Origin',(10.995,-7.69,-81.3));
#54686=CARTESIAN_POINT('',(10.7007720090583,-5.45932075605962,-81.35));
#54687=CARTESIAN_POINT('Origin',(10.6288496112726,-4.91404360754086,-81.35));
#54688=CARTESIAN_POINT('',(11.0177583409252,-5.30295233719346,-81.3));
#54689=CARTESIAN_POINT('Origin',(10.6288496112726,-4.91404360754086,-81.3));
#54690=CARTESIAN_POINT('',(11.0177583409252,-5.30295233719346,-81.35));
#54691=CARTESIAN_POINT('Origin',(11.3889087296526,-4.93180194846606,-81.35));
#54692=CARTESIAN_POINT('',(11.3889087296526,-4.93180194846606,-81.3));
#54693=CARTESIAN_POINT('',(11.3889087296526,-4.93180194846606,-81.3));
#54694=CARTESIAN_POINT('',(11.3889087296526,-4.93180194846606,-81.35));
#54695=CARTESIAN_POINT('Origin',(11.,-4.54289321881346,-81.35));
#54696=CARTESIAN_POINT('',(11.55,-4.54289321881346,-81.3));
#54697=CARTESIAN_POINT('Origin',(11.,-4.54289321881346,-81.3));
#54698=CARTESIAN_POINT('',(11.55,-4.54289321881346,-81.35));
#54699=CARTESIAN_POINT('Origin',(11.55,-3.65710678118656,-81.35));
#54700=CARTESIAN_POINT('',(11.55,-3.65710678118656,-81.3));
#54701=CARTESIAN_POINT('',(11.55,-3.65710678118656,-81.3));
#54702=CARTESIAN_POINT('',(11.55,-3.65710678118656,-81.35));
#54703=CARTESIAN_POINT('Origin',(11.,-3.65710678118656,-81.35));
#54704=CARTESIAN_POINT('',(11.3889087296526,-3.26819805153396,-81.3));
#54705=CARTESIAN_POINT('Origin',(11.,-3.65710678118656,-81.3));
#54706=CARTESIAN_POINT('',(11.3889087296526,-3.26819805153396,-81.35));
#54707=CARTESIAN_POINT('Origin',(11.0177583409252,-2.89704766280654,-81.35));
#54708=CARTESIAN_POINT('',(11.0177583409252,-2.89704766280654,-81.3));
#54709=CARTESIAN_POINT('',(11.0177583409252,-2.89704766280654,-81.3));
#54710=CARTESIAN_POINT('',(11.0177583409252,-2.89704766280654,-81.35));
#54711=CARTESIAN_POINT('Origin',(10.6288496112726,-3.28595639245914,-81.35));
#54712=CARTESIAN_POINT('',(10.7007720090583,-2.74067924394038,-81.3));
#54713=CARTESIAN_POINT('Origin',(10.6288496112726,-3.28595639245914,-81.3));
#54714=CARTESIAN_POINT('',(10.7007720090583,-2.74067924394038,-81.35));
#54715=CARTESIAN_POINT('Origin',(10.995,-0.509999999999999,-81.35));
#54716=CARTESIAN_POINT('',(8.76432075605962,-0.804227990941667,-81.3));
#54717=CARTESIAN_POINT('Origin',(10.995,-0.509999999999999,-81.3));
#54718=CARTESIAN_POINT('',(8.76432075605962,-0.804227990941667,-81.35));
#54719=CARTESIAN_POINT('Origin',(8.21904360754086,-0.876150388727407,-81.35));
#54720=CARTESIAN_POINT('',(8.60795233719346,-0.487241659074806,-81.3));
#54721=CARTESIAN_POINT('Origin',(8.21904360754086,-0.876150388727407,-81.3));
#54722=CARTESIAN_POINT('',(8.60795233719346,-0.487241659074806,-81.35));
#54723=CARTESIAN_POINT('Origin',(8.07071067811865,0.0500000000000006,-81.35));
#54724=CARTESIAN_POINT('',(8.07071067811865,0.0500000000000006,-81.3));
#54725=CARTESIAN_POINT('',(8.07071067811865,0.0500000000000006,-81.3));
#54726=CARTESIAN_POINT('',(8.07071067811865,0.0500000000000006,-81.35));
#54727=CARTESIAN_POINT('Origin',(-8.07071067811865,0.0499999999999998,-81.35));
#54728=CARTESIAN_POINT('',(-8.07071067811865,0.0499999999999998,-81.3));
#54729=CARTESIAN_POINT('',(-8.07071067811865,0.0499999999999998,-81.3));
#54730=CARTESIAN_POINT('',(-8.07071067811865,0.0499999999999998,-81.35));
#54731=CARTESIAN_POINT('Origin',(-8.60795233719346,-0.487241659074809,-81.35));
#54732=CARTESIAN_POINT('',(-8.60795233719346,-0.48724165907481,-81.3));
#54733=CARTESIAN_POINT('',(-8.60795233719346,-0.487241659074809,-81.3));
#54734=CARTESIAN_POINT('',(-8.60795233719346,-0.48724165907481,-81.35));
#54735=CARTESIAN_POINT('Origin',(-8.21904360754086,-0.87615038872741,-81.35));
#54736=CARTESIAN_POINT('',(-8.76432075605962,-0.804227990941668,-81.3));
#54737=CARTESIAN_POINT('Origin',(-8.21904360754086,-0.87615038872741,-81.3));
#54738=CARTESIAN_POINT('',(-8.76432075605962,-0.804227990941668,-81.35));
#54739=CARTESIAN_POINT('Origin',(-10.995,-0.510000000000002,-81.35));
#54740=CARTESIAN_POINT('',(-10.7007720090583,-2.74067924394038,-81.3));
#54741=CARTESIAN_POINT('Origin',(-10.995,-0.510000000000002,-81.3));
#54742=CARTESIAN_POINT('',(-10.7007720090583,-2.74067924394038,-81.35));
#54743=CARTESIAN_POINT('Origin',(-10.6288496112726,-3.28595639245914,-81.35));
#54744=CARTESIAN_POINT('',(-11.0177583409252,-2.89704766280654,-81.3));
#54745=CARTESIAN_POINT('Origin',(-10.6288496112726,-3.28595639245914,-81.3));
#54746=CARTESIAN_POINT('',(-11.0177583409252,-2.89704766280654,-81.35));
#54747=CARTESIAN_POINT('Origin',(-11.3889087296526,-3.26819805153396,-81.35));
#54748=CARTESIAN_POINT('',(-11.3889087296526,-3.26819805153396,-81.3));
#54749=CARTESIAN_POINT('',(-11.3889087296526,-3.26819805153396,-81.3));
#54750=CARTESIAN_POINT('',(-11.3889087296526,-3.26819805153396,-81.35));
#54751=CARTESIAN_POINT('Origin',(-11.,-3.65710678118656,-81.35));
#54752=CARTESIAN_POINT('',(-11.55,-3.65710678118656,-81.3));
#54753=CARTESIAN_POINT('Origin',(-11.,-3.65710678118656,-81.3));
#54754=CARTESIAN_POINT('',(-11.55,-3.65710678118656,-81.35));
#54755=CARTESIAN_POINT('Origin',(-11.55,-4.54289321881346,-81.35));
#54756=CARTESIAN_POINT('',(-11.55,-4.54289321881346,-81.3));
#54757=CARTESIAN_POINT('',(-11.55,-4.54289321881346,-81.3));
#54758=CARTESIAN_POINT('',(-11.55,-4.54289321881346,-81.35));
#54759=CARTESIAN_POINT('Origin',(-11.,-4.54289321881346,-81.35));
#54760=CARTESIAN_POINT('',(-11.3889087296526,-4.93180194846607,-81.3));
#54761=CARTESIAN_POINT('Origin',(-11.,-4.54289321881346,-81.3));
#54762=CARTESIAN_POINT('',(-11.3889087296526,-4.93180194846607,-81.35));
#54763=CARTESIAN_POINT('Origin',(-11.0177583409252,-5.30295233719346,-81.35));
#54764=CARTESIAN_POINT('',(-11.0177583409252,-5.30295233719346,-81.3));
#54765=CARTESIAN_POINT('',(-11.0177583409252,-5.30295233719346,-81.3));
#54766=CARTESIAN_POINT('',(-11.0177583409252,-5.30295233719346,-81.35));
#54767=CARTESIAN_POINT('Origin',(-10.6288496112726,-4.91404360754086,-81.35));
#54768=CARTESIAN_POINT('',(-10.7007720090583,-5.45932075605962,-81.3));
#54769=CARTESIAN_POINT('Origin',(-10.6288496112726,-4.91404360754086,-81.3));
#54770=CARTESIAN_POINT('',(-10.7007720090583,-5.45932075605962,-81.35));
#54771=CARTESIAN_POINT('Origin',(-10.995,-7.69,-81.35));
#54772=CARTESIAN_POINT('',(-8.76432075605962,-7.39577200905833,-81.3));
#54773=CARTESIAN_POINT('Origin',(-10.995,-7.69,-81.3));
#54774=CARTESIAN_POINT('',(-8.76432075605962,-7.39577200905833,-81.35));
#54775=CARTESIAN_POINT('Origin',(-8.21904360754086,-7.32384961127259,-81.35));
#54776=CARTESIAN_POINT('',(-8.60795233719346,-7.7127583409252,-81.3));
#54777=CARTESIAN_POINT('Origin',(-8.21904360754086,-7.32384961127259,-81.3));
#54778=CARTESIAN_POINT('',(-8.60795233719346,-7.7127583409252,-81.35));
#54779=CARTESIAN_POINT('Origin',(-8.23180194846605,-8.0889087296526,-81.35));
#54780=CARTESIAN_POINT('',(-8.23180194846605,-8.0889087296526,-81.3));
#54781=CARTESIAN_POINT('',(-8.23180194846605,-8.0889087296526,-81.3));
#54782=CARTESIAN_POINT('',(-8.23180194846605,-8.0889087296526,-81.35));
#54783=CARTESIAN_POINT('Origin',(-8.55,-8.40710678118654,-81.35));
#54784=CARTESIAN_POINT('',(-8.1,-8.40710678118654,-81.3));
#54785=CARTESIAN_POINT('Origin',(-8.55,-8.40710678118654,-81.3));
#54786=CARTESIAN_POINT('',(-8.1,-8.40710678118654,-81.35));
#54787=CARTESIAN_POINT('Origin',(-8.1,-12.0328932188134,-81.35));
#54788=CARTESIAN_POINT('',(-8.1,-12.0328932188134,-81.3));
#54789=CARTESIAN_POINT('',(-8.1,-12.0328932188134,-81.3));
#54790=CARTESIAN_POINT('',(-8.1,-12.0328932188134,-81.35));
#54791=CARTESIAN_POINT('Origin',(-8.55,-12.0328932188134,-81.35));
#54792=CARTESIAN_POINT('',(-8.23180194846605,-12.3510912703474,-81.3));
#54793=CARTESIAN_POINT('Origin',(-8.55,-12.0328932188134,-81.3));
#54794=CARTESIAN_POINT('',(-8.23180194846605,-12.3510912703474,-81.35));
#54795=CARTESIAN_POINT('Origin',(-12.3307106781186,-16.45,-81.35));
#54796=CARTESIAN_POINT('',(-12.3307106781186,-16.45,-81.3));
#54797=CARTESIAN_POINT('',(-12.3307106781186,-16.45,-81.3));
#54798=CARTESIAN_POINT('',(-12.3307106781186,-16.45,-81.35));
#54799=CARTESIAN_POINT('Origin',(-22.1792893218814,-16.45,-81.35));
#54800=CARTESIAN_POINT('',(-22.1792893218814,-16.45,-81.3));
#54801=CARTESIAN_POINT('',(-22.1792893218814,-16.45,-81.3));
#54802=CARTESIAN_POINT('',(-22.1792893218814,-16.45,-81.35));
#54803=CARTESIAN_POINT('Origin',(-23.15,-15.4792893218813,-81.35));
#54804=CARTESIAN_POINT('',(-23.15,-15.4792893218813,-81.3));
#54805=CARTESIAN_POINT('',(-23.15,-15.4792893218813,-81.3));
#54806=CARTESIAN_POINT('',(-23.15,-15.4792893218813,-81.35));
#54807=CARTESIAN_POINT('Origin',(-23.15,11.9792893218814,-81.35));
#54808=CARTESIAN_POINT('',(-23.15,11.9792893218814,-81.3));
#54809=CARTESIAN_POINT('',(-23.15,11.9792893218814,-81.3));
#54810=CARTESIAN_POINT('',(-23.15,11.9792893218814,-81.35));
#54811=CARTESIAN_POINT('Origin',(-22.1792893218813,12.95,-81.35));
#54812=CARTESIAN_POINT('',(-22.1792893218813,12.95,-81.3));
#54813=CARTESIAN_POINT('',(-22.1792893218813,12.95,-81.3));
#54814=CARTESIAN_POINT('',(-22.1792893218813,12.95,-81.35));
#54815=CARTESIAN_POINT('Origin',(22.1792893218813,12.95,-81.35));
#54816=CARTESIAN_POINT('',(22.1792893218813,12.95,-81.3));
#54817=CARTESIAN_POINT('',(22.1792893218813,12.95,-81.3));
#54818=CARTESIAN_POINT('',(22.1792893218813,12.95,-81.35));
#54819=CARTESIAN_POINT('Origin',(23.15,11.9792893218814,-81.35));
#54820=CARTESIAN_POINT('',(23.15,11.9792893218814,-81.3));
#54821=CARTESIAN_POINT('',(23.15,11.9792893218814,-81.3));
#54822=CARTESIAN_POINT('',(23.15,11.9792893218814,-81.35));
#54823=CARTESIAN_POINT('Origin',(23.15,-15.4792893218813,-81.35));
#54824=CARTESIAN_POINT('',(23.15,-15.4792893218813,-81.3));
#54825=CARTESIAN_POINT('',(23.15,-15.4792893218813,-81.3));
#54826=CARTESIAN_POINT('',(23.15,-15.4792893218813,-81.35));
#54827=CARTESIAN_POINT('Origin',(22.1792893218814,-16.45,-81.35));
#54828=CARTESIAN_POINT('',(22.1792893218814,-16.45,-81.3));
#54829=CARTESIAN_POINT('',(22.1792893218814,-16.45,-81.3));
#54830=CARTESIAN_POINT('',(22.1792893218814,-16.45,-81.35));
#54831=CARTESIAN_POINT('Origin',(12.3307106781187,-16.45,-81.35));
#54832=CARTESIAN_POINT('',(12.3307106781187,-16.45,-81.3));
#54833=CARTESIAN_POINT('Origin',(-1.62630325872826E-14,12.5,-10.6));
#54834=CARTESIAN_POINT('Origin',(-1.50786351795467E-14,12.7,-8.1));
#54835=CARTESIAN_POINT('',(-0.500000000000016,12.7,-8.1));
#54836=CARTESIAN_POINT('',(-0.500000000000016,12.7,-8.1));
#54837=CARTESIAN_POINT('',(0.499999999999983,12.7,-8.1));
#54838=CARTESIAN_POINT('Origin',(-1.50786351795467E-14,12.7,-8.1));
#54839=CARTESIAN_POINT('',(0.499999999999983,12.7,-8.1));
#54840=CARTESIAN_POINT('Origin',(0.,0.,0.));
#54841=CARTESIAN_POINT('',(4.99995,13.,0.));
#54842=CARTESIAN_POINT('',(22.2,13.,0.));
#54843=CARTESIAN_POINT('',(-22.2,13.,0.));
#54844=CARTESIAN_POINT('',(4.99995,8.,0.));
#54845=CARTESIAN_POINT('',(4.99995,13.,0.));
#54846=CARTESIAN_POINT('',(-4.99995,8.,0.));
#54847=CARTESIAN_POINT('Origin',(0.,8.,0.));
#54848=CARTESIAN_POINT('',(-4.99995,13.,0.));
#54849=CARTESIAN_POINT('',(-4.99995,13.,0.));
#54850=CARTESIAN_POINT('',(-22.2,13.,0.));
#54851=CARTESIAN_POINT('',(-22.2,13.,0.));
#54852=CARTESIAN_POINT('',(-23.2,12.,0.));
#54853=CARTESIAN_POINT('',(-22.2,13.,0.));
#54854=CARTESIAN_POINT('',(-23.2,-15.5,0.));
#54855=CARTESIAN_POINT('',(-23.2,12.,0.));
#54856=CARTESIAN_POINT('',(-22.2,-16.5,0.));
#54857=CARTESIAN_POINT('',(-23.2,-15.5,0.));
#54858=CARTESIAN_POINT('',(-12.31,-16.5,0.));
#54859=CARTESIAN_POINT('',(-23.,-16.5,0.));
#54860=CARTESIAN_POINT('',(-8.19644660940672,-12.3864466094067,0.));
#54861=CARTESIAN_POINT('',(-12.31,-16.5,0.));
#54862=CARTESIAN_POINT('',(-8.05,-12.0328932188134,0.));
#54863=CARTESIAN_POINT('Origin',(-8.55,-12.0328932188134,0.));
#54864=CARTESIAN_POINT('',(-8.05,-8.40710678118654,0.));
#54865=CARTESIAN_POINT('',(-8.05,-12.24,0.));
#54866=CARTESIAN_POINT('',(-8.19644660940673,-8.05355339059327,0.));
#54867=CARTESIAN_POINT('Origin',(-8.55,-8.40710678118654,0.));
#54868=CARTESIAN_POINT('',(-8.57259699813413,-7.67740300186587,0.));
#54869=CARTESIAN_POINT('',(-8.05,-8.2,0.));
#54870=CARTESIAN_POINT('',(-8.71475010619428,-7.38923360925963,0.));
#54871=CARTESIAN_POINT('Origin',(-8.21904360754086,-7.32384961127259,0.));
#54872=CARTESIAN_POINT('',(-10.6942336092596,-5.40975010619428,0.));
#54873=CARTESIAN_POINT('Origin',(-10.995,-7.69,0.));
#54874=CARTESIAN_POINT('',(-10.9824030018659,-5.26759699813413,0.));
#54875=CARTESIAN_POINT('Origin',(-10.6288496112726,-4.91404360754086,0.));
#54876=CARTESIAN_POINT('',(-11.3535533905933,-4.89644660940674,0.));
#54877=CARTESIAN_POINT('',(-8.05,-8.2,0.));
#54878=CARTESIAN_POINT('',(-11.5,-4.54289321881346,0.));
#54879=CARTESIAN_POINT('Origin',(-11.,-4.54289321881346,0.));
#54880=CARTESIAN_POINT('',(-11.5,-3.65710678118656,0.));
#54881=CARTESIAN_POINT('',(-11.5,-4.75000000000001,0.));
#54882=CARTESIAN_POINT('',(-11.3535533905933,-3.30355339059329,0.));
#54883=CARTESIAN_POINT('Origin',(-11.,-3.65710678118656,0.));
#54884=CARTESIAN_POINT('',(-10.9824030018659,-2.93240300186587,0.));
#54885=CARTESIAN_POINT('',(-8.05,-1.60428730688303E-15,0.));
#54886=CARTESIAN_POINT('',(-10.6942336092596,-2.79024989380572,0.));
#54887=CARTESIAN_POINT('Origin',(-10.6288496112726,-3.28595639245914,0.));
#54888=CARTESIAN_POINT('',(-8.71475010619428,-0.810766390740372,0.));
#54889=CARTESIAN_POINT('Origin',(-10.995,-0.510000000000002,0.));
#54890=CARTESIAN_POINT('',(-8.57259699813413,-0.522596998134137,0.));
#54891=CARTESIAN_POINT('Origin',(-8.21904360754086,-0.87615038872741,0.));
#54892=CARTESIAN_POINT('',(-8.05,-1.60428730688303E-15,0.));
#54893=CARTESIAN_POINT('',(-8.05,-1.60428730688303E-15,0.));
#54894=CARTESIAN_POINT('',(8.05,3.67394039744206E-16,0.));
#54895=CARTESIAN_POINT('',(8.05,3.67394039744206E-16,0.));
#54896=CARTESIAN_POINT('',(8.57259699813413,-0.522596998134133,0.));
#54897=CARTESIAN_POINT('',(8.05,3.67394039744206E-16,0.));
#54898=CARTESIAN_POINT('',(8.71475010619428,-0.81076639074037,0.));
#54899=CARTESIAN_POINT('Origin',(8.21904360754086,-0.876150388727407,0.));
#54900=CARTESIAN_POINT('',(10.6942336092596,-2.79024989380572,0.));
#54901=CARTESIAN_POINT('Origin',(10.995,-0.509999999999999,0.));
#54902=CARTESIAN_POINT('',(10.9824030018659,-2.93240300186586,0.));
#54903=CARTESIAN_POINT('Origin',(10.6288496112726,-3.28595639245914,0.));
#54904=CARTESIAN_POINT('',(11.3535533905933,-3.30355339059329,0.));
#54905=CARTESIAN_POINT('',(8.05,3.67394039744206E-16,0.));
#54906=CARTESIAN_POINT('',(11.5,-3.65710678118656,0.));
#54907=CARTESIAN_POINT('Origin',(11.,-3.65710678118656,0.));
#54908=CARTESIAN_POINT('',(11.5,-4.54289321881346,0.));
#54909=CARTESIAN_POINT('',(11.5,-4.75000000000001,0.));
#54910=CARTESIAN_POINT('',(11.3535533905933,-4.89644660940673,0.));
#54911=CARTESIAN_POINT('Origin',(11.,-4.54289321881346,0.));
#54912=CARTESIAN_POINT('',(10.9824030018659,-5.26759699813413,0.));
#54913=CARTESIAN_POINT('',(8.05,-8.2,0.));
#54914=CARTESIAN_POINT('',(10.6942336092596,-5.40975010619428,0.));
#54915=CARTESIAN_POINT('Origin',(10.6288496112726,-4.91404360754086,0.));
#54916=CARTESIAN_POINT('',(8.71475010619428,-7.38923360925963,0.));
#54917=CARTESIAN_POINT('Origin',(10.995,-7.69,0.));
#54918=CARTESIAN_POINT('',(8.57259699813413,-7.67740300186587,0.));
#54919=CARTESIAN_POINT('Origin',(8.21904360754086,-7.32384961127259,0.));
#54920=CARTESIAN_POINT('',(8.19644660940673,-8.05355339059327,0.));
#54921=CARTESIAN_POINT('',(8.05,-8.2,0.));
#54922=CARTESIAN_POINT('',(8.05,-8.40710678118654,0.));
#54923=CARTESIAN_POINT('Origin',(8.55,-8.40710678118654,0.));
#54924=CARTESIAN_POINT('',(8.05,-12.0328932188134,0.));
#54925=CARTESIAN_POINT('',(8.05,-12.24,0.));
#54926=CARTESIAN_POINT('',(8.19644660940673,-12.3864466094067,0.));
#54927=CARTESIAN_POINT('Origin',(8.55,-12.0328932188134,0.));
#54928=CARTESIAN_POINT('',(12.31,-16.5,0.));
#54929=CARTESIAN_POINT('',(12.31,-16.5,0.));
#54930=CARTESIAN_POINT('',(22.2,-16.5,0.));
#54931=CARTESIAN_POINT('',(12.31,-16.5,0.));
#54932=CARTESIAN_POINT('',(23.2,-15.5,0.));
#54933=CARTESIAN_POINT('',(23.2,-15.5,0.));
#54934=CARTESIAN_POINT('',(23.2,12.,0.));
#54935=CARTESIAN_POINT('',(23.2,12.,0.));
#54936=CARTESIAN_POINT('',(22.2,13.,0.));
#54937=CARTESIAN_POINT('Origin',(0.499999999999983,12.7,-8.1));
#54938=CARTESIAN_POINT('',(0.499999999999983,13.,-8.1));
#54939=CARTESIAN_POINT('',(0.499999999999983,13.,-8.1));
#54940=CARTESIAN_POINT('',(0.499999999999983,12.7,-8.1));
#54941=CARTESIAN_POINT('Origin',(-0.500000000000016,12.7,-8.1));
#54942=CARTESIAN_POINT('',(-0.500000000000017,13.,-8.1));
#54943=CARTESIAN_POINT('',(-0.500000000000017,13.,-8.1));
#54944=CARTESIAN_POINT('',(-0.500000000000016,12.7,-8.1));
#54945=CARTESIAN_POINT('Origin',(-1.50786351795467E-14,12.7,-8.1));
#54946=CARTESIAN_POINT('Origin',(-1.54689479616415E-14,13.,-8.1));
#54947=CARTESIAN_POINT('Origin',(-1.87674352915389E-14,12.5,-74.2));
#54948=CARTESIAN_POINT('Origin',(-1.50786351795467E-14,12.7,-76.7));
#54949=CARTESIAN_POINT('',(0.499999999999986,12.7,-76.7));
#54950=CARTESIAN_POINT('',(0.499999999999986,12.7,-76.7));
#54951=CARTESIAN_POINT('',(-0.500000000000025,12.7,-76.7));
#54952=CARTESIAN_POINT('Origin',(-1.50786351795467E-14,12.7,-76.7));
#54953=CARTESIAN_POINT('',(-0.500000000000025,12.7,-76.7));
#54954=CARTESIAN_POINT('Origin',(12.31,-16.5,-84.8));
#54955=CARTESIAN_POINT('',(12.31,-16.5,-3.45));
#54956=CARTESIAN_POINT('',(22.2,-16.5,-3.45));
#54957=CARTESIAN_POINT('',(12.31,-16.5,-3.45));
#54958=CARTESIAN_POINT('',(22.2,-16.5,-13.4));
#54959=CARTESIAN_POINT('',(12.31,-16.5,-84.8));
#54960=CARTESIAN_POINT('Origin',(23.2,-15.5,-13.4));
#54961=CARTESIAN_POINT('',(23.2,-15.5,-3.45));
#54962=CARTESIAN_POINT('',(22.2,-16.5,-3.45));
#54963=CARTESIAN_POINT('',(23.2,-15.5,-13.4));
#54964=CARTESIAN_POINT('Origin',(23.2,12.,-13.4));
#54965=CARTESIAN_POINT('',(23.2,12.,-3.45));
#54966=CARTESIAN_POINT('',(23.2,-15.5,-3.45));
#54967=CARTESIAN_POINT('',(23.2,12.,-13.4));
#54968=CARTESIAN_POINT('Origin',(22.2,13.,-13.4));
#54969=CARTESIAN_POINT('',(22.2,13.,-3.45));
#54970=CARTESIAN_POINT('',(23.2,12.,-3.45));
#54971=CARTESIAN_POINT('',(22.2,13.,-13.4));
#54972=CARTESIAN_POINT('Origin',(-22.2,13.,-13.4));
#54973=CARTESIAN_POINT('',(4.99995,13.,-0.999999999999999));
#54974=CARTESIAN_POINT('',(-4.99995,13.,-1.));
#54975=CARTESIAN_POINT('',(-4.99995,13.,-1.));
#54976=CARTESIAN_POINT('',(4.99995,13.,-1.));
#54977=CARTESIAN_POINT('',(-22.2,13.,-3.45));
#54978=CARTESIAN_POINT('',(22.2,13.,-3.45));
#54979=CARTESIAN_POINT('',(-22.2,13.,-13.4));
#54980=CARTESIAN_POINT('',(-4.99995,13.,-1.));
#54981=CARTESIAN_POINT('Origin',(-22.2,13.,-13.4));
#54982=CARTESIAN_POINT('',(-23.2,12.,-3.45));
#54983=CARTESIAN_POINT('',(-22.2,13.,-3.45));
#54984=CARTESIAN_POINT('',(-23.2,12.,-13.4));
#54985=CARTESIAN_POINT('Origin',(-23.2,12.,-13.4));
#54986=CARTESIAN_POINT('',(-23.2,-15.5,-3.45));
#54987=CARTESIAN_POINT('',(-23.2,12.,-3.45));
#54988=CARTESIAN_POINT('',(-23.2,-15.5,-13.4));
#54989=CARTESIAN_POINT('Origin',(-23.2,-15.5,-13.4));
#54990=CARTESIAN_POINT('',(-22.2,-16.5,-3.45));
#54991=CARTESIAN_POINT('',(-23.2,-15.5,-3.45));
#54992=CARTESIAN_POINT('',(-22.2,-16.5,-13.4));
#54993=CARTESIAN_POINT('Origin',(-23.,-16.5,-84.8));
#54994=CARTESIAN_POINT('',(-12.31,-16.5,-3.45));
#54995=CARTESIAN_POINT('',(-22.2,-16.5,-3.45));
#54996=CARTESIAN_POINT('',(-12.31,-16.5,-84.8));
#54997=CARTESIAN_POINT('Origin',(-12.31,-16.5,-84.8));
#54998=CARTESIAN_POINT('',(-8.19644660940672,-12.3864466094067,-3.45));
#54999=CARTESIAN_POINT('',(-12.31,-16.5,-3.45));
#55000=CARTESIAN_POINT('',(-8.19644660940672,-12.3864466094067,-84.8));
#55001=CARTESIAN_POINT('Origin',(-8.55,-12.0328932188134,-84.8));
#55002=CARTESIAN_POINT('',(-8.05,-12.0328932188134,-3.45));
#55003=CARTESIAN_POINT('Origin',(-8.55,-12.0328932188134,-3.45));
#55004=CARTESIAN_POINT('',(-8.05,-12.0328932188134,-84.8));
#55005=CARTESIAN_POINT('Origin',(-8.05,-12.24,-84.8));
#55006=CARTESIAN_POINT('',(-8.05,-8.40710678118654,-3.45));
#55007=CARTESIAN_POINT('',(-8.05,-12.0328932188134,-3.45));
#55008=CARTESIAN_POINT('',(-8.05,-8.40710678118654,-84.8));
#55009=CARTESIAN_POINT('Origin',(-8.55,-8.40710678118654,-84.8));
#55010=CARTESIAN_POINT('',(-8.19644660940673,-8.05355339059327,-3.45));
#55011=CARTESIAN_POINT('Origin',(-8.55,-8.40710678118654,-3.45));
#55012=CARTESIAN_POINT('',(-8.19644660940673,-8.05355339059327,-84.8));
#55013=CARTESIAN_POINT('Origin',(-8.05,-8.2,-84.8));
#55014=CARTESIAN_POINT('',(-8.57259699813413,-7.67740300186587,-3.45));
#55015=CARTESIAN_POINT('',(-8.19644660940673,-8.05355339059327,-3.45));
#55016=CARTESIAN_POINT('',(-8.57259699813413,-7.67740300186587,0.));
#55017=CARTESIAN_POINT('Origin',(-8.21904360754086,-7.32384961127259,-84.8));
#55018=CARTESIAN_POINT('',(-8.71475010619428,-7.38923360925963,-3.45));
#55019=CARTESIAN_POINT('Origin',(-8.21904360754086,-7.32384961127259,-3.45));
#55020=CARTESIAN_POINT('',(-8.71475010619428,-7.38923360925963,-84.8));
#55021=CARTESIAN_POINT('Origin',(-10.995,-7.69,-84.8));
#55022=CARTESIAN_POINT('',(-10.6942336092596,-5.40975010619428,-3.45));
#55023=CARTESIAN_POINT('Origin',(-10.995,-7.69,-3.45));
#55024=CARTESIAN_POINT('',(-10.6942336092596,-5.40975010619428,-84.8));
#55025=CARTESIAN_POINT('Origin',(-10.6288496112726,-4.91404360754086,-84.8));
#55026=CARTESIAN_POINT('',(-10.9824030018659,-5.26759699813413,-3.45));
#55027=CARTESIAN_POINT('Origin',(-10.6288496112726,-4.91404360754086,-3.45));
#55028=CARTESIAN_POINT('',(-10.9824030018659,-5.26759699813413,-84.8));
#55029=CARTESIAN_POINT('Origin',(-8.05,-8.2,-84.8));
#55030=CARTESIAN_POINT('',(-11.3535533905933,-4.89644660940674,-3.45));
#55031=CARTESIAN_POINT('',(-10.9824030018659,-5.26759699813413,-3.45));
#55032=CARTESIAN_POINT('',(-11.3535533905933,-4.89644660940674,0.));
#55033=CARTESIAN_POINT('Origin',(-11.,-4.54289321881346,-84.8));
#55034=CARTESIAN_POINT('',(-11.5,-4.54289321881346,-3.45));
#55035=CARTESIAN_POINT('Origin',(-11.,-4.54289321881346,-3.45));
#55036=CARTESIAN_POINT('',(-11.5,-4.54289321881346,-84.8));
#55037=CARTESIAN_POINT('Origin',(-11.5,-4.75000000000001,-84.8));
#55038=CARTESIAN_POINT('',(-11.5,-3.65710678118656,-3.45));
#55039=CARTESIAN_POINT('',(-11.5,-4.54289321881346,-3.45));
#55040=CARTESIAN_POINT('',(-11.5,-3.65710678118656,0.));
#55041=CARTESIAN_POINT('Origin',(-11.,-3.65710678118656,-84.8));
#55042=CARTESIAN_POINT('',(-11.3535533905933,-3.30355339059329,-3.45));
#55043=CARTESIAN_POINT('Origin',(-11.,-3.65710678118656,-3.45));
#55044=CARTESIAN_POINT('',(-11.3535533905933,-3.30355339059329,-84.8));
#55045=CARTESIAN_POINT('Origin',(-8.05,-1.60428730688303E-15,-84.8));
#55046=CARTESIAN_POINT('',(-10.9824030018659,-2.93240300186587,-3.45));
#55047=CARTESIAN_POINT('',(-11.3535533905933,-3.30355339059329,-3.45));
#55048=CARTESIAN_POINT('',(-10.9824030018659,-2.93240300186587,0.));
#55049=CARTESIAN_POINT('Origin',(-10.6288496112726,-3.28595639245914,-84.8));
#55050=CARTESIAN_POINT('',(-10.6942336092596,-2.79024989380572,-3.45));
#55051=CARTESIAN_POINT('Origin',(-10.6288496112726,-3.28595639245914,-3.45));
#55052=CARTESIAN_POINT('',(-10.6942336092596,-2.79024989380572,-84.8));
#55053=CARTESIAN_POINT('Origin',(-10.995,-0.510000000000002,-84.8));
#55054=CARTESIAN_POINT('',(-8.71475010619428,-0.810766390740372,-3.45));
#55055=CARTESIAN_POINT('Origin',(-10.995,-0.510000000000002,-3.45));
#55056=CARTESIAN_POINT('',(-8.71475010619428,-0.810766390740372,-84.8));
#55057=CARTESIAN_POINT('Origin',(-8.21904360754086,-0.87615038872741,-84.8));
#55058=CARTESIAN_POINT('',(-8.57259699813413,-0.522596998134137,-3.45));
#55059=CARTESIAN_POINT('Origin',(-8.21904360754086,-0.87615038872741,-3.45));
#55060=CARTESIAN_POINT('',(-8.57259699813413,-0.522596998134137,-84.8));
#55061=CARTESIAN_POINT('Origin',(-8.05,-1.60428730688303E-15,-84.8));
#55062=CARTESIAN_POINT('',(-8.05,-1.60428730688303E-15,-3.45));
#55063=CARTESIAN_POINT('',(-8.57259699813413,-0.522596998134137,-3.45));
#55064=CARTESIAN_POINT('',(-8.05,-1.60428730688303E-15,-84.8));
#55065=CARTESIAN_POINT('Origin',(8.05,3.67394039744206E-16,-84.8));
#55066=CARTESIAN_POINT('',(8.05,3.67394039744206E-16,-3.45));
#55067=CARTESIAN_POINT('',(-8.05,-1.60428730688303E-15,-3.45));
#55068=CARTESIAN_POINT('',(8.05,3.67394039744206E-16,-84.8));
#55069=CARTESIAN_POINT('Origin',(8.05,3.67394039744206E-16,-84.8));
#55070=CARTESIAN_POINT('',(8.57259699813413,-0.522596998134133,-3.45));
#55071=CARTESIAN_POINT('',(8.05,3.67394039744206E-16,-3.45));
#55072=CARTESIAN_POINT('',(8.57259699813413,-0.522596998134133,0.));
#55073=CARTESIAN_POINT('Origin',(8.21904360754086,-0.876150388727407,-84.8));
#55074=CARTESIAN_POINT('',(8.71475010619428,-0.81076639074037,-3.45));
#55075=CARTESIAN_POINT('Origin',(8.21904360754086,-0.876150388727407,-3.45));
#55076=CARTESIAN_POINT('',(8.71475010619428,-0.81076639074037,-84.8));
#55077=CARTESIAN_POINT('Origin',(10.995,-0.509999999999999,-84.8));
#55078=CARTESIAN_POINT('',(10.6942336092596,-2.79024989380572,-3.45));
#55079=CARTESIAN_POINT('Origin',(10.995,-0.509999999999999,-3.45));
#55080=CARTESIAN_POINT('',(10.6942336092596,-2.79024989380572,-84.8));
#55081=CARTESIAN_POINT('Origin',(10.6288496112726,-3.28595639245914,-84.8));
#55082=CARTESIAN_POINT('',(10.9824030018659,-2.93240300186586,-3.45));
#55083=CARTESIAN_POINT('Origin',(10.6288496112726,-3.28595639245914,-3.45));
#55084=CARTESIAN_POINT('',(10.9824030018659,-2.93240300186586,-84.8));
#55085=CARTESIAN_POINT('Origin',(8.05,3.67394039744206E-16,-84.8));
#55086=CARTESIAN_POINT('',(11.3535533905933,-3.30355339059329,-3.45));
#55087=CARTESIAN_POINT('',(10.9824030018659,-2.93240300186586,-3.45));
#55088=CARTESIAN_POINT('',(11.3535533905933,-3.30355339059329,0.));
#55089=CARTESIAN_POINT('Origin',(11.,-3.65710678118656,-84.8));
#55090=CARTESIAN_POINT('',(11.5,-3.65710678118656,-3.45));
#55091=CARTESIAN_POINT('Origin',(11.,-3.65710678118656,-3.45));
#55092=CARTESIAN_POINT('',(11.5,-3.65710678118656,-84.8));
#55093=CARTESIAN_POINT('Origin',(11.5,-4.75000000000001,-84.8));
#55094=CARTESIAN_POINT('',(11.5,-4.54289321881346,-3.45));
#55095=CARTESIAN_POINT('',(11.5,-3.65710678118656,-3.45));
#55096=CARTESIAN_POINT('',(11.5,-4.54289321881346,0.));
#55097=CARTESIAN_POINT('Origin',(11.,-4.54289321881346,-84.8));
#55098=CARTESIAN_POINT('',(11.3535533905933,-4.89644660940673,-3.45));
#55099=CARTESIAN_POINT('Origin',(11.,-4.54289321881346,-3.45));
#55100=CARTESIAN_POINT('',(11.3535533905933,-4.89644660940673,-84.8));
#55101=CARTESIAN_POINT('Origin',(8.05,-8.2,-84.8));
#55102=CARTESIAN_POINT('',(10.9824030018659,-5.26759699813413,-3.45));
#55103=CARTESIAN_POINT('',(11.3535533905933,-4.89644660940673,-3.45));
#55104=CARTESIAN_POINT('',(10.9824030018659,-5.26759699813413,0.));
#55105=CARTESIAN_POINT('Origin',(10.6288496112726,-4.91404360754086,-84.8));
#55106=CARTESIAN_POINT('',(10.6942336092596,-5.40975010619428,-3.45));
#55107=CARTESIAN_POINT('Origin',(10.6288496112726,-4.91404360754086,-3.45));
#55108=CARTESIAN_POINT('',(10.6942336092596,-5.40975010619428,-84.8));
#55109=CARTESIAN_POINT('Origin',(10.995,-7.69,-84.8));
#55110=CARTESIAN_POINT('',(8.71475010619428,-7.38923360925963,-3.45));
#55111=CARTESIAN_POINT('Origin',(10.995,-7.69,-3.45));
#55112=CARTESIAN_POINT('',(8.71475010619428,-7.38923360925963,-84.8));
#55113=CARTESIAN_POINT('Origin',(8.21904360754086,-7.32384961127259,-84.8));
#55114=CARTESIAN_POINT('',(8.57259699813413,-7.67740300186587,-3.45));
#55115=CARTESIAN_POINT('Origin',(8.21904360754086,-7.32384961127259,-3.45));
#55116=CARTESIAN_POINT('',(8.57259699813413,-7.67740300186587,-84.8));
#55117=CARTESIAN_POINT('Origin',(8.05,-8.2,-84.8));
#55118=CARTESIAN_POINT('',(8.19644660940673,-8.05355339059327,-3.45));
#55119=CARTESIAN_POINT('',(8.57259699813413,-7.67740300186587,-3.45));
#55120=CARTESIAN_POINT('',(8.19644660940673,-8.05355339059327,-84.8));
#55121=CARTESIAN_POINT('Origin',(8.55,-8.40710678118654,-84.8));
#55122=CARTESIAN_POINT('',(8.05,-8.40710678118654,-3.45));
#55123=CARTESIAN_POINT('Origin',(8.55,-8.40710678118654,-3.45));
#55124=CARTESIAN_POINT('',(8.05,-8.40710678118654,-84.8));
#55125=CARTESIAN_POINT('Origin',(8.05,-12.24,-84.8));
#55126=CARTESIAN_POINT('',(8.05,-12.0328932188134,-3.45));
#55127=CARTESIAN_POINT('',(8.05,-8.40710678118654,-3.45));
#55128=CARTESIAN_POINT('',(8.05,-12.0328932188134,-84.8));
#55129=CARTESIAN_POINT('Origin',(8.55,-12.0328932188134,-84.8));
#55130=CARTESIAN_POINT('',(8.19644660940673,-12.3864466094067,-3.45));
#55131=CARTESIAN_POINT('Origin',(8.55,-12.0328932188134,-3.45));
#55132=CARTESIAN_POINT('',(8.19644660940673,-12.3864466094067,-84.8));
#55133=CARTESIAN_POINT('Origin',(12.31,-16.5,-84.8));
#55134=CARTESIAN_POINT('',(8.19644660940673,-12.3864466094067,-3.45));
#55135=CARTESIAN_POINT('Origin',(-1.54689479616415E-14,13.,-8.1));
#55136=CARTESIAN_POINT('Origin',(-34.5,4.40457132572236E-15,-104.175753233145));
#55137=CARTESIAN_POINT('',(-30.9292009086072,4.33680868994202E-15,-59.4));
#55138=CARTESIAN_POINT('',(-30.9292009086072,4.33680868994202E-15,-25.4));
#55139=CARTESIAN_POINT('',(-30.9292009086072,4.37613505316247E-15,-13.4));
#55140=CARTESIAN_POINT('',(-34.,4.4005895457577E-15,-25.4));
#55141=CARTESIAN_POINT('',(-34.5,4.40457132572236E-15,-25.4));
#55142=CARTESIAN_POINT('',(-34.,4.4005895457577E-15,-59.4));
#55143=CARTESIAN_POINT('',(-34.,4.4005895457577E-15,-104.175753233145));
#55144=CARTESIAN_POINT('',(-34.5,4.40457132572236E-15,-59.4));
#55145=CARTESIAN_POINT('Origin',(35.,6.66784336078585E-15,-104.175753233145));
#55146=CARTESIAN_POINT('',(34.5,6.46233547508513E-15,-59.4));
#55147=CARTESIAN_POINT('',(34.5,6.46233547508513E-15,-25.4));
#55148=CARTESIAN_POINT('',(34.5,6.46233547508513E-15,-104.175753233145));
#55149=CARTESIAN_POINT('',(30.9292009086072,4.77048955893622E-15,-25.4));
#55150=CARTESIAN_POINT('',(35.,6.66784336078585E-15,-25.4));
#55151=CARTESIAN_POINT('',(30.9292009086072,4.99468073201678E-15,-59.4));
#55152=CARTESIAN_POINT('',(30.9292009086072,4.99468073201678E-15,-71.4));
#55153=CARTESIAN_POINT('',(35.,6.66784336078585E-15,-59.4));
#55154=CARTESIAN_POINT('Origin',(-0.500000000000025,12.7,-76.7));
#55155=CARTESIAN_POINT('',(-0.500000000000025,13.,-76.7));
#55156=CARTESIAN_POINT('',(-0.500000000000025,13.,-76.7));
#55157=CARTESIAN_POINT('',(-0.500000000000025,12.7,-76.7));
#55158=CARTESIAN_POINT('Origin',(0.499999999999986,12.7,-76.7));
#55159=CARTESIAN_POINT('',(0.499999999999986,13.,-76.7));
#55160=CARTESIAN_POINT('',(0.499999999999986,13.,-76.7));
#55161=CARTESIAN_POINT('',(0.499999999999986,12.7,-76.7));
#55162=CARTESIAN_POINT('Origin',(-1.50786351795467E-14,12.7,-76.7));
#55163=CARTESIAN_POINT('Origin',(-1.54689479616415E-14,13.,-76.7));
#55164=CARTESIAN_POINT('Origin',(-30.9292009086072,-2.,-104.175753233145));
#55165=CARTESIAN_POINT('',(-28.9973492560291,-1.48236190979496,-25.4));
#55166=CARTESIAN_POINT('Origin',(-30.9292009086072,-2.,-25.4));
#55167=CARTESIAN_POINT('',(-28.9973492560291,-1.48236190979496,-59.4));
#55168=CARTESIAN_POINT('Origin',(-30.9292009086072,-2.,-59.4));
#55169=CARTESIAN_POINT('',(-28.9973492560291,-1.48236190979496,-71.4));
#55170=CARTESIAN_POINT('Origin',(0.,0.,-25.4));
#55171=CARTESIAN_POINT('',(-25.7,-13.788236863595,-25.4));
#55172=CARTESIAN_POINT('',(-29.3945469326493,4.36391374425416E-15,-25.4));
#55173=CARTESIAN_POINT('',(-25.7,0.500000000000004,-25.4));
#55174=CARTESIAN_POINT('',(-25.7,-16.5,-25.4));
#55175=CARTESIAN_POINT('',(-34.5,0.500000000000005,-25.4));
#55176=CARTESIAN_POINT('',(-25.7,0.500000000000004,-25.4));
#55177=CARTESIAN_POINT('',(-34.5,0.500000000000005,-25.4));
#55178=CARTESIAN_POINT('Origin',(-25.7,-16.5,-25.4));
#55179=CARTESIAN_POINT('',(-25.7,-13.788236863595,-24.6339201514178));
#55180=CARTESIAN_POINT('',(-25.7,-13.788236863595,-104.175753233145));
#55181=CARTESIAN_POINT('',(-25.7,0.500000000000004,-24.6339201514178));
#55182=CARTESIAN_POINT('',(-25.7,24.2065391822594,-24.6339201514178));
#55183=CARTESIAN_POINT('',(-25.7,0.500000000000004,-25.4));
#55184=CARTESIAN_POINT('Origin',(25.7,0.500000000000004,-25.4));
#55185=CARTESIAN_POINT('',(25.7,0.500000000000004,-25.4));
#55186=CARTESIAN_POINT('',(25.7,0.499999999999997,-24.6339201514179));
#55187=CARTESIAN_POINT('',(25.7,0.500000000000004,-25.4));
#55188=CARTESIAN_POINT('',(25.7,-13.788236863595,-24.6339201514178));
#55189=CARTESIAN_POINT('',(25.7,24.2065391822594,-24.6339201514179));
#55190=CARTESIAN_POINT('',(25.7,-13.788236863595,-25.4));
#55191=CARTESIAN_POINT('',(25.7,-13.788236863595,-104.175753233145));
#55192=CARTESIAN_POINT('',(25.7,0.500000000000004,-25.4));
#55193=CARTESIAN_POINT('Origin',(0.,0.,-25.4));
#55194=CARTESIAN_POINT('',(28.9973492560291,-1.48236190979496,-25.4));
#55195=CARTESIAN_POINT('',(29.3945469326493,4.36391374425416E-15,-25.4));
#55196=CARTESIAN_POINT('Origin',(30.9292009086072,-2.,-25.4));
#55197=CARTESIAN_POINT('',(35.,0.500000000000005,-25.4));
#55198=CARTESIAN_POINT('',(34.5,6.46233547508513E-15,-25.4));
#55199=CARTESIAN_POINT('',(35.,0.500000000000005,-25.4));
#55200=CARTESIAN_POINT('Origin',(30.9292009086072,-2.,-104.175753233145));
#55201=CARTESIAN_POINT('',(28.9973492560291,-1.48236190979496,-59.4));
#55202=CARTESIAN_POINT('',(28.9973492560291,-1.48236190979496,-13.4));
#55203=CARTESIAN_POINT('Origin',(30.9292009086072,-2.,-59.4));
#55204=CARTESIAN_POINT('Origin',(-8.55,-12.0328932188134,-3.45));
#55205=CARTESIAN_POINT('',(12.3307106781187,-16.45,-3.45));
#55206=CARTESIAN_POINT('',(22.1792893218814,-16.45,-3.45));
#55207=CARTESIAN_POINT('',(12.3307106781187,-16.45,-3.45));
#55208=CARTESIAN_POINT('',(23.15,-15.4792893218813,-3.45));
#55209=CARTESIAN_POINT('',(22.1792893218814,-16.45,-3.45));
#55210=CARTESIAN_POINT('',(23.15,11.9792893218814,-3.45));
#55211=CARTESIAN_POINT('',(23.15,-15.4792893218813,-3.45));
#55212=CARTESIAN_POINT('',(22.1792893218813,12.95,-3.45));
#55213=CARTESIAN_POINT('',(23.15,11.9792893218814,-3.45));
#55214=CARTESIAN_POINT('',(-22.1792893218813,12.95,-3.45));
#55215=CARTESIAN_POINT('',(22.1792893218813,12.95,-3.45));
#55216=CARTESIAN_POINT('',(-23.15,11.9792893218814,-3.45));
#55217=CARTESIAN_POINT('',(-22.1792893218813,12.95,-3.45));
#55218=CARTESIAN_POINT('',(-23.15,-15.4792893218813,-3.45));
#55219=CARTESIAN_POINT('',(-23.15,11.9792893218814,-3.45));
#55220=CARTESIAN_POINT('',(-22.1792893218814,-16.45,-3.45));
#55221=CARTESIAN_POINT('',(-23.15,-15.4792893218813,-3.45));
#55222=CARTESIAN_POINT('',(-12.3307106781186,-16.45,-3.45));
#55223=CARTESIAN_POINT('',(-22.1792893218814,-16.45,-3.45));
#55224=CARTESIAN_POINT('',(-8.23180194846605,-12.3510912703474,-3.45));
#55225=CARTESIAN_POINT('',(-12.3307106781186,-16.45,-3.45));
#55226=CARTESIAN_POINT('',(-8.1,-12.0328932188134,-3.45));
#55227=CARTESIAN_POINT('Origin',(-8.55,-12.0328932188134,-3.45));
#55228=CARTESIAN_POINT('',(-8.1,-8.40710678118654,-3.45));
#55229=CARTESIAN_POINT('',(-8.1,-12.0328932188134,-3.45));
#55230=CARTESIAN_POINT('',(-8.23180194846605,-8.0889087296526,-3.45));
#55231=CARTESIAN_POINT('Origin',(-8.55,-8.40710678118654,-3.45));
#55232=CARTESIAN_POINT('',(-8.60795233719346,-7.7127583409252,-3.45));
#55233=CARTESIAN_POINT('',(-8.23180194846605,-8.0889087296526,-3.45));
#55234=CARTESIAN_POINT('',(-8.76432075605962,-7.39577200905833,-3.45));
#55235=CARTESIAN_POINT('Origin',(-8.21904360754086,-7.32384961127259,-3.45));
#55236=CARTESIAN_POINT('',(-10.7007720090583,-5.45932075605962,-3.45));
#55237=CARTESIAN_POINT('Origin',(-10.995,-7.69,-3.45));
#55238=CARTESIAN_POINT('',(-11.0177583409252,-5.30295233719346,-3.45));
#55239=CARTESIAN_POINT('Origin',(-10.6288496112726,-4.91404360754086,-3.45));
#55240=CARTESIAN_POINT('',(-11.3889087296526,-4.93180194846607,-3.45));
#55241=CARTESIAN_POINT('',(-11.0177583409252,-5.30295233719346,-3.45));
#55242=CARTESIAN_POINT('',(-11.55,-4.54289321881346,-3.45));
#55243=CARTESIAN_POINT('Origin',(-11.,-4.54289321881346,-3.45));
#55244=CARTESIAN_POINT('',(-11.55,-3.65710678118656,-3.45));
#55245=CARTESIAN_POINT('',(-11.55,-4.54289321881346,-3.45));
#55246=CARTESIAN_POINT('',(-11.3889087296526,-3.26819805153396,-3.45));
#55247=CARTESIAN_POINT('Origin',(-11.,-3.65710678118656,-3.45));
#55248=CARTESIAN_POINT('',(-11.0177583409252,-2.89704766280654,-3.45));
#55249=CARTESIAN_POINT('',(-11.3889087296526,-3.26819805153396,-3.45));
#55250=CARTESIAN_POINT('',(-10.7007720090583,-2.74067924394038,-3.45));
#55251=CARTESIAN_POINT('Origin',(-10.6288496112726,-3.28595639245914,-3.45));
#55252=CARTESIAN_POINT('',(-8.76432075605962,-0.804227990941668,-3.45));
#55253=CARTESIAN_POINT('Origin',(-10.995,-0.510000000000002,-3.45));
#55254=CARTESIAN_POINT('',(-8.60795233719346,-0.48724165907481,-3.45));
#55255=CARTESIAN_POINT('Origin',(-8.21904360754086,-0.87615038872741,-3.45));
#55256=CARTESIAN_POINT('',(-8.07071067811865,0.0499999999999998,-3.45));
#55257=CARTESIAN_POINT('',(-8.60795233719346,-0.487241659074809,-3.45));
#55258=CARTESIAN_POINT('',(8.07071067811865,0.0500000000000006,-3.45));
#55259=CARTESIAN_POINT('',(-8.07071067811865,0.0499999999999998,-3.45));
#55260=CARTESIAN_POINT('',(8.60795233719346,-0.487241659074806,-3.45));
#55261=CARTESIAN_POINT('',(8.07071067811865,0.0500000000000006,-3.45));
#55262=CARTESIAN_POINT('',(8.76432075605962,-0.804227990941667,-3.45));
#55263=CARTESIAN_POINT('Origin',(8.21904360754086,-0.876150388727407,-3.45));
#55264=CARTESIAN_POINT('',(10.7007720090583,-2.74067924394038,-3.45));
#55265=CARTESIAN_POINT('Origin',(10.995,-0.509999999999999,-3.45));
#55266=CARTESIAN_POINT('',(11.0177583409252,-2.89704766280654,-3.45));
#55267=CARTESIAN_POINT('Origin',(10.6288496112726,-3.28595639245914,-3.45));
#55268=CARTESIAN_POINT('',(11.3889087296526,-3.26819805153396,-3.45));
#55269=CARTESIAN_POINT('',(11.0177583409252,-2.89704766280654,-3.45));
#55270=CARTESIAN_POINT('',(11.55,-3.65710678118656,-3.45));
#55271=CARTESIAN_POINT('Origin',(11.,-3.65710678118656,-3.45));
#55272=CARTESIAN_POINT('',(11.55,-4.54289321881346,-3.45));
#55273=CARTESIAN_POINT('',(11.55,-3.65710678118656,-3.45));
#55274=CARTESIAN_POINT('',(11.3889087296526,-4.93180194846606,-3.45));
#55275=CARTESIAN_POINT('Origin',(11.,-4.54289321881346,-3.45));
#55276=CARTESIAN_POINT('',(11.0177583409252,-5.30295233719346,-3.45));
#55277=CARTESIAN_POINT('',(11.3889087296526,-4.93180194846606,-3.45));
#55278=CARTESIAN_POINT('',(10.7007720090583,-5.45932075605962,-3.45));
#55279=CARTESIAN_POINT('Origin',(10.6288496112726,-4.91404360754086,-3.45));
#55280=CARTESIAN_POINT('',(8.76432075605962,-7.39577200905833,-3.45));
#55281=CARTESIAN_POINT('Origin',(10.995,-7.69,-3.45));
#55282=CARTESIAN_POINT('',(8.60795233719346,-7.71275834092519,-3.45));
#55283=CARTESIAN_POINT('Origin',(8.21904360754086,-7.32384961127259,-3.45));
#55284=CARTESIAN_POINT('',(8.23180194846606,-8.08890872965259,-3.45));
#55285=CARTESIAN_POINT('',(8.60795233719346,-7.71275834092519,-3.45));
#55286=CARTESIAN_POINT('',(8.1,-8.40710678118654,-3.45));
#55287=CARTESIAN_POINT('Origin',(8.55,-8.40710678118654,-3.45));
#55288=CARTESIAN_POINT('',(8.1,-12.0328932188134,-3.45));
#55289=CARTESIAN_POINT('',(8.1,-8.40710678118654,-3.45));
#55290=CARTESIAN_POINT('',(8.23180194846605,-12.3510912703474,-3.45));
#55291=CARTESIAN_POINT('Origin',(8.55,-12.0328932188134,-3.45));
#55292=CARTESIAN_POINT('',(8.23180194846605,-12.3510912703474,-3.45));
#55293=CARTESIAN_POINT('Origin',(34.5,6.46233547508513E-15,-104.175753233145));
#55294=CARTESIAN_POINT('',(35.,0.500000000000005,-59.4));
#55295=CARTESIAN_POINT('',(35.,0.500000000000007,-104.175753233145));
#55296=CARTESIAN_POINT('',(34.5,6.46233547508513E-15,-59.4));
#55297=CARTESIAN_POINT('Origin',(-34.5,0.500000000000005,-104.175753233145));
#55298=CARTESIAN_POINT('',(-34.5,0.500000000000005,-59.4));
#55299=CARTESIAN_POINT('',(-34.5,0.500000000000005,-104.175753233145));
#55300=CARTESIAN_POINT('',(-34.5,0.500000000000005,-59.4));
#55301=CARTESIAN_POINT('Origin',(0.,0.,-59.4));
#55302=CARTESIAN_POINT('',(-25.7,0.500000000000004,-59.4));
#55303=CARTESIAN_POINT('',(-25.7,-13.788236863595,-59.4));
#55304=CARTESIAN_POINT('',(-25.7,0.500000000000004,-59.4));
#55305=CARTESIAN_POINT('',(-29.3945469326493,4.36391374425416E-15,-59.4));
#55306=CARTESIAN_POINT('',(-35.,0.500000000000005,-59.4));
#55307=CARTESIAN_POINT('Origin',(-25.7,0.500000000000004,-59.4));
#55308=CARTESIAN_POINT('',(-25.7,0.500000000000004,-60.1660798485821));
#55309=CARTESIAN_POINT('',(-25.7,0.500000000000004,-59.4));
#55310=CARTESIAN_POINT('',(-25.7,-13.788236863595,-60.1660798485821));
#55311=CARTESIAN_POINT('',(-25.7,24.2065391822594,-60.1660798485822));
#55312=CARTESIAN_POINT('',(-25.7,-13.788236863595,-104.175753233145));
#55313=CARTESIAN_POINT('Origin',(0.,0.,-59.4));
#55314=CARTESIAN_POINT('',(25.7,0.500000000000004,-59.4));
#55315=CARTESIAN_POINT('',(35.,0.500000000000005,-59.4));
#55316=CARTESIAN_POINT('',(25.7,-13.788236863595,-59.4));
#55317=CARTESIAN_POINT('',(29.3945469326493,4.36391374425416E-15,-59.4));
#55318=CARTESIAN_POINT('',(25.7,0.500000000000004,-59.4));
#55319=CARTESIAN_POINT('Origin',(25.7,0.500000000000004,-59.4));
#55320=CARTESIAN_POINT('',(25.7,-13.788236863595,-60.1660798485821));
#55321=CARTESIAN_POINT('',(25.7,-13.788236863595,-104.175753233145));
#55322=CARTESIAN_POINT('',(25.7,0.499999999999997,-60.1660798485821));
#55323=CARTESIAN_POINT('',(25.7,24.2065391822594,-60.1660798485821));
#55324=CARTESIAN_POINT('',(25.7,0.500000000000004,-59.4));
#55325=CARTESIAN_POINT('Origin',(-1.54689479616415E-14,13.,-76.7));
#55326=CARTESIAN_POINT('Origin',(-29.3945469326493,4.36391374425416E-15,
-104.175753233145));
#55327=CARTESIAN_POINT('Origin',(-28.5,-3.33849460240199,-64.9));
#55328=CARTESIAN_POINT('Origin',(-28.5,-3.33849460240201,-19.9));
#55329=CARTESIAN_POINT('Origin',(35.,0.500000000000005,-25.4));
#55330=CARTESIAN_POINT('',(25.7,0.499999999999997,-15.1660798485821));
#55331=CARTESIAN_POINT('Origin',(28.5,0.499999999999997,-19.9));
#55332=CARTESIAN_POINT('',(35.,0.500000000000005,-13.4));
#55333=CARTESIAN_POINT('',(35.,0.500000000000007,-104.175753233145));
#55334=CARTESIAN_POINT('',(25.7,0.500000000000004,-13.4));
#55335=CARTESIAN_POINT('',(35.,0.500000000000005,-13.4));
#55336=CARTESIAN_POINT('',(25.7,0.500000000000004,-25.4));
#55337=CARTESIAN_POINT('Origin',(25.7,0.500000000000004,-25.4));
#55338=CARTESIAN_POINT('',(25.7,-13.788236863595,-13.4));
#55339=CARTESIAN_POINT('',(25.7,-13.788236863595,-15.1660798485821));
#55340=CARTESIAN_POINT('',(25.7,-13.788236863595,-104.175753233145));
#55341=CARTESIAN_POINT('',(25.7,24.2065391822594,-15.1660798485821));
#55342=CARTESIAN_POINT('',(25.7,0.500000000000004,-13.4));
#55343=CARTESIAN_POINT('Origin',(-29.3945469326493,4.36391374425416E-15,
-104.175753233145));
#55344=CARTESIAN_POINT('',(-25.7,-13.788236863595,-15.1660798485821));
#55345=CARTESIAN_POINT('Origin',(-28.5,-3.33849460240201,-19.9));
#55346=CARTESIAN_POINT('',(-25.7,-13.788236863595,-13.4));
#55347=CARTESIAN_POINT('',(-29.3945469326493,4.36391374425416E-15,-13.4));
#55348=CARTESIAN_POINT('',(-25.7,-13.788236863595,-104.175753233145));
#55349=CARTESIAN_POINT('Origin',(-25.7,-16.5,-25.4));
#55350=CARTESIAN_POINT('',(-25.7,0.500000000000004,-15.1660798485822));
#55351=CARTESIAN_POINT('',(-25.7,0.500000000000004,-13.4));
#55352=CARTESIAN_POINT('',(-25.7,0.500000000000004,-25.4));
#55353=CARTESIAN_POINT('',(-25.7,24.2065391822594,-15.1660798485822));
#55354=CARTESIAN_POINT('',(-25.7,-16.5,-13.4));
#55355=CARTESIAN_POINT('Origin',(-25.7,0.500000000000004,-25.4));
#55356=CARTESIAN_POINT('',(-34.5,0.500000000000005,-13.4));
#55357=CARTESIAN_POINT('',(-25.7,0.500000000000004,-13.4));
#55358=CARTESIAN_POINT('',(-34.5,0.500000000000005,-104.175753233145));
#55359=CARTESIAN_POINT('Origin',(-28.5,0.500000000000004,-19.9));
#55360=CARTESIAN_POINT('Origin',(29.3945469326493,4.36391374425416E-15,
-104.175753233145));
#55361=CARTESIAN_POINT('',(25.4958861827765,-14.55,-15.2929076226792));
#55362=CARTESIAN_POINT('Origin',(28.5,-3.33849460240214,-19.9));
#55363=CARTESIAN_POINT('',(25.4958861827765,-14.55,-13.4));
#55364=CARTESIAN_POINT('',(29.3945469326493,4.36391374425416E-15,-13.4));
#55365=CARTESIAN_POINT('',(25.4958861827765,-14.55,-104.175753233145));
#55366=CARTESIAN_POINT('Origin',(29.3945469326493,4.36391374425416E-15,
-104.175753233145));
#55367=CARTESIAN_POINT('Origin',(28.5,-3.33849460240214,-64.9));
#55368=CARTESIAN_POINT('Origin',(28.5,-3.33849460240214,-19.9));
#55369=CARTESIAN_POINT('Origin',(12.3307106781187,-16.45,-3.45));
#55370=CARTESIAN_POINT('',(12.3307106781187,-16.45,-3.5));
#55371=CARTESIAN_POINT('',(22.1792893218814,-16.45,-3.5));
#55372=CARTESIAN_POINT('',(12.3307106781187,-16.45,-3.5));
#55373=CARTESIAN_POINT('',(22.1792893218814,-16.45,-3.45));
#55374=CARTESIAN_POINT('',(12.3307106781187,-16.45,-3.45));
#55375=CARTESIAN_POINT('Origin',(22.1792893218814,-16.45,-3.45));
#55376=CARTESIAN_POINT('',(23.15,-15.4792893218813,-3.5));
#55377=CARTESIAN_POINT('',(22.1792893218814,-16.45,-3.5));
#55378=CARTESIAN_POINT('',(23.15,-15.4792893218813,-3.45));
#55379=CARTESIAN_POINT('Origin',(23.15,-15.4792893218813,-3.45));
#55380=CARTESIAN_POINT('',(23.15,11.9792893218814,-3.5));
#55381=CARTESIAN_POINT('',(23.15,-15.4792893218813,-3.5));
#55382=CARTESIAN_POINT('',(23.15,11.9792893218814,-3.45));
#55383=CARTESIAN_POINT('Origin',(23.15,11.9792893218814,-3.45));
#55384=CARTESIAN_POINT('',(22.1792893218813,12.95,-3.5));
#55385=CARTESIAN_POINT('',(23.15,11.9792893218814,-3.5));
#55386=CARTESIAN_POINT('',(22.1792893218813,12.95,-3.45));
#55387=CARTESIAN_POINT('Origin',(22.1792893218813,12.95,-3.45));
#55388=CARTESIAN_POINT('',(-22.1792893218813,12.95,-3.5));
#55389=CARTESIAN_POINT('',(22.1792893218813,12.95,-3.5));
#55390=CARTESIAN_POINT('',(-22.1792893218813,12.95,-3.45));
#55391=CARTESIAN_POINT('Origin',(-22.1792893218813,12.95,-3.45));
#55392=CARTESIAN_POINT('',(-23.15,11.9792893218814,-3.5));
#55393=CARTESIAN_POINT('',(-22.1792893218813,12.95,-3.5));
#55394=CARTESIAN_POINT('',(-23.15,11.9792893218814,-3.45));
#55395=CARTESIAN_POINT('Origin',(-23.15,11.9792893218814,-3.45));
#55396=CARTESIAN_POINT('',(-23.15,-15.4792893218813,-3.5));
#55397=CARTESIAN_POINT('',(-23.15,11.9792893218814,-3.5));
#55398=CARTESIAN_POINT('',(-23.15,-15.4792893218813,-3.45));
#55399=CARTESIAN_POINT('Origin',(-23.15,-15.4792893218813,-3.45));
#55400=CARTESIAN_POINT('',(-22.1792893218814,-16.45,-3.5));
#55401=CARTESIAN_POINT('',(-23.15,-15.4792893218813,-3.5));
#55402=CARTESIAN_POINT('',(-22.1792893218814,-16.45,-3.45));
#55403=CARTESIAN_POINT('Origin',(-22.1792893218814,-16.45,-3.45));
#55404=CARTESIAN_POINT('',(-12.3307106781186,-16.45,-3.5));
#55405=CARTESIAN_POINT('',(-22.1792893218814,-16.45,-3.5));
#55406=CARTESIAN_POINT('',(-12.3307106781186,-16.45,-3.45));
#55407=CARTESIAN_POINT('Origin',(-12.3307106781186,-16.45,-3.45));
#55408=CARTESIAN_POINT('',(-8.23180194846605,-12.3510912703474,-3.5));
#55409=CARTESIAN_POINT('',(-12.3307106781186,-16.45,-3.5));
#55410=CARTESIAN_POINT('',(-8.23180194846605,-12.3510912703474,-3.45));
#55411=CARTESIAN_POINT('Origin',(-8.55,-12.0328932188134,-3.45));
#55412=CARTESIAN_POINT('',(-8.1,-12.0328932188134,-3.5));
#55413=CARTESIAN_POINT('Origin',(-8.55,-12.0328932188134,-3.5));
#55414=CARTESIAN_POINT('',(-8.1,-12.0328932188134,-3.45));
#55415=CARTESIAN_POINT('Origin',(-8.1,-12.0328932188134,-3.45));
#55416=CARTESIAN_POINT('',(-8.1,-8.40710678118654,-3.5));
#55417=CARTESIAN_POINT('',(-8.1,-12.0328932188134,-3.5));
#55418=CARTESIAN_POINT('',(-8.1,-8.40710678118654,-3.45));
#55419=CARTESIAN_POINT('Origin',(-8.55,-8.40710678118654,-3.45));
#55420=CARTESIAN_POINT('',(-8.23180194846605,-8.0889087296526,-3.5));
#55421=CARTESIAN_POINT('Origin',(-8.55,-8.40710678118654,-3.5));
#55422=CARTESIAN_POINT('',(-8.23180194846605,-8.0889087296526,-3.45));
#55423=CARTESIAN_POINT('Origin',(-8.23180194846605,-8.0889087296526,-3.45));
#55424=CARTESIAN_POINT('',(-8.60795233719346,-7.7127583409252,-3.5));
#55425=CARTESIAN_POINT('',(-8.23180194846605,-8.0889087296526,-3.5));
#55426=CARTESIAN_POINT('',(-8.60795233719346,-7.7127583409252,-3.45));
#55427=CARTESIAN_POINT('Origin',(-8.21904360754086,-7.32384961127259,-3.45));
#55428=CARTESIAN_POINT('',(-8.76432075605962,-7.39577200905833,-3.5));
#55429=CARTESIAN_POINT('Origin',(-8.21904360754086,-7.32384961127259,-3.5));
#55430=CARTESIAN_POINT('',(-8.76432075605962,-7.39577200905833,-3.45));
#55431=CARTESIAN_POINT('Origin',(-10.995,-7.69,-3.45));
#55432=CARTESIAN_POINT('',(-10.7007720090583,-5.45932075605962,-3.5));
#55433=CARTESIAN_POINT('Origin',(-10.995,-7.69,-3.5));
#55434=CARTESIAN_POINT('',(-10.7007720090583,-5.45932075605962,-3.45));
#55435=CARTESIAN_POINT('Origin',(-10.6288496112726,-4.91404360754086,-3.45));
#55436=CARTESIAN_POINT('',(-11.0177583409252,-5.30295233719346,-3.5));
#55437=CARTESIAN_POINT('Origin',(-10.6288496112726,-4.91404360754086,-3.5));
#55438=CARTESIAN_POINT('',(-11.0177583409252,-5.30295233719346,-3.45));
#55439=CARTESIAN_POINT('Origin',(-11.0177583409252,-5.30295233719346,-3.45));
#55440=CARTESIAN_POINT('',(-11.3889087296526,-4.93180194846607,-3.5));
#55441=CARTESIAN_POINT('',(-11.0177583409252,-5.30295233719346,-3.5));
#55442=CARTESIAN_POINT('',(-11.3889087296526,-4.93180194846607,-3.45));
#55443=CARTESIAN_POINT('Origin',(-11.,-4.54289321881346,-3.45));
#55444=CARTESIAN_POINT('',(-11.55,-4.54289321881346,-3.5));
#55445=CARTESIAN_POINT('Origin',(-11.,-4.54289321881346,-3.5));
#55446=CARTESIAN_POINT('',(-11.55,-4.54289321881346,-3.45));
#55447=CARTESIAN_POINT('Origin',(-11.55,-4.54289321881346,-3.45));
#55448=CARTESIAN_POINT('',(-11.55,-3.65710678118656,-3.5));
#55449=CARTESIAN_POINT('',(-11.55,-4.54289321881346,-3.5));
#55450=CARTESIAN_POINT('',(-11.55,-3.65710678118656,-3.45));
#55451=CARTESIAN_POINT('Origin',(-11.,-3.65710678118656,-3.45));
#55452=CARTESIAN_POINT('',(-11.3889087296526,-3.26819805153396,-3.5));
#55453=CARTESIAN_POINT('Origin',(-11.,-3.65710678118656,-3.5));
#55454=CARTESIAN_POINT('',(-11.3889087296526,-3.26819805153396,-3.45));
#55455=CARTESIAN_POINT('Origin',(-11.3889087296526,-3.26819805153396,-3.45));
#55456=CARTESIAN_POINT('',(-11.0177583409252,-2.89704766280654,-3.5));
#55457=CARTESIAN_POINT('',(-11.3889087296526,-3.26819805153396,-3.5));
#55458=CARTESIAN_POINT('',(-11.0177583409252,-2.89704766280654,-3.45));
#55459=CARTESIAN_POINT('Origin',(-10.6288496112726,-3.28595639245914,-3.45));
#55460=CARTESIAN_POINT('',(-10.7007720090583,-2.74067924394038,-3.5));
#55461=CARTESIAN_POINT('Origin',(-10.6288496112726,-3.28595639245914,-3.5));
#55462=CARTESIAN_POINT('',(-10.7007720090583,-2.74067924394038,-3.45));
#55463=CARTESIAN_POINT('Origin',(-10.995,-0.510000000000002,-3.45));
#55464=CARTESIAN_POINT('',(-8.76432075605962,-0.804227990941668,-3.5));
#55465=CARTESIAN_POINT('Origin',(-10.995,-0.510000000000002,-3.5));
#55466=CARTESIAN_POINT('',(-8.76432075605962,-0.804227990941668,-3.45));
#55467=CARTESIAN_POINT('Origin',(-8.21904360754086,-0.87615038872741,-3.45));
#55468=CARTESIAN_POINT('',(-8.60795233719346,-0.48724165907481,-3.5));
#55469=CARTESIAN_POINT('Origin',(-8.21904360754086,-0.87615038872741,-3.5));
#55470=CARTESIAN_POINT('',(-8.60795233719346,-0.48724165907481,-3.45));
#55471=CARTESIAN_POINT('Origin',(-8.60795233719346,-0.487241659074809,-3.45));
#55472=CARTESIAN_POINT('',(-8.07071067811865,0.0499999999999998,-3.5));
#55473=CARTESIAN_POINT('',(-8.60795233719346,-0.487241659074809,-3.5));
#55474=CARTESIAN_POINT('',(-8.07071067811865,0.0499999999999998,-3.45));
#55475=CARTESIAN_POINT('Origin',(-8.07071067811865,0.0499999999999998,-3.45));
#55476=CARTESIAN_POINT('',(8.07071067811865,0.0500000000000006,-3.5));
#55477=CARTESIAN_POINT('',(-8.07071067811865,0.0499999999999998,-3.5));
#55478=CARTESIAN_POINT('',(8.07071067811865,0.0500000000000006,-3.45));
#55479=CARTESIAN_POINT('Origin',(8.07071067811865,0.0500000000000006,-3.45));
#55480=CARTESIAN_POINT('',(8.60795233719346,-0.487241659074806,-3.5));
#55481=CARTESIAN_POINT('',(8.07071067811865,0.0500000000000006,-3.5));
#55482=CARTESIAN_POINT('',(8.60795233719346,-0.487241659074806,-3.45));
#55483=CARTESIAN_POINT('Origin',(8.21904360754086,-0.876150388727407,-3.45));
#55484=CARTESIAN_POINT('',(8.76432075605962,-0.804227990941667,-3.5));
#55485=CARTESIAN_POINT('Origin',(8.21904360754086,-0.876150388727407,-3.5));
#55486=CARTESIAN_POINT('',(8.76432075605962,-0.804227990941667,-3.45));
#55487=CARTESIAN_POINT('Origin',(10.995,-0.509999999999999,-3.45));
#55488=CARTESIAN_POINT('',(10.7007720090583,-2.74067924394038,-3.5));
#55489=CARTESIAN_POINT('Origin',(10.995,-0.509999999999999,-3.5));
#55490=CARTESIAN_POINT('',(10.7007720090583,-2.74067924394038,-3.45));
#55491=CARTESIAN_POINT('Origin',(10.6288496112726,-3.28595639245914,-3.45));
#55492=CARTESIAN_POINT('',(11.0177583409252,-2.89704766280654,-3.5));
#55493=CARTESIAN_POINT('Origin',(10.6288496112726,-3.28595639245914,-3.5));
#55494=CARTESIAN_POINT('',(11.0177583409252,-2.89704766280654,-3.45));
#55495=CARTESIAN_POINT('Origin',(11.0177583409252,-2.89704766280654,-3.45));
#55496=CARTESIAN_POINT('',(11.3889087296526,-3.26819805153396,-3.5));
#55497=CARTESIAN_POINT('',(11.0177583409252,-2.89704766280654,-3.5));
#55498=CARTESIAN_POINT('',(11.3889087296526,-3.26819805153396,-3.45));
#55499=CARTESIAN_POINT('Origin',(11.,-3.65710678118656,-3.45));
#55500=CARTESIAN_POINT('',(11.55,-3.65710678118656,-3.5));
#55501=CARTESIAN_POINT('Origin',(11.,-3.65710678118656,-3.5));
#55502=CARTESIAN_POINT('',(11.55,-3.65710678118656,-3.45));
#55503=CARTESIAN_POINT('Origin',(11.55,-3.65710678118656,-3.45));
#55504=CARTESIAN_POINT('',(11.55,-4.54289321881346,-3.5));
#55505=CARTESIAN_POINT('',(11.55,-3.65710678118656,-3.5));
#55506=CARTESIAN_POINT('',(11.55,-4.54289321881346,-3.45));
#55507=CARTESIAN_POINT('Origin',(11.,-4.54289321881346,-3.45));
#55508=CARTESIAN_POINT('',(11.3889087296526,-4.93180194846606,-3.5));
#55509=CARTESIAN_POINT('Origin',(11.,-4.54289321881346,-3.5));
#55510=CARTESIAN_POINT('',(11.3889087296526,-4.93180194846606,-3.45));
#55511=CARTESIAN_POINT('Origin',(11.3889087296526,-4.93180194846606,-3.45));
#55512=CARTESIAN_POINT('',(11.0177583409252,-5.30295233719346,-3.5));
#55513=CARTESIAN_POINT('',(11.3889087296526,-4.93180194846606,-3.5));
#55514=CARTESIAN_POINT('',(11.0177583409252,-5.30295233719346,-3.45));
#55515=CARTESIAN_POINT('Origin',(10.6288496112726,-4.91404360754086,-3.45));
#55516=CARTESIAN_POINT('',(10.7007720090583,-5.45932075605962,-3.5));
#55517=CARTESIAN_POINT('Origin',(10.6288496112726,-4.91404360754086,-3.5));
#55518=CARTESIAN_POINT('',(10.7007720090583,-5.45932075605962,-3.45));
#55519=CARTESIAN_POINT('Origin',(10.995,-7.69,-3.45));
#55520=CARTESIAN_POINT('',(8.76432075605962,-7.39577200905833,-3.5));
#55521=CARTESIAN_POINT('Origin',(10.995,-7.69,-3.5));
#55522=CARTESIAN_POINT('',(8.76432075605962,-7.39577200905833,-3.45));
#55523=CARTESIAN_POINT('Origin',(8.21904360754086,-7.32384961127259,-3.45));
#55524=CARTESIAN_POINT('',(8.60795233719346,-7.71275834092519,-3.5));
#55525=CARTESIAN_POINT('Origin',(8.21904360754086,-7.32384961127259,-3.5));
#55526=CARTESIAN_POINT('',(8.60795233719346,-7.71275834092519,-3.45));
#55527=CARTESIAN_POINT('Origin',(8.60795233719346,-7.71275834092519,-3.45));
#55528=CARTESIAN_POINT('',(8.23180194846606,-8.08890872965259,-3.5));
#55529=CARTESIAN_POINT('',(8.60795233719346,-7.71275834092519,-3.5));
#55530=CARTESIAN_POINT('',(8.23180194846606,-8.08890872965259,-3.45));
#55531=CARTESIAN_POINT('Origin',(8.55,-8.40710678118654,-3.45));
#55532=CARTESIAN_POINT('',(8.1,-8.40710678118654,-3.5));
#55533=CARTESIAN_POINT('Origin',(8.55,-8.40710678118654,-3.5));
#55534=CARTESIAN_POINT('',(8.1,-8.40710678118654,-3.45));
#55535=CARTESIAN_POINT('Origin',(8.1,-8.40710678118654,-3.45));
#55536=CARTESIAN_POINT('',(8.1,-12.0328932188134,-3.5));
#55537=CARTESIAN_POINT('',(8.1,-8.40710678118654,-3.5));
#55538=CARTESIAN_POINT('',(8.1,-12.0328932188134,-3.45));
#55539=CARTESIAN_POINT('Origin',(8.55,-12.0328932188134,-3.45));
#55540=CARTESIAN_POINT('',(8.23180194846605,-12.3510912703474,-3.5));
#55541=CARTESIAN_POINT('Origin',(8.55,-12.0328932188134,-3.5));
#55542=CARTESIAN_POINT('',(8.23180194846605,-12.3510912703474,-3.45));
#55543=CARTESIAN_POINT('Origin',(8.23180194846605,-12.3510912703474,-3.45));
#55544=CARTESIAN_POINT('',(8.23180194846605,-12.3510912703474,-3.5));
#55545=CARTESIAN_POINT('Origin',(-1.64657055886728E-14,13.8,-1.36260717503886E-30));
#55546=CARTESIAN_POINT('',(-4.99999999999999,13.8,-3.5));
#55547=CARTESIAN_POINT('',(5.00000000000001,13.8,-3.5));
#55548=CARTESIAN_POINT('',(-5.8,13.8,-3.5));
#55549=CARTESIAN_POINT('',(5.,13.8,-13.4));
#55550=CARTESIAN_POINT('',(5.,13.8,-13.4));
#55551=CARTESIAN_POINT('',(-4.99999999999999,13.8,-13.4));
#55552=CARTESIAN_POINT('',(-5.8,13.8,-13.4));
#55553=CARTESIAN_POINT('',(-4.99999999999999,13.8,-3.5));
#55554=CARTESIAN_POINT('Origin',(5.00000000000001,13.8,-2.19030741916265E-15));
#55555=CARTESIAN_POINT('',(5.8,13.,-3.5));
#55556=CARTESIAN_POINT('',(5.00000000000001,13.8,-3.5));
#55557=CARTESIAN_POINT('',(5.8,13.,-13.4));
#55558=CARTESIAN_POINT('',(5.8,13.,-13.4));
#55559=CARTESIAN_POINT('',(5.00000000000001,13.8,-13.4));
#55560=CARTESIAN_POINT('Origin',(-22.2,13.,-13.4));
#55561=CARTESIAN_POINT('',(22.2,13.,-3.5));
#55562=CARTESIAN_POINT('',(22.2,13.,-3.5));
#55563=CARTESIAN_POINT('',(22.2,13.,-13.4));
#55564=CARTESIAN_POINT('',(22.2,13.,-13.4));
#55565=CARTESIAN_POINT('',(-22.2,13.,-13.4));
#55566=CARTESIAN_POINT('Origin',(22.2,13.,-13.4));
#55567=CARTESIAN_POINT('',(23.2,12.,-3.5));
#55568=CARTESIAN_POINT('',(23.2,12.,-3.5));
#55569=CARTESIAN_POINT('',(23.2,12.,-13.4));
#55570=CARTESIAN_POINT('',(23.2,12.,-13.4));
#55571=CARTESIAN_POINT('',(22.2,13.,-13.4));
#55572=CARTESIAN_POINT('Origin',(23.2,12.,-13.4));
#55573=CARTESIAN_POINT('',(23.2,-15.5,-3.5));
#55574=CARTESIAN_POINT('',(23.2,-15.5,-3.5));
#55575=CARTESIAN_POINT('',(23.2,-15.5,-13.4));
#55576=CARTESIAN_POINT('',(23.2,-15.5,-13.4));
#55577=CARTESIAN_POINT('',(23.2,12.,-13.4));
#55578=CARTESIAN_POINT('Origin',(-23.2,12.,-13.4));
#55579=CARTESIAN_POINT('',(-23.2,12.,-3.5));
#55580=CARTESIAN_POINT('',(-23.2,-15.5,-3.5));
#55581=CARTESIAN_POINT('',(-23.2,12.,-3.5));
#55582=CARTESIAN_POINT('',(-23.2,12.,-13.4));
#55583=CARTESIAN_POINT('',(-23.2,12.,-13.4));
#55584=CARTESIAN_POINT('',(-23.2,-15.5,-13.4));
#55585=CARTESIAN_POINT('',(-23.2,12.,-13.4));
#55586=CARTESIAN_POINT('',(-23.2,-15.5,-13.4));
#55587=CARTESIAN_POINT('Origin',(-22.2,13.,-13.4));
#55588=CARTESIAN_POINT('',(-22.2,13.,-3.5));
#55589=CARTESIAN_POINT('',(-22.2,13.,-3.5));
#55590=CARTESIAN_POINT('',(-22.2,13.,-13.4));
#55591=CARTESIAN_POINT('',(-22.2,13.,-13.4));
#55592=CARTESIAN_POINT('',(-22.2,13.,-13.4));
#55593=CARTESIAN_POINT('Origin',(-22.2,13.,-13.4));
#55594=CARTESIAN_POINT('',(-5.8,13.,-3.5));
#55595=CARTESIAN_POINT('',(22.2,13.,-3.5));
#55596=CARTESIAN_POINT('',(-5.8,13.,-13.4));
#55597=CARTESIAN_POINT('',(-5.8,13.,-13.4));
#55598=CARTESIAN_POINT('',(-22.2,13.,-13.4));
#55599=CARTESIAN_POINT('Origin',(-4.99999999999999,13.8,-4.38061483832526E-16));
#55600=CARTESIAN_POINT('',(-4.99999999999999,13.8,-13.4));
#55601=CARTESIAN_POINT('',(-4.99999999999999,13.8,-3.5));
#55602=CARTESIAN_POINT('Origin',(35.,13.,-104.175753233145));
#55603=CARTESIAN_POINT('',(35.,13.,-13.4));
#55604=CARTESIAN_POINT('',(35.,13.,-13.4));
#55605=CARTESIAN_POINT('',(35.,0.500000000000005,-71.4));
#55606=CARTESIAN_POINT('',(35.,0.500000000000005,-59.4));
#55607=CARTESIAN_POINT('',(35.,13.,-71.4));
#55608=CARTESIAN_POINT('',(35.,13.,-71.4));
#55609=CARTESIAN_POINT('',(35.,13.,-104.175753233145));
#55610=CARTESIAN_POINT('Origin',(34.,14.,-104.175753233145));
#55611=CARTESIAN_POINT('',(34.,14.,-71.4));
#55612=CARTESIAN_POINT('',(34.,14.,-71.4));
#55613=CARTESIAN_POINT('',(34.,14.,-13.4));
#55614=CARTESIAN_POINT('',(34.,14.,-104.175753233145));
#55615=CARTESIAN_POINT('',(34.,14.,-13.4));
#55616=CARTESIAN_POINT('Origin',(-23.,14.,-84.8));
#55617=CARTESIAN_POINT('',(17.505,14.,-71.4));
#55618=CARTESIAN_POINT('',(17.505,14.,-13.4));
#55619=CARTESIAN_POINT('',(17.505,14.,-83.0807063142603));
#55620=CARTESIAN_POINT('',(23.,14.,-13.4));
#55621=CARTESIAN_POINT('',(23.,14.,-71.4));
#55622=CARTESIAN_POINT('Origin',(17.005,13.5,-83.0807063142603));
#55623=CARTESIAN_POINT('',(17.005,13.5,-71.4));
#55624=CARTESIAN_POINT('',(17.005,13.5,-13.4));
#55625=CARTESIAN_POINT('',(17.005,13.5,-83.0807063142603));
#55626=CARTESIAN_POINT('',(17.005,13.5,-13.4));
#55627=CARTESIAN_POINT('',(17.005,13.5,-71.4));
#55628=CARTESIAN_POINT('Origin',(17.005,13.5,-83.0807063142603));
#55629=CARTESIAN_POINT('',(6.33500000000001,13.5,-71.4));
#55630=CARTESIAN_POINT('',(6.33500000000001,13.5,-13.4));
#55631=CARTESIAN_POINT('',(6.33500000000001,13.5,-83.0807063142603));
#55632=CARTESIAN_POINT('',(17.005,13.5,-13.4));
#55633=CARTESIAN_POINT('',(17.005,13.5,-71.4));
#55634=CARTESIAN_POINT('Origin',(6.33500000000001,13.5,-83.0807063142603));
#55635=CARTESIAN_POINT('',(5.835,14.,-71.4));
#55636=CARTESIAN_POINT('',(5.835,14.,-13.4));
#55637=CARTESIAN_POINT('',(5.835,14.,-83.0807063142603));
#55638=CARTESIAN_POINT('',(6.33500000000001,13.5,-13.4));
#55639=CARTESIAN_POINT('',(6.33500000000001,13.5,-71.4));
#55640=CARTESIAN_POINT('Origin',(-23.,14.,-84.8));
#55641=CARTESIAN_POINT('',(-5.835,14.,-71.4));
#55642=CARTESIAN_POINT('',(23.,14.,-71.4));
#55643=CARTESIAN_POINT('',(-5.835,14.,-13.4));
#55644=CARTESIAN_POINT('',(-5.835,14.,-83.0807063142603));
#55645=CARTESIAN_POINT('',(23.,14.,-13.4));
#55646=CARTESIAN_POINT('Origin',(-6.33500000000001,13.5,-83.0807063142603));
#55647=CARTESIAN_POINT('',(-6.33500000000001,13.5,-71.4));
#55648=CARTESIAN_POINT('',(-6.33500000000001,13.5,-13.4));
#55649=CARTESIAN_POINT('',(-6.33500000000001,13.5,-83.0807063142603));
#55650=CARTESIAN_POINT('',(-6.33500000000001,13.5,-13.4));
#55651=CARTESIAN_POINT('',(-6.33500000000001,13.5,-71.4));
#55652=CARTESIAN_POINT('Origin',(-17.005,13.5,-83.0807063142603));
#55653=CARTESIAN_POINT('',(-17.005,13.5,-71.4));
#55654=CARTESIAN_POINT('',(-17.005,13.5,-13.4));
#55655=CARTESIAN_POINT('',(-17.005,13.5,-83.0807063142603));
#55656=CARTESIAN_POINT('',(-17.005,13.5,-13.4));
#55657=CARTESIAN_POINT('',(-17.005,13.5,-71.4));
#55658=CARTESIAN_POINT('Origin',(-17.005,13.5,-83.0807063142603));
#55659=CARTESIAN_POINT('',(-17.505,14.,-71.4));
#55660=CARTESIAN_POINT('',(-17.505,14.,-13.4));
#55661=CARTESIAN_POINT('',(-17.505,14.,-83.0807063142603));
#55662=CARTESIAN_POINT('',(-17.005,13.5,-13.4));
#55663=CARTESIAN_POINT('',(-17.005,13.5,-71.4));
#55664=CARTESIAN_POINT('Origin',(-23.,14.,-84.8));
#55665=CARTESIAN_POINT('',(-34.,14.,-71.4));
#55666=CARTESIAN_POINT('',(23.,14.,-71.4));
#55667=CARTESIAN_POINT('',(-34.,14.,-13.4));
#55668=CARTESIAN_POINT('',(-34.,14.,-104.175753233145));
#55669=CARTESIAN_POINT('',(23.,14.,-13.4));
#55670=CARTESIAN_POINT('Origin',(-34.,14.,-104.175753233145));
#55671=CARTESIAN_POINT('',(-35.,13.,-71.4));
#55672=CARTESIAN_POINT('',(-34.,14.,-71.4));
#55673=CARTESIAN_POINT('',(-35.,13.,-13.4));
#55674=CARTESIAN_POINT('',(-35.,13.,-104.175753233145));
#55675=CARTESIAN_POINT('',(-34.,14.,-13.4));
#55676=CARTESIAN_POINT('Origin',(-35.,13.,-104.175753233145));
#55677=CARTESIAN_POINT('',(-35.,5.6,-71.4));
#55678=CARTESIAN_POINT('',(-35.,13.,-71.4));
#55679=CARTESIAN_POINT('',(-35.,5.6,-13.4));
#55680=CARTESIAN_POINT('',(-35.,5.6,-104.175753233145));
#55681=CARTESIAN_POINT('',(-35.,13.,-13.4));
#55682=CARTESIAN_POINT('Origin',(-35.,5.6,-104.175753233145));
#55683=CARTESIAN_POINT('',(-34.5,5.10000000000001,-71.4));
#55684=CARTESIAN_POINT('',(-35.,5.6,-71.4));
#55685=CARTESIAN_POINT('',(-34.5,5.10000000000001,-13.4));
#55686=CARTESIAN_POINT('',(-34.5,5.10000000000001,-104.175753233145));
#55687=CARTESIAN_POINT('',(-35.,5.6,-13.4));
#55688=CARTESIAN_POINT('Origin',(-34.5,5.10000000000001,-104.175753233145));
#55689=CARTESIAN_POINT('',(-34.5,0.500000000000005,-71.4));
#55690=CARTESIAN_POINT('',(-34.5,5.10000000000001,-71.4));
#55691=CARTESIAN_POINT('',(-34.5,0.500000000000005,-104.175753233145));
#55692=CARTESIAN_POINT('',(-34.5,5.10000000000001,-13.4));
#55693=CARTESIAN_POINT('Origin',(-35.,0.500000000000005,-59.4));
#55694=CARTESIAN_POINT('',(-25.7,0.500000000000004,-69.6339201514178));
#55695=CARTESIAN_POINT('Origin',(-28.5,0.500000000000004,-64.9));
#55696=CARTESIAN_POINT('',(-25.7,0.500000000000004,-71.4));
#55697=CARTESIAN_POINT('',(-35.,0.500000000000005,-71.4));
#55698=CARTESIAN_POINT('',(-25.7,0.500000000000004,-59.4));
#55699=CARTESIAN_POINT('Origin',(-25.7,0.500000000000004,-59.4));
#55700=CARTESIAN_POINT('',(-25.7,-13.788236863595,-71.4));
#55701=CARTESIAN_POINT('',(-25.7,-13.788236863595,-69.6339201514178));
#55702=CARTESIAN_POINT('',(-25.7,-13.788236863595,-104.175753233145));
#55703=CARTESIAN_POINT('',(-25.7,24.2065391822594,-69.6339201514178));
#55704=CARTESIAN_POINT('',(-25.7,0.500000000000004,-71.4));
#55705=CARTESIAN_POINT('Origin',(-29.3945469326493,4.36391374425416E-15,
-104.175753233145));
#55706=CARTESIAN_POINT('',(-25.4958861827765,-14.55,-69.5070923773207));
#55707=CARTESIAN_POINT('Origin',(-28.5,-3.33849460240199,-64.9));
#55708=CARTESIAN_POINT('',(-25.4958861827765,-14.55,-71.4));
#55709=CARTESIAN_POINT('',(-29.3945469326493,4.36391374425416E-15,-71.4));
#55710=CARTESIAN_POINT('',(-25.4958861827765,-14.55,-104.175753233145));
#55711=CARTESIAN_POINT('Origin',(29.3945469326493,4.36391374425416E-15,
-104.175753233145));
#55712=CARTESIAN_POINT('',(25.7,-13.788236863595,-69.6339201514178));
#55713=CARTESIAN_POINT('Origin',(28.5,-3.33849460240214,-64.9));
#55714=CARTESIAN_POINT('',(25.7,-13.788236863595,-71.4));
#55715=CARTESIAN_POINT('',(29.3945469326493,4.36391374425416E-15,-71.4));
#55716=CARTESIAN_POINT('',(25.7,-13.788236863595,-104.175753233145));
#55717=CARTESIAN_POINT('Origin',(25.7,0.500000000000004,-59.4));
#55718=CARTESIAN_POINT('',(25.7,0.499999999999997,-69.6339201514178));
#55719=CARTESIAN_POINT('',(25.7,0.500000000000004,-71.4));
#55720=CARTESIAN_POINT('',(25.7,0.500000000000004,-59.4));
#55721=CARTESIAN_POINT('',(25.7,24.2065391822594,-69.6339201514178));
#55722=CARTESIAN_POINT('',(25.7,0.500000000000004,-71.4));
#55723=CARTESIAN_POINT('Origin',(35.,0.500000000000005,-59.4));
#55724=CARTESIAN_POINT('',(35.,0.500000000000005,-71.4));
#55725=CARTESIAN_POINT('Origin',(28.5,0.499999999999997,-64.9));
#55726=CARTESIAN_POINT('Origin',(-25.4958861827765,-14.55,-104.175753233145));
#55727=CARTESIAN_POINT('Origin',(-28.5000000000034,-12.2029290542103,-64.8999999999982));
#55728=CARTESIAN_POINT('',(-23.,-16.5,-71.4));
#55729=CARTESIAN_POINT('',(-25.4958861827765,-14.55,-71.4));
#55730=CARTESIAN_POINT('',(-23.,-16.5,-84.8));
#55731=CARTESIAN_POINT('Origin',(-23.2,-15.5,-13.4));
#55732=CARTESIAN_POINT('',(-22.2,-16.5,-3.5));
#55733=CARTESIAN_POINT('',(-23.2,-15.5,-3.5));
#55734=CARTESIAN_POINT('',(-22.2,-16.5,-13.4));
#55735=CARTESIAN_POINT('',(-23.2,-15.5,-13.4));
#55736=CARTESIAN_POINT('',(-22.2,-16.5,-13.4));
#55737=CARTESIAN_POINT('Origin',(23.2,-15.5,-13.4));
#55738=CARTESIAN_POINT('',(22.2,-16.5,-3.5));
#55739=CARTESIAN_POINT('',(22.2,-16.5,-3.5));
#55740=CARTESIAN_POINT('',(22.2,-16.5,-13.4));
#55741=CARTESIAN_POINT('',(22.2,-16.5,-13.4));
#55742=CARTESIAN_POINT('',(23.2,-15.5,-13.4));
#55743=CARTESIAN_POINT('Origin',(0.,0.,-13.4));
#55744=CARTESIAN_POINT('',(-23.,-16.5,-13.4));
#55745=CARTESIAN_POINT('',(23.,-16.5,-13.4));
#55746=CARTESIAN_POINT('',(22.2,-16.5,-13.4));
#55747=CARTESIAN_POINT('',(25.4958861827765,-14.55,-13.4));
#55748=CARTESIAN_POINT('Origin',(25.4958861827765,-14.55,-104.175753233145));
#55749=CARTESIAN_POINT('Origin',(28.5000000000021,-12.2029290542113,-19.9000000000011));
#55750=CARTESIAN_POINT('',(23.,-16.5,-84.8));
#55751=CARTESIAN_POINT('Origin',(-5.8,13.8,-3.5));
#55752=CARTESIAN_POINT('',(-12.31,-16.5,-3.5));
#55753=CARTESIAN_POINT('',(-22.2,-16.5,-3.5));
#55754=CARTESIAN_POINT('',(-8.19644660940672,-12.3864466094067,-3.5));
#55755=CARTESIAN_POINT('',(-12.31,-16.5,-3.5));
#55756=CARTESIAN_POINT('',(-8.05,-12.0328932188134,-3.5));
#55757=CARTESIAN_POINT('Origin',(-8.55,-12.0328932188134,-3.5));
#55758=CARTESIAN_POINT('',(-8.05,-8.40710678118654,-3.5));
#55759=CARTESIAN_POINT('',(-8.05,-12.0328932188134,-3.5));
#55760=CARTESIAN_POINT('',(-8.19644660940673,-8.05355339059327,-3.5));
#55761=CARTESIAN_POINT('Origin',(-8.55,-8.40710678118654,-3.5));
#55762=CARTESIAN_POINT('',(-8.57259699813413,-7.67740300186587,-3.5));
#55763=CARTESIAN_POINT('',(-8.19644660940673,-8.05355339059327,-3.5));
#55764=CARTESIAN_POINT('',(-8.71475010619428,-7.38923360925963,-3.5));
#55765=CARTESIAN_POINT('Origin',(-8.21904360754086,-7.32384961127259,-3.5));
#55766=CARTESIAN_POINT('',(-10.6942336092596,-5.40975010619428,-3.5));
#55767=CARTESIAN_POINT('Origin',(-10.995,-7.69,-3.5));
#55768=CARTESIAN_POINT('',(-10.9824030018659,-5.26759699813413,-3.5));
#55769=CARTESIAN_POINT('Origin',(-10.6288496112726,-4.91404360754086,-3.5));
#55770=CARTESIAN_POINT('',(-11.3535533905933,-4.89644660940674,-3.5));
#55771=CARTESIAN_POINT('',(-10.9824030018659,-5.26759699813413,-3.5));
#55772=CARTESIAN_POINT('',(-11.5,-4.54289321881346,-3.5));
#55773=CARTESIAN_POINT('Origin',(-11.,-4.54289321881346,-3.5));
#55774=CARTESIAN_POINT('',(-11.5,-3.65710678118656,-3.5));
#55775=CARTESIAN_POINT('',(-11.5,-4.54289321881346,-3.5));
#55776=CARTESIAN_POINT('',(-11.3535533905933,-3.30355339059329,-3.5));
#55777=CARTESIAN_POINT('Origin',(-11.,-3.65710678118656,-3.5));
#55778=CARTESIAN_POINT('',(-10.9824030018659,-2.93240300186587,-3.5));
#55779=CARTESIAN_POINT('',(-11.3535533905933,-3.30355339059329,-3.5));
#55780=CARTESIAN_POINT('',(-10.6942336092596,-2.79024989380572,-3.5));
#55781=CARTESIAN_POINT('Origin',(-10.6288496112726,-3.28595639245914,-3.5));
#55782=CARTESIAN_POINT('',(-8.71475010619428,-0.810766390740372,-3.5));
#55783=CARTESIAN_POINT('Origin',(-10.995,-0.510000000000002,-3.5));
#55784=CARTESIAN_POINT('',(-8.57259699813413,-0.522596998134137,-3.5));
#55785=CARTESIAN_POINT('Origin',(-8.21904360754086,-0.87615038872741,-3.5));
#55786=CARTESIAN_POINT('',(-8.05,-1.60428730688303E-15,-3.5));
#55787=CARTESIAN_POINT('',(-8.57259699813413,-0.522596998134137,-3.5));
#55788=CARTESIAN_POINT('',(8.05,3.67394039744206E-16,-3.5));
#55789=CARTESIAN_POINT('',(-8.05,-1.60428730688303E-15,-3.5));
#55790=CARTESIAN_POINT('',(8.57259699813413,-0.522596998134133,-3.5));
#55791=CARTESIAN_POINT('',(8.05,3.67394039744206E-16,-3.5));
#55792=CARTESIAN_POINT('',(8.71475010619428,-0.81076639074037,-3.5));
#55793=CARTESIAN_POINT('Origin',(8.21904360754086,-0.876150388727407,-3.5));
#55794=CARTESIAN_POINT('',(10.6942336092596,-2.79024989380572,-3.5));
#55795=CARTESIAN_POINT('Origin',(10.995,-0.509999999999999,-3.5));
#55796=CARTESIAN_POINT('',(10.9824030018659,-2.93240300186586,-3.5));
#55797=CARTESIAN_POINT('Origin',(10.6288496112726,-3.28595639245914,-3.5));
#55798=CARTESIAN_POINT('',(11.3535533905933,-3.30355339059329,-3.5));
#55799=CARTESIAN_POINT('',(10.9824030018659,-2.93240300186586,-3.5));
#55800=CARTESIAN_POINT('',(11.5,-3.65710678118656,-3.5));
#55801=CARTESIAN_POINT('Origin',(11.,-3.65710678118656,-3.5));
#55802=CARTESIAN_POINT('',(11.5,-4.54289321881346,-3.5));
#55803=CARTESIAN_POINT('',(11.5,-3.65710678118656,-3.5));
#55804=CARTESIAN_POINT('',(11.3535533905933,-4.89644660940673,-3.5));
#55805=CARTESIAN_POINT('Origin',(11.,-4.54289321881346,-3.5));
#55806=CARTESIAN_POINT('',(10.9824030018659,-5.26759699813413,-3.5));
#55807=CARTESIAN_POINT('',(11.3535533905933,-4.89644660940673,-3.5));
#55808=CARTESIAN_POINT('',(10.6942336092596,-5.40975010619428,-3.5));
#55809=CARTESIAN_POINT('Origin',(10.6288496112726,-4.91404360754086,-3.5));
#55810=CARTESIAN_POINT('',(8.71475010619428,-7.38923360925963,-3.5));
#55811=CARTESIAN_POINT('Origin',(10.995,-7.69,-3.5));
#55812=CARTESIAN_POINT('',(8.57259699813413,-7.67740300186587,-3.5));
#55813=CARTESIAN_POINT('Origin',(8.21904360754086,-7.32384961127259,-3.5));
#55814=CARTESIAN_POINT('',(8.19644660940673,-8.05355339059327,-3.5));
#55815=CARTESIAN_POINT('',(8.57259699813413,-7.67740300186587,-3.5));
#55816=CARTESIAN_POINT('',(8.05,-8.40710678118654,-3.5));
#55817=CARTESIAN_POINT('Origin',(8.55,-8.40710678118654,-3.5));
#55818=CARTESIAN_POINT('',(8.05,-12.0328932188134,-3.5));
#55819=CARTESIAN_POINT('',(8.05,-8.40710678118654,-3.5));
#55820=CARTESIAN_POINT('',(8.19644660940673,-12.3864466094067,-3.5));
#55821=CARTESIAN_POINT('Origin',(8.55,-12.0328932188134,-3.5));
#55822=CARTESIAN_POINT('',(12.31,-16.5,-3.5));
#55823=CARTESIAN_POINT('',(8.19644660940673,-12.3864466094067,-3.5));
#55824=CARTESIAN_POINT('',(12.31,-16.5,-3.5));
#55825=CARTESIAN_POINT('Origin',(0.,0.,-71.4));
#55826=CARTESIAN_POINT('',(22.2,-16.5,-71.4));
#55827=CARTESIAN_POINT('',(22.2,-16.5,-71.4));
#55828=CARTESIAN_POINT('',(23.2,-15.5,-71.4));
#55829=CARTESIAN_POINT('',(23.2,-15.5,-71.4));
#55830=CARTESIAN_POINT('',(23.2,12.,-71.4));
#55831=CARTESIAN_POINT('',(23.2,12.,-71.4));
#55832=CARTESIAN_POINT('',(22.2,13.,-71.4));
#55833=CARTESIAN_POINT('',(22.2,13.,-71.4));
#55834=CARTESIAN_POINT('',(5.79999999999999,13.,-71.4));
#55835=CARTESIAN_POINT('',(-22.2,13.,-71.4));
#55836=CARTESIAN_POINT('',(4.99999999999997,13.8,-71.4));
#55837=CARTESIAN_POINT('',(4.99999999999996,13.8,-71.4));
#55838=CARTESIAN_POINT('',(-4.99999999999998,13.8,-71.4));
#55839=CARTESIAN_POINT('',(-5.79999999999999,13.8,-71.4));
#55840=CARTESIAN_POINT('',(-5.79999999999999,13.,-71.4));
#55841=CARTESIAN_POINT('',(-4.99999999999997,13.8,-71.4));
#55842=CARTESIAN_POINT('',(-22.2,13.,-71.4));
#55843=CARTESIAN_POINT('',(-22.2,13.,-71.4));
#55844=CARTESIAN_POINT('',(-23.2,12.,-71.4));
#55845=CARTESIAN_POINT('',(-23.2,12.,-71.4));
#55846=CARTESIAN_POINT('',(-23.2,-15.5,-71.4));
#55847=CARTESIAN_POINT('',(-23.2,-15.5,-71.4));
#55848=CARTESIAN_POINT('',(-22.2,-16.5,-71.4));
#55849=CARTESIAN_POINT('',(-22.2,-16.5,-71.4));
#55850=CARTESIAN_POINT('',(-23.,-16.5,-71.4));
#55851=CARTESIAN_POINT('Origin',(-4.99999999999996,13.8,1.31418445149757E-15));
#55852=CARTESIAN_POINT('',(-5.79999999999999,13.,-81.3));
#55853=CARTESIAN_POINT('',(-4.99999999999999,13.8,-81.3));
#55854=CARTESIAN_POINT('',(-4.99999999999997,13.8,-81.3));
#55855=CARTESIAN_POINT('',(-5.8,13.,-81.3));
#55856=CARTESIAN_POINT('',(-4.99999999999998,13.8,-71.4));
#55857=CARTESIAN_POINT('Origin',(22.2,13.,-84.8));
#55858=CARTESIAN_POINT('',(23.2,12.,-81.3));
#55859=CARTESIAN_POINT('',(22.2,13.,-81.3));
#55860=CARTESIAN_POINT('',(23.2,12.,-81.3));
#55861=CARTESIAN_POINT('',(22.2,13.,-84.8));
#55862=CARTESIAN_POINT('',(23.2,12.,-84.8));
#55863=CARTESIAN_POINT('Origin',(23.2,12.,-84.8));
#55864=CARTESIAN_POINT('',(23.2,-15.5,-81.3));
#55865=CARTESIAN_POINT('',(23.2,-15.5,-81.3));
#55866=CARTESIAN_POINT('',(23.2,-15.5,-84.8));
#55867=CARTESIAN_POINT('Origin',(23.2,-15.5,-84.8));
#55868=CARTESIAN_POINT('',(22.2,-16.5,-81.3));
#55869=CARTESIAN_POINT('',(22.2,-16.5,-81.3));
#55870=CARTESIAN_POINT('',(22.2,-16.5,-84.8));
#55871=CARTESIAN_POINT('Origin',(-22.2,13.,-84.8));
#55872=CARTESIAN_POINT('',(5.8,13.,-81.3));
#55873=CARTESIAN_POINT('',(22.2,13.,-81.3));
#55874=CARTESIAN_POINT('',(5.8,13.,-81.3));
#55875=CARTESIAN_POINT('Origin',(8.55,-12.0328932188134,-84.8));
#55876=CARTESIAN_POINT('',(8.05,-12.0328932188134,-81.3));
#55877=CARTESIAN_POINT('',(8.05,-12.0328932188134,-84.8));
#55878=CARTESIAN_POINT('',(8.19644660940673,-12.3864466094067,-81.3));
#55879=CARTESIAN_POINT('Origin',(8.55,-12.0328932188134,-81.3));
#55880=CARTESIAN_POINT('',(8.19644660940673,-12.3864466094067,-84.8));
#55881=CARTESIAN_POINT('Origin',(8.55,-8.40710678118654,-84.8));
#55882=CARTESIAN_POINT('',(8.19644660940673,-8.05355339059327,-81.3));
#55883=CARTESIAN_POINT('',(8.19644660940673,-8.05355339059327,-84.8));
#55884=CARTESIAN_POINT('',(8.05,-8.40710678118654,-81.3));
#55885=CARTESIAN_POINT('Origin',(8.55,-8.40710678118654,-81.3));
#55886=CARTESIAN_POINT('',(8.05,-8.40710678118654,-84.8));
#55887=CARTESIAN_POINT('Origin',(8.05,-12.24,-84.8));
#55888=CARTESIAN_POINT('',(8.05,-8.40710678118654,-81.3));
#55889=CARTESIAN_POINT('Origin',(12.31,-16.5,-84.8));
#55890=CARTESIAN_POINT('',(12.31,-16.5,-81.3));
#55891=CARTESIAN_POINT('',(8.19644660940673,-12.3864466094067,-81.3));
#55892=CARTESIAN_POINT('',(12.31,-16.5,-84.8));
#55893=CARTESIAN_POINT('Origin',(12.31,-16.5,-84.8));
#55894=CARTESIAN_POINT('',(12.31,-16.5,-81.3));
#55895=CARTESIAN_POINT('Origin',(8.21904360754086,-7.32384961127259,-84.8));
#55896=CARTESIAN_POINT('',(8.71475010619428,-7.38923360925963,-81.3));
#55897=CARTESIAN_POINT('',(8.57259699813413,-7.67740300186587,-81.3));
#55898=CARTESIAN_POINT('Origin',(8.21904360754086,-7.32384961127259,-81.3));
#55899=CARTESIAN_POINT('',(8.57259699813413,-7.67740300186587,-84.8));
#55900=CARTESIAN_POINT('',(8.71475010619428,-7.38923360925963,-84.8));
#55901=CARTESIAN_POINT('Origin',(10.6288496112726,-4.91404360754086,-84.8));
#55902=CARTESIAN_POINT('',(10.9824030018659,-5.26759699813413,-81.3));
#55903=CARTESIAN_POINT('',(10.6942336092596,-5.40975010619428,-81.3));
#55904=CARTESIAN_POINT('Origin',(10.6288496112726,-4.91404360754086,-81.3));
#55905=CARTESIAN_POINT('',(10.6942336092596,-5.40975010619428,-84.8));
#55906=CARTESIAN_POINT('',(10.9824030018659,-5.26759699813413,0.));
#55907=CARTESIAN_POINT('Origin',(10.995,-7.69,-84.8));
#55908=CARTESIAN_POINT('Origin',(10.995,-7.69,-81.3));
#55909=CARTESIAN_POINT('Origin',(11.,-4.54289321881346,-84.8));
#55910=CARTESIAN_POINT('',(11.5,-4.54289321881346,-81.3));
#55911=CARTESIAN_POINT('',(11.3535533905933,-4.89644660940673,-81.3));
#55912=CARTESIAN_POINT('Origin',(11.,-4.54289321881346,-81.3));
#55913=CARTESIAN_POINT('',(11.3535533905933,-4.89644660940673,-84.8));
#55914=CARTESIAN_POINT('',(11.5,-4.54289321881346,0.));
#55915=CARTESIAN_POINT('Origin',(11.,-3.65710678118656,-84.8));
#55916=CARTESIAN_POINT('',(11.3535533905933,-3.30355339059329,-81.3));
#55917=CARTESIAN_POINT('',(11.5,-3.65710678118656,-81.3));
#55918=CARTESIAN_POINT('Origin',(11.,-3.65710678118656,-81.3));
#55919=CARTESIAN_POINT('',(11.5,-3.65710678118656,-84.8));
#55920=CARTESIAN_POINT('',(11.3535533905933,-3.30355339059329,0.));
#55921=CARTESIAN_POINT('Origin',(11.5,-4.75000000000001,-84.8));
#55922=CARTESIAN_POINT('',(11.5,-3.65710678118656,-81.3));
#55923=CARTESIAN_POINT('Origin',(8.05,-8.2,-84.8));
#55924=CARTESIAN_POINT('',(11.3535533905933,-4.89644660940673,-81.3));
#55925=CARTESIAN_POINT('Origin',(10.6288496112726,-3.28595639245914,-84.8));
#55926=CARTESIAN_POINT('',(10.6942336092596,-2.79024989380572,-81.3));
#55927=CARTESIAN_POINT('',(10.9824030018659,-2.93240300186586,-81.3));
#55928=CARTESIAN_POINT('Origin',(10.6288496112726,-3.28595639245914,-81.3));
#55929=CARTESIAN_POINT('',(10.9824030018659,-2.93240300186586,-84.8));
#55930=CARTESIAN_POINT('',(10.6942336092596,-2.79024989380572,-84.8));
#55931=CARTESIAN_POINT('Origin',(8.21904360754086,-0.876150388727407,-84.8));
#55932=CARTESIAN_POINT('',(8.57259699813413,-0.522596998134133,-81.3));
#55933=CARTESIAN_POINT('',(8.71475010619428,-0.81076639074037,-81.3));
#55934=CARTESIAN_POINT('Origin',(8.21904360754086,-0.876150388727407,-81.3));
#55935=CARTESIAN_POINT('',(8.71475010619428,-0.81076639074037,-84.8));
#55936=CARTESIAN_POINT('',(8.57259699813413,-0.522596998134133,0.));
#55937=CARTESIAN_POINT('Origin',(10.995,-0.509999999999999,-84.8));
#55938=CARTESIAN_POINT('Origin',(10.995,-0.509999999999999,-81.3));
#55939=CARTESIAN_POINT('Origin',(8.05,3.67394039744206E-16,-84.8));
#55940=CARTESIAN_POINT('',(-8.05,-1.60428730688303E-15,-81.3));
#55941=CARTESIAN_POINT('',(-8.05,-1.60428730688303E-15,-84.8));
#55942=CARTESIAN_POINT('',(8.05,3.67394039744206E-16,-81.3));
#55943=CARTESIAN_POINT('',(-8.05,-1.60428730688303E-15,-81.3));
#55944=CARTESIAN_POINT('',(8.05,3.67394039744206E-16,-84.8));
#55945=CARTESIAN_POINT('Origin',(8.05,3.67394039744206E-16,-84.8));
#55946=CARTESIAN_POINT('',(8.05,3.67394039744206E-16,-81.3));
#55947=CARTESIAN_POINT('Origin',(-8.21904360754086,-0.87615038872741,-84.8));
#55948=CARTESIAN_POINT('',(-8.71475010619428,-0.810766390740372,-81.3));
#55949=CARTESIAN_POINT('',(-8.57259699813413,-0.522596998134137,-81.3));
#55950=CARTESIAN_POINT('Origin',(-8.21904360754086,-0.87615038872741,-81.3));
#55951=CARTESIAN_POINT('',(-8.57259699813413,-0.522596998134137,-84.8));
#55952=CARTESIAN_POINT('',(-8.71475010619428,-0.810766390740372,-84.8));
#55953=CARTESIAN_POINT('Origin',(-10.6288496112726,-3.28595639245914,-84.8));
#55954=CARTESIAN_POINT('',(-10.9824030018659,-2.93240300186587,-81.3));
#55955=CARTESIAN_POINT('',(-10.6942336092596,-2.79024989380572,-81.3));
#55956=CARTESIAN_POINT('Origin',(-10.6288496112726,-3.28595639245914,-81.3));
#55957=CARTESIAN_POINT('',(-10.6942336092596,-2.79024989380572,-84.8));
#55958=CARTESIAN_POINT('',(-10.9824030018659,-2.93240300186587,0.));
#55959=CARTESIAN_POINT('Origin',(-10.995,-0.510000000000002,-84.8));
#55960=CARTESIAN_POINT('Origin',(-10.995,-0.510000000000002,-81.3));
#55961=CARTESIAN_POINT('Origin',(-11.,-3.65710678118656,-84.8));
#55962=CARTESIAN_POINT('',(-11.5,-3.65710678118656,-81.3));
#55963=CARTESIAN_POINT('',(-11.3535533905933,-3.30355339059329,-81.3));
#55964=CARTESIAN_POINT('Origin',(-11.,-3.65710678118656,-81.3));
#55965=CARTESIAN_POINT('',(-11.3535533905933,-3.30355339059329,-84.8));
#55966=CARTESIAN_POINT('',(-11.5,-3.65710678118656,0.));
#55967=CARTESIAN_POINT('Origin',(-11.,-4.54289321881346,-84.8));
#55968=CARTESIAN_POINT('',(-11.3535533905933,-4.89644660940674,-81.3));
#55969=CARTESIAN_POINT('',(-11.5,-4.54289321881346,-81.3));
#55970=CARTESIAN_POINT('Origin',(-11.,-4.54289321881346,-81.3));
#55971=CARTESIAN_POINT('',(-11.5,-4.54289321881346,-84.8));
#55972=CARTESIAN_POINT('',(-11.3535533905933,-4.89644660940674,0.));
#55973=CARTESIAN_POINT('Origin',(-11.5,-4.75000000000001,-84.8));
#55974=CARTESIAN_POINT('',(-11.5,-4.54289321881346,-81.3));
#55975=CARTESIAN_POINT('Origin',(-8.05,-1.60428730688303E-15,-84.8));
#55976=CARTESIAN_POINT('',(-11.3535533905933,-3.30355339059329,-81.3));
#55977=CARTESIAN_POINT('Origin',(-8.05,-1.60428730688303E-15,-84.8));
#55978=CARTESIAN_POINT('',(-8.57259699813413,-0.522596998134137,-81.3));
#55979=CARTESIAN_POINT('Origin',(-10.6288496112726,-4.91404360754086,-84.8));
#55980=CARTESIAN_POINT('',(-10.6942336092596,-5.40975010619428,-81.3));
#55981=CARTESIAN_POINT('',(-10.9824030018659,-5.26759699813413,-81.3));
#55982=CARTESIAN_POINT('Origin',(-10.6288496112726,-4.91404360754086,-81.3));
#55983=CARTESIAN_POINT('',(-10.9824030018659,-5.26759699813413,-84.8));
#55984=CARTESIAN_POINT('',(-10.6942336092596,-5.40975010619428,-84.8));
#55985=CARTESIAN_POINT('Origin',(-8.21904360754086,-7.32384961127259,-84.8));
#55986=CARTESIAN_POINT('',(-8.57259699813413,-7.67740300186587,-81.3));
#55987=CARTESIAN_POINT('',(-8.71475010619428,-7.38923360925963,-81.3));
#55988=CARTESIAN_POINT('Origin',(-8.21904360754086,-7.32384961127259,-81.3));
#55989=CARTESIAN_POINT('',(-8.71475010619428,-7.38923360925963,-84.8));
#55990=CARTESIAN_POINT('',(-8.57259699813413,-7.67740300186587,0.));
#55991=CARTESIAN_POINT('Origin',(-10.995,-7.69,-84.8));
#55992=CARTESIAN_POINT('Origin',(-10.995,-7.69,-81.3));
#55993=CARTESIAN_POINT('Origin',(-8.55,-8.40710678118654,-84.8));
#55994=CARTESIAN_POINT('',(-8.05,-8.40710678118654,-81.3));
#55995=CARTESIAN_POINT('',(-8.05,-8.40710678118654,-84.8));
#55996=CARTESIAN_POINT('',(-8.19644660940673,-8.05355339059327,-81.3));
#55997=CARTESIAN_POINT('Origin',(-8.55,-8.40710678118654,-81.3));
#55998=CARTESIAN_POINT('',(-8.19644660940673,-8.05355339059327,-84.8));
#55999=CARTESIAN_POINT('Origin',(-8.55,-12.0328932188134,-84.8));
#56000=CARTESIAN_POINT('',(-8.19644660940672,-12.3864466094067,-81.3));
#56001=CARTESIAN_POINT('',(-8.19644660940672,-12.3864466094067,-84.8));
#56002=CARTESIAN_POINT('',(-8.05,-12.0328932188134,-81.3));
#56003=CARTESIAN_POINT('Origin',(-8.55,-12.0328932188134,-81.3));
#56004=CARTESIAN_POINT('',(-8.05,-12.0328932188134,-84.8));
#56005=CARTESIAN_POINT('Origin',(-22.2,-16.5,-84.8));
#56006=CARTESIAN_POINT('',(-23.2,-15.5,-81.3));
#56007=CARTESIAN_POINT('',(-22.2,-16.5,-81.3));
#56008=CARTESIAN_POINT('',(-23.2,-15.5,-81.3));
#56009=CARTESIAN_POINT('',(-22.2,-16.5,-84.8));
#56010=CARTESIAN_POINT('',(-23.2,-15.5,-84.8));
#56011=CARTESIAN_POINT('Origin',(-23.2,-15.5,-84.8));
#56012=CARTESIAN_POINT('',(-23.2,12.,-81.3));
#56013=CARTESIAN_POINT('',(-23.2,12.,-81.3));
#56014=CARTESIAN_POINT('',(-23.2,12.,-84.8));
#56015=CARTESIAN_POINT('Origin',(-23.2,12.,-84.8));
#56016=CARTESIAN_POINT('',(-22.2,13.,-81.3));
#56017=CARTESIAN_POINT('',(-22.2,13.,-81.3));
#56018=CARTESIAN_POINT('',(-22.2,13.,-84.8));
#56019=CARTESIAN_POINT('Origin',(-22.2,13.,-84.8));
#56020=CARTESIAN_POINT('',(22.2,13.,-81.3));
#56021=CARTESIAN_POINT('Origin',(-23.,-16.5,-84.8));
#56022=CARTESIAN_POINT('',(-12.31,-16.5,-81.3));
#56023=CARTESIAN_POINT('',(-22.2,-16.5,-81.3));
#56024=CARTESIAN_POINT('',(-12.31,-16.5,-84.8));
#56025=CARTESIAN_POINT('Origin',(-12.31,-16.5,-84.8));
#56026=CARTESIAN_POINT('',(-12.31,-16.5,-81.3));
#56027=CARTESIAN_POINT('Origin',(-8.05,-12.24,-84.8));
#56028=CARTESIAN_POINT('',(-8.05,-12.0328932188134,-81.3));
#56029=CARTESIAN_POINT('Origin',(-8.05,-8.2,-84.8));
#56030=CARTESIAN_POINT('',(-8.19644660940673,-8.05355339059327,-81.3));
#56031=CARTESIAN_POINT('Origin',(-8.05,-8.2,-84.8));
#56032=CARTESIAN_POINT('',(-10.9824030018659,-5.26759699813413,-81.3));
#56033=CARTESIAN_POINT('Origin',(8.05,3.67394039744206E-16,-84.8));
#56034=CARTESIAN_POINT('',(10.9824030018659,-2.93240300186586,-81.3));
#56035=CARTESIAN_POINT('Origin',(8.05,-8.2,-84.8));
#56036=CARTESIAN_POINT('',(8.57259699813413,-7.67740300186587,-81.3));
#56037=CARTESIAN_POINT('Origin',(4.99999999999995,13.8,1.31418445149758E-15));
#56038=CARTESIAN_POINT('',(4.99999999999997,13.8,-81.3));
#56039=CARTESIAN_POINT('',(4.99999999999996,13.8,-81.3));
#56040=CARTESIAN_POINT('',(4.99999999999997,13.8,-81.3));
#56041=CARTESIAN_POINT('Origin',(-1.64657055886728E-14,13.8,4.08782152511659E-30));
#56042=CARTESIAN_POINT('',(-5.8,13.8,-81.3));
#56043=CARTESIAN_POINT('Origin',(-5.8,13.8,-81.3));
#56044=CARTESIAN_POINT('Origin',(4.99995,13.,-1.));
#56045=CARTESIAN_POINT('',(4.99995,8.,-1.));
#56046=CARTESIAN_POINT('',(4.99995,13.,-1.));
#56047=CARTESIAN_POINT('',(4.99995,8.,-1.));
#56048=CARTESIAN_POINT('Origin',(0.,8.,-1.));
#56049=CARTESIAN_POINT('',(-4.99995,8.,-1.));
#56050=CARTESIAN_POINT('Origin',(0.,8.,-1.));
#56051=CARTESIAN_POINT('',(-4.99995,8.,-1.));
#56052=CARTESIAN_POINT('Origin',(-4.99995,13.,-1.));
#56053=CARTESIAN_POINT('',(-4.99995,13.,-1.));
#56054=CARTESIAN_POINT('Origin',(0.,8.,-1.));
#56055=CARTESIAN_POINT('Origin',(-28.5,24.2065391822594,-19.9));
#56056=CARTESIAN_POINT('Origin',(-28.5,24.2065391822594,-64.9));
#56057=CARTESIAN_POINT('Origin',(28.5,24.2065391822594,-19.9));
#56058=CARTESIAN_POINT('Origin',(28.5,24.2065391822594,-64.9));
#57032=UNCERTAINTY_MEASURE_WITH_UNIT(LENGTH_MEASURE(0.01),#57080,
'DISTANCE_ACCURACY_VALUE',
'Maximum model space distance between geometric entities at asserted c
onnectivities');
#57040=UNCERTAINTY_MEASURE_WITH_UNIT(LENGTH_MEASURE(0.01),#57080,
'DISTANCE_ACCURACY_VALUE',
'Maximum model space distance between geometric entities at asserted c
onnectivities');
#57071=(
GEOMETRIC_REPRESENTATION_CONTEXT(3)
GLOBAL_UNCERTAINTY_ASSIGNED_CONTEXT((#57032))
GLOBAL_UNIT_ASSIGNED_CONTEXT((#57080,#57082,#57083))
REPRESENTATION_CONTEXT('','3D')
);
#57079=(
GEOMETRIC_REPRESENTATION_CONTEXT(3)
GLOBAL_UNCERTAINTY_ASSIGNED_CONTEXT((#57040))
GLOBAL_UNIT_ASSIGNED_CONTEXT((#57080,#57082,#57083))
REPRESENTATION_CONTEXT('','3D')
);
#57080=(
LENGTH_UNIT()
NAMED_UNIT(*)
SI_UNIT(.MILLI.,.METRE.)
);
#57082=(
NAMED_UNIT(*)
PLANE_ANGLE_UNIT()
SI_UNIT($,.RADIAN.)
);
#57083=(
NAMED_UNIT(*)
SI_UNIT($,.STERADIAN.)
SOLID_ANGLE_UNIT()
);
#57114=SHAPE_DEFINITION_REPRESENTATION(#57168,#57279);
#57168=PRODUCT_DEFINITION_SHAPE('',$,#57318);
#57279=SHAPE_REPRESENTATION('',(#26507),#57071);
#57287=PRODUCT_DEFINITION_CONTEXT('part definition',#57403,'design');
#57318=PRODUCT_DEFINITION('Linear Guide Slider','Linear Guide Slider',#57356,
#57287);
#57356=PRODUCT_DEFINITION_FORMATION('',$,#57435);
#57403=APPLICATION_CONTEXT(
'Core Data for Automotive Mechanical Design Process');
#57404=PRODUCT_CONTEXT('part definition',#57403,'mechanical');
#57435=PRODUCT('Linear Guide Slider','Linear Guide Slider',$,(#57404));
#57444=PRESENTATION_STYLE_ASSIGNMENT((#57446));
#57446=SURFACE_STYLE_USAGE(.BOTH.,#57448);
#57448=SURFACE_SIDE_STYLE('',(#57450));
#57450=SURFACE_STYLE_FILL_AREA(#57452);
#57452=FILL_AREA_STYLE('Opaque(202,209,238)',(#57454));
#57454=FILL_AREA_STYLE_COLOUR('Opaque(202,209,238)',#57456);
#57456=COLOUR_RGB('Opaque(202,209,238)',0.792156862745098,0.819607843137255,
0.933333333333333);
ENDSEC;
END-ISO-10303-21;
